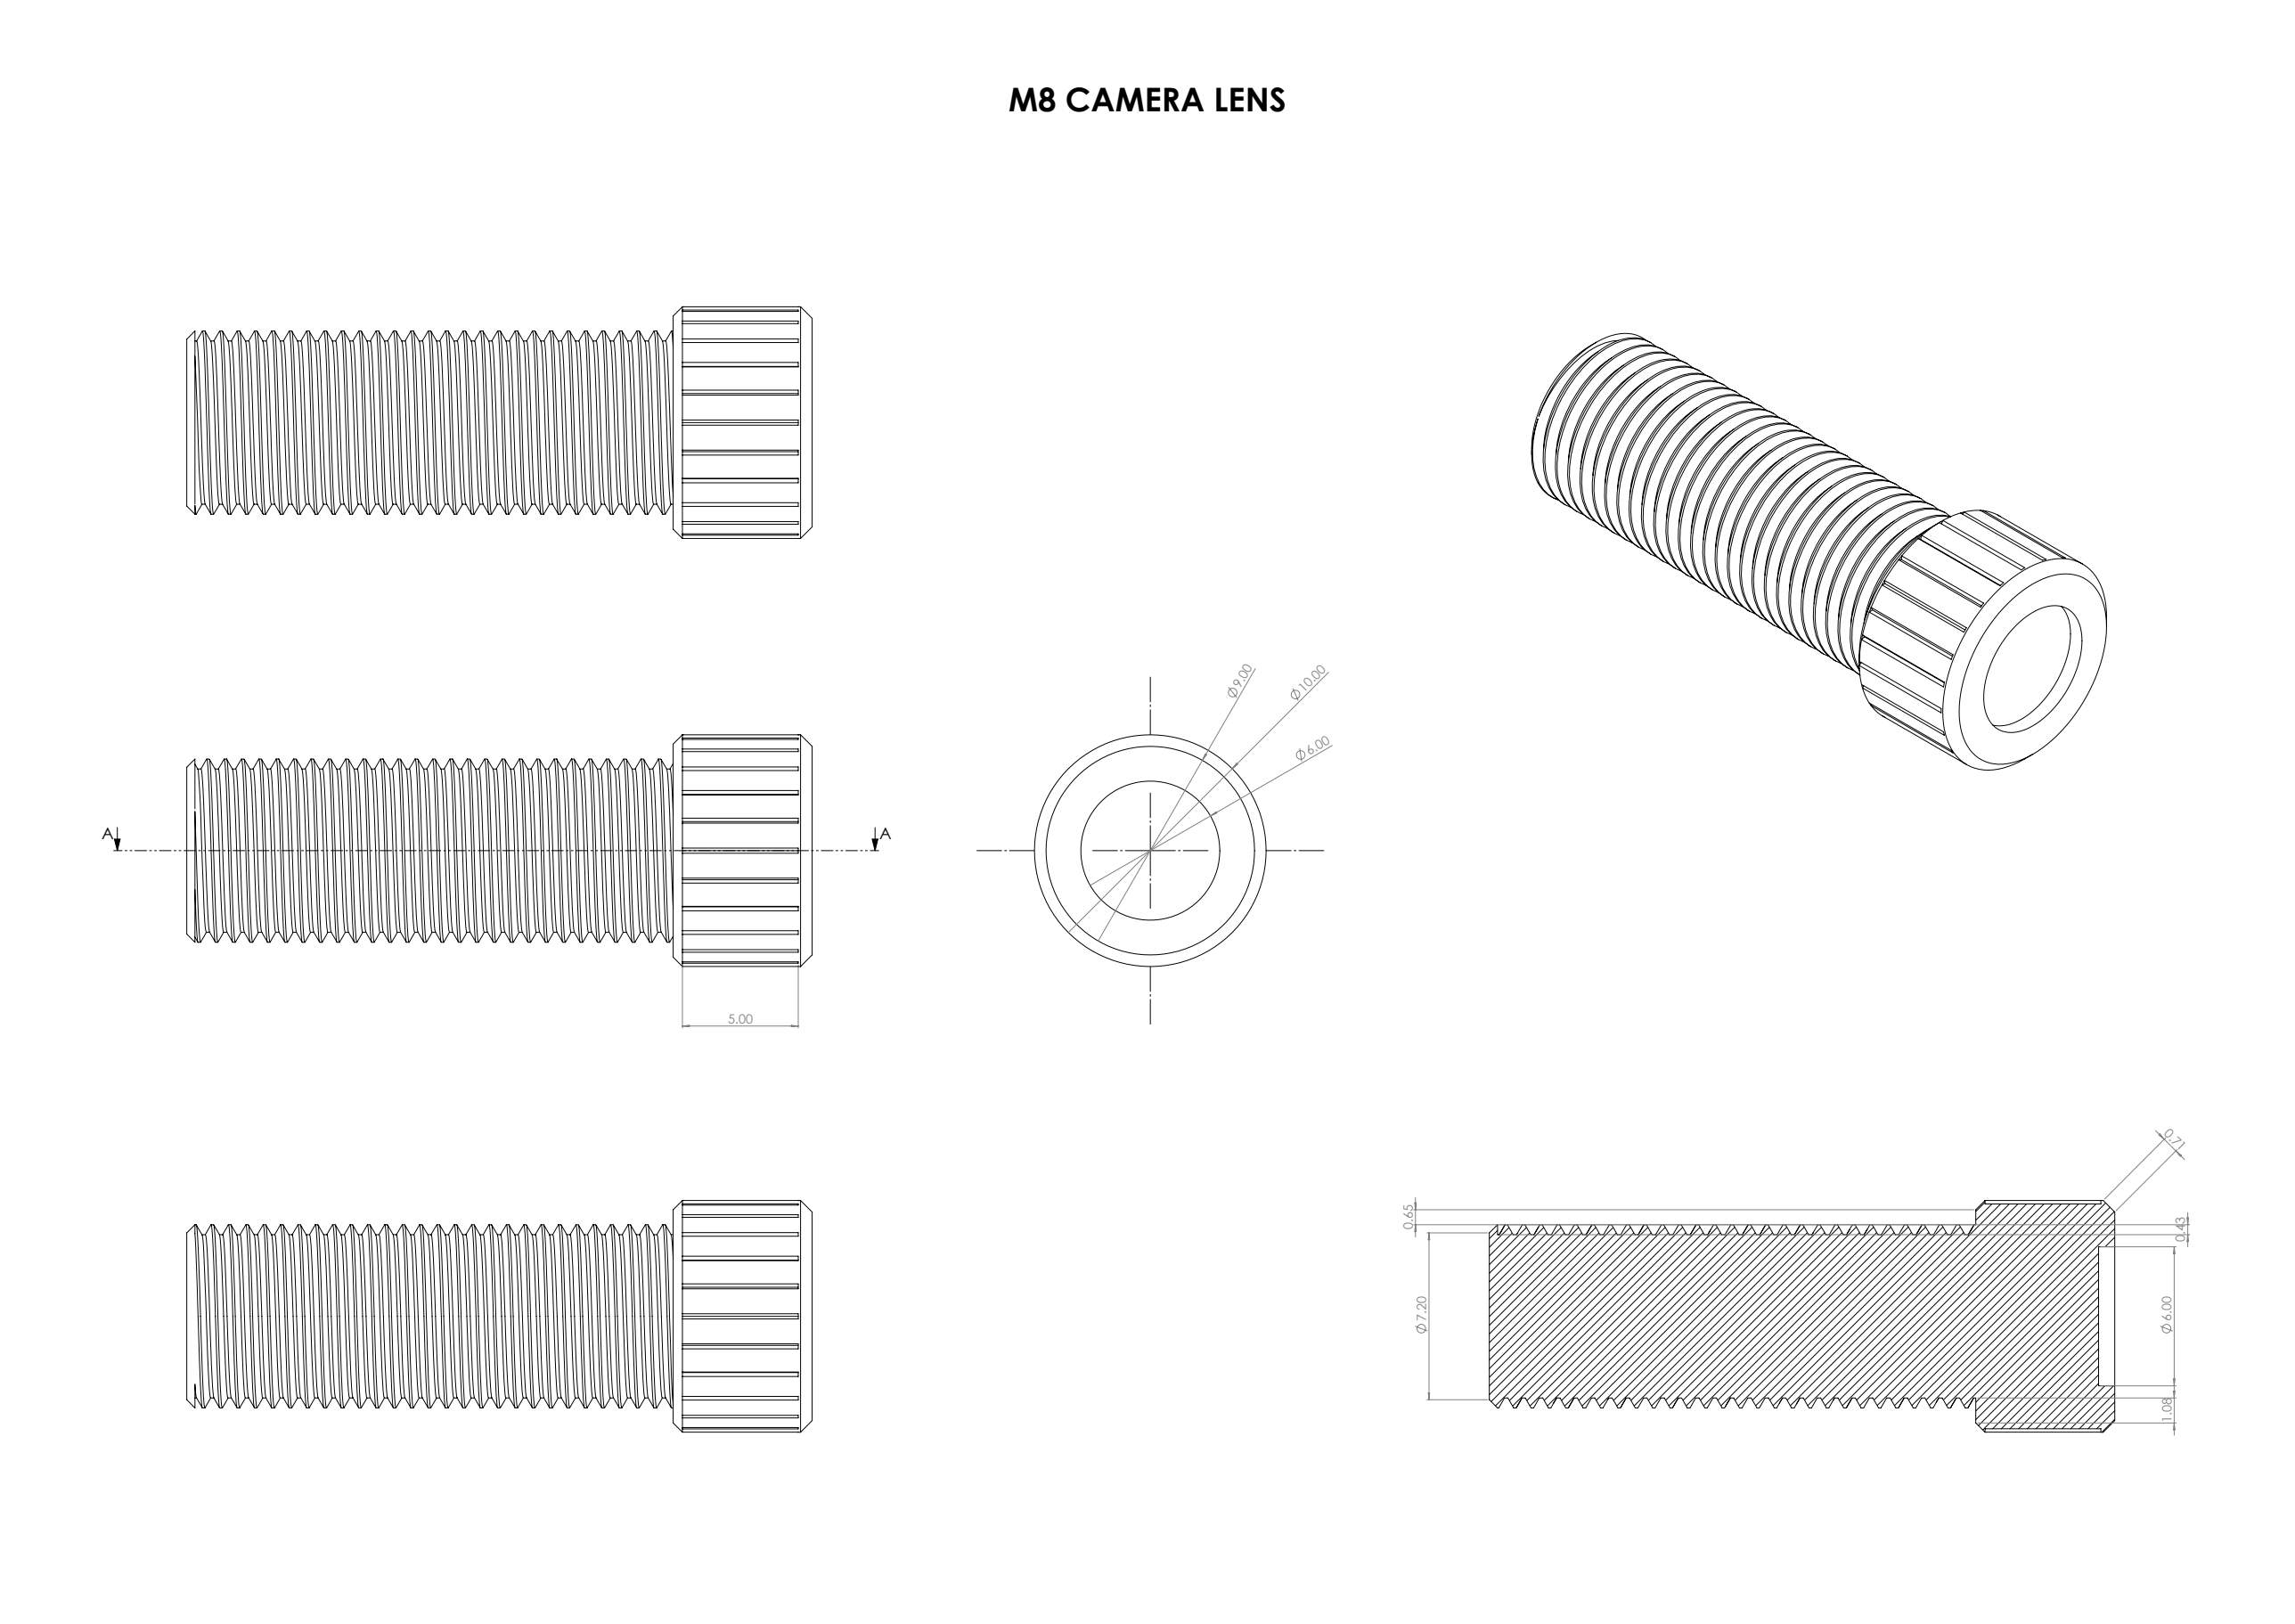
ISO-10303-21;
HEADER;
/* Generated by software containing ST-Developer
 * from STEP Tools, Inc. (www.steptools.com) 
 */

FILE_DESCRIPTION(
/* description */ (''),
/* implementation_level */ '2;1');

FILE_NAME(
/* name */ '07_M8_Camera_Lens.step',
/* time_stamp */ '2026-10-21T02:01:14-07:00',
/* author */ (''),
/* organization */ (''),
/* preprocessor_version */ 'ST-DEVELOPER v20.2',
/* originating_system */ 'Autodesk Translation Framework v15.15.0.0',
/* authorisation */ '');

FILE_SCHEMA (('AUTOMOTIVE_DESIGN { 1 0 10303 214 3 1 1 }'));
ENDSEC;

DATA;
#10=MECHANICAL_DESIGN_GEOMETRIC_PRESENTATION_REPRESENTATION('',(#620),#37181);
#111=B_SPLINE_SURFACE_WITH_KNOTS('',3,3,((#24257,#24258,#24259,#24260,#24261,
#24262,#24263,#24264,#24265,#24266,#24267,#24268,#24269,#24270,#24271,#24272,
#24273,#24274,#24275,#24276,#24277,#24278,#24279,#24280,#24281,#24282,#24283,
#24284,#24285,#24286,#24287,#24288,#24289,#24290,#24291,#24292,#24293,#24294,
#24295,#24296,#24297,#24298,#24299,#24300,#24301,#24302,#24303,#24304,#24305,
#24306,#24307,#24308,#24309,#24310,#24311,#24312,#24313,#24314,#24315,#24316,
#24317,#24318,#24319,#24320,#24321,#24322,#24323,#24324,#24325,#24326,#24327,
#24328,#24329,#24330,#24331,#24332,#24333,#24334,#24335,#24336,#24337,#24338,
#24339,#24340,#24341,#24342,#24343,#24344,#24345,#24346,#24347,#24348,#24349,
#24350,#24351,#24352,#24353,#24354,#24355,#24356,#24357,#24358,#24359,#24360,
#24361,#24362,#24363,#24364,#24365,#24366,#24367,#24368,#24369,#24370,#24371,
#24372,#24373,#24374,#24375,#24376,#24377,#24378,#24379,#24380,#24381,#24382,
#24383,#24384,#24385,#24386,#24387,#24388,#24389,#24390,#24391,#24392,#24393,
#24394,#24395,#24396,#24397,#24398,#24399,#24400,#24401,#24402,#24403,#24404,
#24405,#24406,#24407,#24408,#24409,#24410,#24411,#24412,#24413,#24414,#24415,
#24416,#24417,#24418,#24419,#24420,#24421,#24422,#24423,#24424,#24425,#24426,
#24427,#24428,#24429,#24430,#24431,#24432,#24433,#24434,#24435),(#24436,
#24437,#24438,#24439,#24440,#24441,#24442,#24443,#24444,#24445,#24446,#24447,
#24448,#24449,#24450,#24451,#24452,#24453,#24454,#24455,#24456,#24457,#24458,
#24459,#24460,#24461,#24462,#24463,#24464,#24465,#24466,#24467,#24468,#24469,
#24470,#24471,#24472,#24473,#24474,#24475,#24476,#24477,#24478,#24479,#24480,
#24481,#24482,#24483,#24484,#24485,#24486,#24487,#24488,#24489,#24490,#24491,
#24492,#24493,#24494,#24495,#24496,#24497,#24498,#24499,#24500,#24501,#24502,
#24503,#24504,#24505,#24506,#24507,#24508,#24509,#24510,#24511,#24512,#24513,
#24514,#24515,#24516,#24517,#24518,#24519,#24520,#24521,#24522,#24523,#24524,
#24525,#24526,#24527,#24528,#24529,#24530,#24531,#24532,#24533,#24534,#24535,
#24536,#24537,#24538,#24539,#24540,#24541,#24542,#24543,#24544,#24545,#24546,
#24547,#24548,#24549,#24550,#24551,#24552,#24553,#24554,#24555,#24556,#24557,
#24558,#24559,#24560,#24561,#24562,#24563,#24564,#24565,#24566,#24567,#24568,
#24569,#24570,#24571,#24572,#24573,#24574,#24575,#24576,#24577,#24578,#24579,
#24580,#24581,#24582,#24583,#24584,#24585,#24586,#24587,#24588,#24589,#24590,
#24591,#24592,#24593,#24594,#24595,#24596,#24597,#24598,#24599,#24600,#24601,
#24602,#24603,#24604,#24605,#24606,#24607,#24608,#24609,#24610,#24611,#24612,
#24613,#24614),(#24615,#24616,#24617,#24618,#24619,#24620,#24621,#24622,
#24623,#24624,#24625,#24626,#24627,#24628,#24629,#24630,#24631,#24632,#24633,
#24634,#24635,#24636,#24637,#24638,#24639,#24640,#24641,#24642,#24643,#24644,
#24645,#24646,#24647,#24648,#24649,#24650,#24651,#24652,#24653,#24654,#24655,
#24656,#24657,#24658,#24659,#24660,#24661,#24662,#24663,#24664,#24665,#24666,
#24667,#24668,#24669,#24670,#24671,#24672,#24673,#24674,#24675,#24676,#24677,
#24678,#24679,#24680,#24681,#24682,#24683,#24684,#24685,#24686,#24687,#24688,
#24689,#24690,#24691,#24692,#24693,#24694,#24695,#24696,#24697,#24698,#24699,
#24700,#24701,#24702,#24703,#24704,#24705,#24706,#24707,#24708,#24709,#24710,
#24711,#24712,#24713,#24714,#24715,#24716,#24717,#24718,#24719,#24720,#24721,
#24722,#24723,#24724,#24725,#24726,#24727,#24728,#24729,#24730,#24731,#24732,
#24733,#24734,#24735,#24736,#24737,#24738,#24739,#24740,#24741,#24742,#24743,
#24744,#24745,#24746,#24747,#24748,#24749,#24750,#24751,#24752,#24753,#24754,
#24755,#24756,#24757,#24758,#24759,#24760,#24761,#24762,#24763,#24764,#24765,
#24766,#24767,#24768,#24769,#24770,#24771,#24772,#24773,#24774,#24775,#24776,
#24777,#24778,#24779,#24780,#24781,#24782,#24783,#24784,#24785,#24786,#24787,
#24788,#24789,#24790,#24791,#24792,#24793),(#24794,#24795,#24796,#24797,
#24798,#24799,#24800,#24801,#24802,#24803,#24804,#24805,#24806,#24807,#24808,
#24809,#24810,#24811,#24812,#24813,#24814,#24815,#24816,#24817,#24818,#24819,
#24820,#24821,#24822,#24823,#24824,#24825,#24826,#24827,#24828,#24829,#24830,
#24831,#24832,#24833,#24834,#24835,#24836,#24837,#24838,#24839,#24840,#24841,
#24842,#24843,#24844,#24845,#24846,#24847,#24848,#24849,#24850,#24851,#24852,
#24853,#24854,#24855,#24856,#24857,#24858,#24859,#24860,#24861,#24862,#24863,
#24864,#24865,#24866,#24867,#24868,#24869,#24870,#24871,#24872,#24873,#24874,
#24875,#24876,#24877,#24878,#24879,#24880,#24881,#24882,#24883,#24884,#24885,
#24886,#24887,#24888,#24889,#24890,#24891,#24892,#24893,#24894,#24895,#24896,
#24897,#24898,#24899,#24900,#24901,#24902,#24903,#24904,#24905,#24906,#24907,
#24908,#24909,#24910,#24911,#24912,#24913,#24914,#24915,#24916,#24917,#24918,
#24919,#24920,#24921,#24922,#24923,#24924,#24925,#24926,#24927,#24928,#24929,
#24930,#24931,#24932,#24933,#24934,#24935,#24936,#24937,#24938,#24939,#24940,
#24941,#24942,#24943,#24944,#24945,#24946,#24947,#24948,#24949,#24950,#24951,
#24952,#24953,#24954,#24955,#24956,#24957,#24958,#24959,#24960,#24961,#24962,
#24963,#24964,#24965,#24966,#24967,#24968,#24969,#24970,#24971,#24972)),
 .UNSPECIFIED.,.F.,.F.,.F.,(4,4),(4,1,1,1,1,1,1,1,1,1,1,1,1,1,1,1,1,1,1,
1,1,1,1,1,1,1,1,1,1,1,1,1,1,1,1,1,1,1,1,1,1,1,1,1,1,1,1,1,1,1,1,1,1,1,1,
1,1,1,1,1,1,1,1,1,1,1,1,1,1,1,1,1,1,1,1,1,1,1,1,1,1,1,1,1,1,1,1,1,1,1,1,
1,1,1,1,1,1,1,1,1,1,1,1,1,1,1,1,1,1,1,1,1,1,1,1,1,1,1,1,1,1,1,1,1,1,1,1,
1,1,1,1,1,1,1,1,1,1,1,1,1,1,1,1,1,1,1,1,1,1,1,1,1,1,1,1,1,1,1,1,1,1,1,1,
1,1,1,1,1,1,1,1,1,1,1,1,1,4),(0.,0.0496809906637673),(8.29514371672438,
9.2897150667619,10.2842864167994,11.2788577668369,12.2734291168745,13.268000466912,
14.2625718169495,15.257143166987,16.2517145170246,17.2462858670621,18.2408572170996,
19.2354285671371,20.2299999171747,21.2245712672122,22.2191426172497,23.2137139672872,
24.2082853173248,25.2028566673623,26.1974280173998,27.1919993674374,28.1865707174749,
29.1811420675124,30.1757134175499,31.1702847675875,32.164856117625,33.1594274676625,
34.1539988177,35.1485701677375,36.1431415177751,37.1377128678126,38.1322842178501,
39.1268555678876,40.1214269179252,41.1159982679627,42.1105696180002,43.1051409680378,
44.0997123180753,45.0942836681128,46.0888550181503,47.0834263681879,48.0779977182254,
49.0725690682629,50.0671404183004,51.061711768338,52.0562831183755,53.050854468413,
54.0454258184505,55.039997168488,56.0345685185256,57.0291398685631,58.0237112186006,
59.0182825686381,60.0128539186757,61.0074252687132,62.0019966187507,62.9965679687882,
63.9911393188258,64.9857106688633,65.9802820189008,66.9748533689383,67.9694247189759,
68.9639960690134,69.9585674190509,70.9531387690884,71.947710119126,72.9422814691635,
73.936852819201,74.9314241692385,75.9259955192761,76.9205668693136,77.9151382193511,
78.9097095693886,79.9042809194262,80.8988522694637,81.8934236195012,82.8879949695387,
83.8825663195763,84.8771376696138,85.8717090196513,86.8662803696888,87.8608517197264,
88.8554230697639,89.8499944198014,90.8445657698389,91.8391371198765,92.833708469914,
93.8282798199515,94.822851169989,95.8174225200266,96.8119938700641,97.8065652201016,
98.8011365701391,99.7957079201767,100.790279270214,101.784850620252,102.779421970289,
103.773993320327,104.768564670364,105.763136020402,106.757707370439,107.752278720477,
108.746850070514,109.741421420552,110.735992770589,111.730564120627,112.725135470664,
113.719706820702,114.71427817074,115.708849520777,116.703420870815,117.697992220852,
118.69256357089,119.687134920927,120.681706270965,121.676277621002,122.67084897104,
123.665420321077,124.659991671115,125.654563021152,126.64913437119,127.643705721227,
128.638277071265,129.632848421302,130.62741977134,131.621991121377,132.616562471415,
133.611133821453,134.60570517149,135.600276521528,136.594847871565,137.589419221603,
138.58399057164,139.578561921678,140.573133271715,141.567704621753,142.56227597179,
143.556847321828,144.551418671865,145.545990021903,146.54056137194,147.535132721978,
148.529704072015,149.524275422053,150.51884677209,151.513418122128,152.507989472165,
153.502560822203,154.497132172241,155.491703522278,156.486274872316,157.480846222353,
158.475417572391,159.469988922428,160.464560272466,161.459131622503,162.453702972541,
163.448274322578,164.442845672616,165.437417022653,166.431988372691,167.426559722728,
168.421131072766,169.415702422803,170.410273772841,171.404845122878,172.399416472916,
173.393987822954,174.388559172991,175.383130523029,176.377701873066,177.372273223104,
178.366844573141,179.361415923179,180.355987273216,181.350558623254,182.345129973291,
183.339701323329),.UNSPECIFIED.);
#112=B_SPLINE_SURFACE_WITH_KNOTS('',3,3,((#25202,#25203,#25204,#25205,#25206,
#25207,#25208,#25209,#25210,#25211,#25212,#25213,#25214,#25215,#25216,#25217,
#25218,#25219,#25220,#25221,#25222,#25223,#25224,#25225,#25226,#25227,#25228,
#25229,#25230,#25231,#25232,#25233,#25234,#25235,#25236,#25237,#25238,#25239,
#25240,#25241,#25242,#25243,#25244,#25245,#25246,#25247,#25248,#25249,#25250,
#25251,#25252,#25253,#25254,#25255,#25256,#25257,#25258,#25259,#25260,#25261,
#25262,#25263,#25264,#25265,#25266,#25267,#25268,#25269,#25270,#25271,#25272,
#25273,#25274,#25275,#25276,#25277,#25278,#25279,#25280,#25281,#25282,#25283,
#25284,#25285,#25286,#25287,#25288,#25289,#25290,#25291,#25292,#25293,#25294,
#25295,#25296,#25297,#25298,#25299,#25300,#25301,#25302,#25303,#25304,#25305,
#25306,#25307,#25308,#25309,#25310,#25311,#25312,#25313,#25314,#25315,#25316,
#25317,#25318,#25319,#25320,#25321,#25322,#25323,#25324,#25325,#25326,#25327,
#25328,#25329,#25330,#25331,#25332,#25333,#25334,#25335,#25336,#25337,#25338,
#25339,#25340,#25341,#25342,#25343,#25344,#25345,#25346,#25347,#25348,#25349,
#25350,#25351,#25352,#25353,#25354,#25355,#25356,#25357,#25358,#25359,#25360,
#25361,#25362,#25363,#25364,#25365,#25366,#25367,#25368,#25369,#25370,#25371,
#25372,#25373,#25374,#25375,#25376,#25377,#25378,#25379,#25380),(#25381,
#25382,#25383,#25384,#25385,#25386,#25387,#25388,#25389,#25390,#25391,#25392,
#25393,#25394,#25395,#25396,#25397,#25398,#25399,#25400,#25401,#25402,#25403,
#25404,#25405,#25406,#25407,#25408,#25409,#25410,#25411,#25412,#25413,#25414,
#25415,#25416,#25417,#25418,#25419,#25420,#25421,#25422,#25423,#25424,#25425,
#25426,#25427,#25428,#25429,#25430,#25431,#25432,#25433,#25434,#25435,#25436,
#25437,#25438,#25439,#25440,#25441,#25442,#25443,#25444,#25445,#25446,#25447,
#25448,#25449,#25450,#25451,#25452,#25453,#25454,#25455,#25456,#25457,#25458,
#25459,#25460,#25461,#25462,#25463,#25464,#25465,#25466,#25467,#25468,#25469,
#25470,#25471,#25472,#25473,#25474,#25475,#25476,#25477,#25478,#25479,#25480,
#25481,#25482,#25483,#25484,#25485,#25486,#25487,#25488,#25489,#25490,#25491,
#25492,#25493,#25494,#25495,#25496,#25497,#25498,#25499,#25500,#25501,#25502,
#25503,#25504,#25505,#25506,#25507,#25508,#25509,#25510,#25511,#25512,#25513,
#25514,#25515,#25516,#25517,#25518,#25519,#25520,#25521,#25522,#25523,#25524,
#25525,#25526,#25527,#25528,#25529,#25530,#25531,#25532,#25533,#25534,#25535,
#25536,#25537,#25538,#25539,#25540,#25541,#25542,#25543,#25544,#25545,#25546,
#25547,#25548,#25549,#25550,#25551,#25552,#25553,#25554,#25555,#25556,#25557,
#25558,#25559),(#25560,#25561,#25562,#25563,#25564,#25565,#25566,#25567,
#25568,#25569,#25570,#25571,#25572,#25573,#25574,#25575,#25576,#25577,#25578,
#25579,#25580,#25581,#25582,#25583,#25584,#25585,#25586,#25587,#25588,#25589,
#25590,#25591,#25592,#25593,#25594,#25595,#25596,#25597,#25598,#25599,#25600,
#25601,#25602,#25603,#25604,#25605,#25606,#25607,#25608,#25609,#25610,#25611,
#25612,#25613,#25614,#25615,#25616,#25617,#25618,#25619,#25620,#25621,#25622,
#25623,#25624,#25625,#25626,#25627,#25628,#25629,#25630,#25631,#25632,#25633,
#25634,#25635,#25636,#25637,#25638,#25639,#25640,#25641,#25642,#25643,#25644,
#25645,#25646,#25647,#25648,#25649,#25650,#25651,#25652,#25653,#25654,#25655,
#25656,#25657,#25658,#25659,#25660,#25661,#25662,#25663,#25664,#25665,#25666,
#25667,#25668,#25669,#25670,#25671,#25672,#25673,#25674,#25675,#25676,#25677,
#25678,#25679,#25680,#25681,#25682,#25683,#25684,#25685,#25686,#25687,#25688,
#25689,#25690,#25691,#25692,#25693,#25694,#25695,#25696,#25697,#25698,#25699,
#25700,#25701,#25702,#25703,#25704,#25705,#25706,#25707,#25708,#25709,#25710,
#25711,#25712,#25713,#25714,#25715,#25716,#25717,#25718,#25719,#25720,#25721,
#25722,#25723,#25724,#25725,#25726,#25727,#25728,#25729,#25730,#25731,#25732,
#25733,#25734,#25735,#25736,#25737,#25738),(#25739,#25740,#25741,#25742,
#25743,#25744,#25745,#25746,#25747,#25748,#25749,#25750,#25751,#25752,#25753,
#25754,#25755,#25756,#25757,#25758,#25759,#25760,#25761,#25762,#25763,#25764,
#25765,#25766,#25767,#25768,#25769,#25770,#25771,#25772,#25773,#25774,#25775,
#25776,#25777,#25778,#25779,#25780,#25781,#25782,#25783,#25784,#25785,#25786,
#25787,#25788,#25789,#25790,#25791,#25792,#25793,#25794,#25795,#25796,#25797,
#25798,#25799,#25800,#25801,#25802,#25803,#25804,#25805,#25806,#25807,#25808,
#25809,#25810,#25811,#25812,#25813,#25814,#25815,#25816,#25817,#25818,#25819,
#25820,#25821,#25822,#25823,#25824,#25825,#25826,#25827,#25828,#25829,#25830,
#25831,#25832,#25833,#25834,#25835,#25836,#25837,#25838,#25839,#25840,#25841,
#25842,#25843,#25844,#25845,#25846,#25847,#25848,#25849,#25850,#25851,#25852,
#25853,#25854,#25855,#25856,#25857,#25858,#25859,#25860,#25861,#25862,#25863,
#25864,#25865,#25866,#25867,#25868,#25869,#25870,#25871,#25872,#25873,#25874,
#25875,#25876,#25877,#25878,#25879,#25880,#25881,#25882,#25883,#25884,#25885,
#25886,#25887,#25888,#25889,#25890,#25891,#25892,#25893,#25894,#25895,#25896,
#25897,#25898,#25899,#25900,#25901,#25902,#25903,#25904,#25905,#25906,#25907,
#25908,#25909,#25910,#25911,#25912,#25913,#25914,#25915,#25916,#25917)),
 .UNSPECIFIED.,.F.,.F.,.F.,(4,4),(4,1,1,1,1,1,1,1,1,1,1,1,1,1,1,1,1,1,1,
1,1,1,1,1,1,1,1,1,1,1,1,1,1,1,1,1,1,1,1,1,1,1,1,1,1,1,1,1,1,1,1,1,1,1,1,
1,1,1,1,1,1,1,1,1,1,1,1,1,1,1,1,1,1,1,1,1,1,1,1,1,1,1,1,1,1,1,1,1,1,1,1,
1,1,1,1,1,1,1,1,1,1,1,1,1,1,1,1,1,1,1,1,1,1,1,1,1,1,1,1,1,1,1,1,1,1,1,1,
1,1,1,1,1,1,1,1,1,1,1,1,1,1,1,1,1,1,1,1,1,1,1,1,1,1,1,1,1,1,1,1,1,1,1,1,
1,1,1,1,1,1,1,1,1,1,1,1,1,4),(0.,0.0496809906637673),(11.6149723878396,
12.6095437378771,13.6041150879146,14.5986864379522,15.5932577879897,16.5878291380272,
17.5824004880647,18.5769718381023,19.5715431881398,20.5661145381773,21.5606858882148,
22.5552572382524,23.5498285882899,24.5443999383274,25.5389712883649,26.5335426384025,
27.52811398844,28.5226853384775,29.517256688515,30.5118280385526,31.5063993885901,
32.5009707386276,33.4955420886651,34.4901134387027,35.4846847887402,36.4792561387777,
37.4738274888152,38.4683988388528,39.4629701888903,40.4575415389278,41.4521128889653,
42.4466842390029,43.4412555890404,44.4358269390779,45.4303982891154,46.424969639153,
47.4195409891905,48.414112339228,49.4086836892655,50.4032550393031,51.3978263893406,
52.3923977393781,53.3869690894156,54.3815404394532,55.3761117894907,56.3706831395282,
57.3652544895657,58.3598258396033,59.3543971896408,60.3489685396783,61.3435398897158,
62.3381112397534,63.3326825897909,64.3272539398284,65.3218252898659,66.3163966399035,
67.310967989941,68.3055393399785,69.300110690016,70.2946820400536,71.2892533900911,
72.2838247401286,73.2783960901661,74.2729674402037,75.2675387902412,76.2621101402787,
77.2566814903162,78.2512528403538,79.2458241903913,80.2403955404288,81.2349668904663,
82.2295382405039,83.2241095905414,84.2186809405789,85.2132522906164,86.207823640654,
87.2023949906915,88.196966340729,89.1915376907665,90.1861090408041,91.1806803908416,
92.1752517408791,93.1698230909166,94.1643944409542,95.1589657909917,96.1535371410292,
97.1481084910667,98.1426798411043,99.1372511911418,100.131822541179,101.126393891217,
102.120965241254,103.115536591292,104.110107941329,105.104679291367,106.099250641404,
107.093821991442,108.08839334148,109.082964691517,110.077536041555,111.072107391592,
112.06667874163,113.061250091667,114.055821441705,115.050392791742,116.04496414178,
117.039535491817,118.034106841855,119.028678191892,120.02324954193,121.017820891967,
122.012392242005,123.006963592042,124.00153494208,124.996106292117,125.990677642155,
126.985248992192,127.97982034223,128.974391692268,129.968963042305,130.963534392343,
131.95810574238,132.952677092418,133.947248442455,134.941819792493,135.93639114253,
136.930962492568,137.925533842605,138.920105192643,139.91467654268,140.909247892718,
141.903819242755,142.898390592793,143.89296194283,144.887533292868,145.882104642905,
146.876675992943,147.87124734298,148.865818693018,149.860390043056,150.854961393093,
151.849532743131,152.844104093168,153.838675443206,154.833246793243,155.827818143281,
156.822389493318,157.816960843356,158.811532193393,159.806103543431,160.800674893468,
161.795246243506,162.789817593543,163.784388943581,164.778960293618,165.773531643656,
166.768102993693,167.762674343731,168.757245693769,169.751817043806,170.746388393844,
171.740959743881,172.735531093919,173.730102443956,174.724673793994,175.719245144031,
176.713816494069,177.708387844106,178.702959194144,179.697530544181,180.692101894219,
181.686673244256,182.681244594294,183.675815944331,184.670387294369,185.664958644406,
186.659529994444),.UNSPECIFIED.);
#141=B_SPLINE_CURVE_WITH_KNOTS('',3,(#21804,#21805,#21806,#21807,#21808,
#21809,#21810,#21811,#21812,#21813),.UNSPECIFIED.,.F.,.F.,(4,3,3,4),(-4.09299088010945,
-3.9782854001501,-2.98371405011257,-2.08103247056473),.UNSPECIFIED.);
#142=B_SPLINE_CURVE_WITH_KNOTS('',3,(#21816,#21817,#21818,#21819,#21820,
#21821,#21822),.UNSPECIFIED.,.F.,.F.,(4,3,4),(0.,0.994571350037526,1.12963424404512),
 .UNSPECIFIED.);
#143=B_SPLINE_CURVE_WITH_KNOTS('',3,(#21827,#21828,#21829,#21830,#21831,
#21832,#21833,#21834,#21835,#21836,#21837,#21838,#21839,#21840,#21841,#21842,
#21843,#21844,#21845,#21846,#21847,#21848),.UNSPECIFIED.,.F.,.F.,(4,3,3,
3,3,3,3,4),(-10.376176187289,-9.94571350037525,-8.95114215033773,-7.9565708003002,
-6.96199945026268,-5.96742810022515,-4.97285675018763,-4.09299088010945),
 .UNSPECIFIED.);
#144=B_SPLINE_CURVE_WITH_KNOTS('',3,(#21849,#21850,#21851,#21852,#21853,
#21854,#21855,#21856,#21857,#21858,#21859,#21860,#21861,#21862,#21863,#21864,
#21865,#21866,#21867,#21868,#21869,#21870),.UNSPECIFIED.,.F.,.F.,(4,3,3,
3,3,3,3,4),(1.12963424404512,1.98914270007505,2.98371405011257,3.9782854001501,
4.97285675018762,5.96742810022515,6.96199945026267,7.4128195512247),
 .UNSPECIFIED.);
#145=B_SPLINE_CURVE_WITH_KNOTS('',3,(#21875,#21876,#21877,#21878,#21879,
#21880,#21881,#21882,#21883,#21884,#21885,#21886,#21887,#21888,#21889,#21890,
#21891,#21892,#21893,#21894,#21895,#21896),.UNSPECIFIED.,.F.,.F.,(4,3,3,
3,3,3,3,4),(-16.6593614944686,-15.9131416006004,-14.9185702505629,-13.9239989005253,
-12.9294275504878,-11.9348562004503,-10.9402848504128,-10.376176187289),
 .UNSPECIFIED.);
#146=B_SPLINE_CURVE_WITH_KNOTS('',3,(#21897,#21898,#21899,#21900,#21901,
#21902,#21903,#21904,#21905,#21906,#21907,#21908,#21909,#21910,#21911,#21912,
#21913,#21914,#21915,#21916,#21917,#21918),.UNSPECIFIED.,.F.,.F.,(4,3,3,
3,3,3,3,4),(7.4128195512247,7.9565708003002,8.95114215033773,9.94571350037526,
10.9402848504128,11.9348562004503,12.9294275504878,13.6960048584043),
 .UNSPECIFIED.);
#147=B_SPLINE_CURVE_WITH_KNOTS('',3,(#21923,#21924,#21925,#21926,#21927,
#21928,#21929,#21930,#21931,#21932,#21933,#21934,#21935,#21936,#21937,#21938,
#21939,#21940,#21941,#21942,#21943,#21944,#21945,#21946,#21947),
 .UNSPECIFIED.,.F.,.F.,(4,3,3,3,3,3,3,3,4),(-22.9425468016482,-22.8751410508631,
-21.8805697008255,-20.885998350788,-19.8914270007505,-18.896855650713,-17.9022843006754,
-16.9077129506379,-16.6593614944686),.UNSPECIFIED.);
#148=B_SPLINE_CURVE_WITH_KNOTS('',3,(#21948,#21949,#21950,#21951,#21952,
#21953,#21954,#21955,#21956,#21957,#21958,#21959,#21960,#21961,#21962,#21963,
#21964,#21965,#21966,#21967,#21968,#21969,#21970,#21971,#21972),
 .UNSPECIFIED.,.F.,.F.,(4,3,3,3,3,3,3,3,4),(13.6960048584043,13.9239989005254,
14.9185702505629,15.9131416006004,16.9077129506379,17.9022843006755,18.896855650713,
19.8914270007505,19.9791901655839),.UNSPECIFIED.);
#149=B_SPLINE_CURVE_WITH_KNOTS('',3,(#21977,#21978,#21979,#21980,#21981,
#21982,#21983,#21984,#21985,#21986,#21987,#21988,#21989,#21990,#21991,#21992,
#21993,#21994,#21995,#21996,#21997,#21998),.UNSPECIFIED.,.F.,.F.,(4,3,3,
3,3,3,3,4),(-29.2257321088278,-28.8425691510882,-27.8479978010507,-26.8534264510132,
-25.8588551009757,-24.8642837509381,-23.8697124009006,-22.9425468016482),
 .UNSPECIFIED.);
#150=B_SPLINE_CURVE_WITH_KNOTS('',3,(#21999,#22000,#22001,#22002,#22003,
#22004,#22005,#22006,#22007,#22008,#22009,#22010,#22011,#22012,#22013,#22014,
#22015,#22016,#22017,#22018,#22019,#22020),.UNSPECIFIED.,.F.,.F.,(4,3,3,
3,3,3,3,4),(19.9791901655839,20.885998350788,21.8805697008255,22.8751410508631,
23.8697124009006,24.8642837509381,25.8588551009756,26.2623754727635),
 .UNSPECIFIED.);
#151=B_SPLINE_CURVE_WITH_KNOTS('',3,(#22025,#22026,#22027,#22028,#22029,
#22030,#22031,#22032,#22033,#22034,#22035,#22036,#22037,#22038,#22039,#22040,
#22041,#22042,#22043,#22044,#22045,#22046),.UNSPECIFIED.,.F.,.F.,(4,3,3,
3,3,3,3,4),(-35.5089174160074,-34.8099972513134,-33.8154259012759,-32.8208545512383,
-31.8262832012008,-30.8317118511633,-29.8371405011258,-29.2257321088278),
 .UNSPECIFIED.);
#152=B_SPLINE_CURVE_WITH_KNOTS('',3,(#22047,#22048,#22049,#22050,#22051,
#22052,#22053,#22054,#22055,#22056,#22057,#22058,#22059,#22060,#22061,#22062,
#22063,#22064,#22065,#22066,#22067,#22068),.UNSPECIFIED.,.F.,.F.,(4,3,3,
3,3,3,3,4),(26.2623754727635,26.8534264510132,27.8479978010507,28.8425691510882,
29.8371405011258,30.8317118511633,31.8262832012008,32.545560779943),
 .UNSPECIFIED.);
#153=B_SPLINE_CURVE_WITH_KNOTS('',3,(#22073,#22074,#22075,#22076,#22077,
#22078,#22079,#22080,#22081,#22082,#22083,#22084,#22085,#22086,#22087,#22088,
#22089,#22090,#22091,#22092,#22093,#22094,#22095,#22096,#22097),
 .UNSPECIFIED.,.F.,.F.,(4,3,3,3,3,3,3,3,4),(-41.792102723187,-41.771996701576,
-40.7774253515385,-39.782854001501,-38.7882826514635,-37.7937113014259,
-36.7991399513884,-35.8045686013509,-35.5089174160074),.UNSPECIFIED.);
#154=B_SPLINE_CURVE_WITH_KNOTS('',3,(#22098,#22099,#22100,#22101,#22102,
#22103,#22104,#22105,#22106,#22107,#22108,#22109,#22110,#22111,#22112,#22113,
#22114,#22115,#22116,#22117,#22118,#22119,#22120,#22121,#22122),
 .UNSPECIFIED.,.F.,.F.,(4,3,3,3,3,3,3,3,4),(32.545560779943,32.8208545512383,
33.8154259012759,34.8099972513134,35.8045686013509,36.7991399513884,37.7937113014259,
38.7882826514634,38.8287460871226),.UNSPECIFIED.);
#155=B_SPLINE_CURVE_WITH_KNOTS('',3,(#22127,#22128,#22129,#22130,#22131,
#22132,#22133,#22134,#22135,#22136,#22137,#22138,#22139,#22140,#22141,#22142,
#22143,#22144,#22145,#22146,#22147,#22148),.UNSPECIFIED.,.F.,.F.,(4,3,3,
3,3,3,3,4),(-48.0752880303666,-47.7394248018012,-46.7448534517637,-45.7502821017261,
-44.7557107516886,-43.7611394016511,-42.7665680516136,-41.792102723187),
 .UNSPECIFIED.);
#156=B_SPLINE_CURVE_WITH_KNOTS('',3,(#22149,#22150,#22151,#22152,#22153,
#22154,#22155,#22156,#22157,#22158,#22159,#22160,#22161,#22162,#22163,#22164,
#22165,#22166,#22167,#22168,#22169,#22170),.UNSPECIFIED.,.F.,.F.,(4,3,3,
3,3,3,3,4),(38.8287460871226,39.782854001501,40.7774253515385,41.771996701576,
42.7665680516136,43.7611394016511,44.7557107516886,45.1119313943022),
 .UNSPECIFIED.);
#157=B_SPLINE_CURVE_WITH_KNOTS('',3,(#22175,#22176,#22177,#22178,#22179,
#22180,#22181,#22182,#22183,#22184,#22185,#22186,#22187,#22188,#22189,#22190,
#22191,#22192,#22193,#22194,#22195,#22196),.UNSPECIFIED.,.F.,.F.,(4,3,3,
3,3,3,3,4),(-54.3584733375462,-53.7068529020263,-52.7122815519888,-51.7177102019513,
-50.7231388519138,-49.7285675018762,-48.7339961518387,-48.0752880303666),
 .UNSPECIFIED.);
#158=B_SPLINE_CURVE_WITH_KNOTS('',3,(#22197,#22198,#22199,#22200,#22201,
#22202,#22203,#22204,#22205,#22206,#22207,#22208,#22209,#22210,#22211,#22212,
#22213,#22214,#22215,#22216,#22217,#22218),.UNSPECIFIED.,.F.,.F.,(4,3,3,
3,3,3,3,4),(45.1119313943022,45.7502821017262,46.7448534517637,47.7394248018012,
48.7339961518387,49.7285675018763,50.7231388519138,51.3951167014818),
 .UNSPECIFIED.);
#159=B_SPLINE_CURVE_WITH_KNOTS('',3,(#22223,#22224,#22225,#22226,#22227,
#22228,#22229,#22230,#22231,#22232,#22233,#22234,#22235,#22236,#22237,#22238,
#22239,#22240,#22241,#22242,#22243,#22244),.UNSPECIFIED.,.F.,.F.,(4,3,3,
3,3,3,3,4),(-60.6416586447258,-59.6742810022515,-58.679709652214,-57.6851383021764,
-56.6905669521389,-55.6959956021014,-54.7014242520639,-54.3584733375462),
 .UNSPECIFIED.);
#160=B_SPLINE_CURVE_WITH_KNOTS('',3,(#22245,#22246,#22247,#22248,#22249,
#22250,#22251,#22252,#22253,#22254,#22255,#22256,#22257,#22258,#22259,#22260,
#22261,#22262,#22263,#22264,#22265,#22266),.UNSPECIFIED.,.F.,.F.,(4,3,3,
3,3,3,3,4),(51.3951167014818,51.7177102019513,52.7122815519888,53.7068529020263,
54.7014242520639,55.6959956021014,56.6905669521389,57.6783020086614),
 .UNSPECIFIED.);
#161=B_SPLINE_CURVE_WITH_KNOTS('',3,(#22271,#22272,#22273,#22274,#22275,
#22276,#22277,#22278,#22279,#22280,#22281,#22282,#22283,#22284,#22285,#22286,
#22287,#22288,#22289,#22290,#22291,#22292,#22293,#22294,#22295),
 .UNSPECIFIED.,.F.,.F.,(4,3,3,3,3,3,3,3,4),(-66.9248439519054,-66.6362804525142,
-65.6417091024766,-64.6471377524391,-63.6525664024016,-62.6579950523641,
-61.6634237023265,-60.668852352289,-60.6416586447258),.UNSPECIFIED.);
#162=B_SPLINE_CURVE_WITH_KNOTS('',3,(#22296,#22297,#22298,#22299,#22300,
#22301,#22302,#22303,#22304,#22305,#22306,#22307,#22308,#22309,#22310,#22311,
#22312,#22313,#22314,#22315,#22316,#22317,#22318,#22319,#22320),
 .UNSPECIFIED.,.F.,.F.,(4,3,3,3,3,3,3,3,4),(57.6783020086614,57.6851383021765,
58.679709652214,59.6742810022515,60.668852352289,61.6634237023265,62.6579950523641,
63.6525664024016,63.961487315841),.UNSPECIFIED.);
#163=B_SPLINE_CURVE_WITH_KNOTS('',3,(#22325,#22326,#22327,#22328,#22329,
#22330,#22331,#22332,#22333,#22334,#22335,#22336,#22337,#22338,#22339,#22340,
#22341,#22342,#22343,#22344,#22345,#22346),.UNSPECIFIED.,.F.,.F.,(4,3,3,
3,3,3,3,4),(-73.2080292590849,-72.6037085527393,-71.6091372027018,-70.6145658526643,
-69.6199945026267,-68.6254231525892,-67.6308518025517,-66.9248439519054),
 .UNSPECIFIED.);
#164=B_SPLINE_CURVE_WITH_KNOTS('',3,(#22347,#22348,#22349,#22350,#22351,
#22352,#22353,#22354,#22355,#22356,#22357,#22358,#22359,#22360,#22361,#22362,
#22363,#22364,#22365,#22366,#22367,#22368),.UNSPECIFIED.,.F.,.F.,(4,3,3,
3,3,3,3,4),(63.961487315841,64.6471377524391,65.6417091024766,66.6362804525142,
67.6308518025517,68.6254231525892,69.6199945026268,70.2446726230206),
 .UNSPECIFIED.);
#165=B_SPLINE_CURVE_WITH_KNOTS('',3,(#22373,#22374,#22375,#22376,#22377,
#22378,#22379,#22380,#22381,#22382,#22383,#22384,#22385,#22386,#22387,#22388,
#22389,#22390,#22391,#22392,#22393,#22394),.UNSPECIFIED.,.F.,.F.,(4,3,3,
3,3,3,3,4),(-79.4912145662645,-78.5711366529645,-77.5765653029269,-76.5819939528894,
-75.5874226028519,-74.5928512528144,-73.5982799027768,-73.2080292590849),
 .UNSPECIFIED.);
#166=B_SPLINE_CURVE_WITH_KNOTS('',3,(#22395,#22396,#22397,#22398,#22399,
#22400,#22401,#22402,#22403,#22404,#22405,#22406,#22407,#22408,#22409,#22410,
#22411,#22412,#22413,#22414,#22415,#22416),.UNSPECIFIED.,.F.,.F.,(4,3,3,
3,3,3,3,4),(70.2446726230206,70.6145658526643,71.6091372027018,72.6037085527393,
73.5982799027769,74.5928512528144,75.5874226028519,76.5278579302002),
 .UNSPECIFIED.);
#167=B_SPLINE_CURVE_WITH_KNOTS('',3,(#22421,#22422,#22423,#22424,#22425,
#22426,#22427,#22428,#22429,#22430,#22431,#22432,#22433,#22434,#22435,#22436,
#22437,#22438,#22439,#22440,#22441,#22442,#22443,#22444,#22445),
 .UNSPECIFIED.,.F.,.F.,(4,3,3,3,3,3,3,3,4),(-85.7743998734441,-85.5331361032271,
-84.5385647531896,-83.5439934031521,-82.5494220531146,-81.554850703077,
-80.5602793530395,-79.565708003002,-79.4912145662645),.UNSPECIFIED.);
#168=B_SPLINE_CURVE_WITH_KNOTS('',3,(#22446,#22447,#22448,#22449,#22450,
#22451,#22452,#22453,#22454,#22455,#22456,#22457,#22458,#22459,#22460,#22461,
#22462,#22463,#22464,#22465,#22466,#22467,#22468,#22469,#22470),
 .UNSPECIFIED.,.F.,.F.,(4,3,3,3,3,3,3,3,4),(76.5278579302002,76.5819939528894,
77.576565302927,78.5711366529645,79.565708003002,80.5602793530395,81.5548507030771,
82.5494220531146,82.8110432373798),.UNSPECIFIED.);
#169=B_SPLINE_CURVE_WITH_KNOTS('',3,(#22475,#22476,#22477,#22478,#22479,
#22480,#22481,#22482,#22483,#22484,#22485,#22486,#22487,#22488,#22489,#22490,
#22491,#22492,#22493,#22494,#22495,#22496),.UNSPECIFIED.,.F.,.F.,(4,3,3,
3,3,3,3,4),(-92.0575851806237,-91.5005642034523,-90.5059928534148,-89.5114215033772,
-88.5168501533397,-87.5222788033022,-86.5277074532647,-85.7743998734441),
 .UNSPECIFIED.);
#170=B_SPLINE_CURVE_WITH_KNOTS('',3,(#22497,#22498,#22499,#22500,#22501,
#22502,#22503,#22504,#22505,#22506,#22507,#22508,#22509,#22510,#22511,#22512,
#22513,#22514,#22515,#22516,#22517,#22518),.UNSPECIFIED.,.F.,.F.,(4,3,3,
3,3,3,3,4),(82.8110432373798,83.5439934031521,84.5385647531896,85.5331361032272,
86.5277074532647,87.5222788033022,88.5168501533397,89.0942285445594),
 .UNSPECIFIED.);
#171=B_SPLINE_CURVE_WITH_KNOTS('',3,(#22523,#22524,#22525,#22526,#22527,
#22528,#22529,#22530,#22531,#22532,#22533,#22534,#22535,#22536,#22537,#22538,
#22539,#22540,#22541,#22542,#22543,#22544),.UNSPECIFIED.,.F.,.F.,(4,3,3,
3,3,3,3,4),(-98.3407704878033,-97.4679923036774,-96.4734209536399,-95.4788496036024,
-94.4842782535649,-93.4897069035273,-92.4951355534898,-92.0575851806237),
 .UNSPECIFIED.);
#172=B_SPLINE_CURVE_WITH_KNOTS('',3,(#22545,#22546,#22547,#22548,#22549,
#22550,#22551,#22552,#22553,#22554,#22555,#22556,#22557,#22558,#22559,#22560,
#22561,#22562,#22563,#22564,#22565,#22566),.UNSPECIFIED.,.F.,.F.,(4,3,3,
3,3,3,3,4),(89.0942285445594,89.5114215033772,90.5059928534148,91.5005642034523,
92.4951355534898,93.4897069035273,94.4842782535649,95.377413851739),
 .UNSPECIFIED.);
#173=B_SPLINE_CURVE_WITH_KNOTS('',3,(#22571,#22572,#22573,#22574,#22575,
#22576,#22577,#22578,#22579,#22580,#22581,#22582,#22583,#22584,#22585,#22586,
#22587,#22588,#22589,#22590,#22591,#22592,#22593,#22594,#22595),
 .UNSPECIFIED.,.F.,.F.,(4,3,3,3,3,3,3,3,4),(-104.623955794983,-104.42999175394,
-103.435420403903,-102.440849053865,-101.446277703828,-100.45170635379,
-99.4571350037525,-98.462563653715,-98.3407704878033),.UNSPECIFIED.);
#174=B_SPLINE_CURVE_WITH_KNOTS('',3,(#22596,#22597,#22598,#22599,#22600,
#22601,#22602,#22603,#22604,#22605,#22606,#22607,#22608,#22609,#22610,#22611,
#22612,#22613,#22614,#22615,#22616,#22617,#22618,#22619,#22620),
 .UNSPECIFIED.,.F.,.F.,(4,3,3,3,3,3,3,3,4),(95.377413851739,95.4788496036024,
96.4734209536399,97.4679923036774,98.462563653715,99.4571350037525,100.45170635379,
101.446277703828,101.660599158919),.UNSPECIFIED.);
#175=B_SPLINE_CURVE_WITH_KNOTS('',3,(#22625,#22626,#22627,#22628,#22629,
#22630,#22631,#22632,#22633,#22634,#22635,#22636,#22637,#22638,#22639,#22640,
#22641,#22642,#22643,#22644,#22645,#22646),.UNSPECIFIED.,.F.,.F.,(4,3,3,
3,3,3,3,4),(-110.907141102163,-110.397419854165,-109.402848504128,-108.40827715409,
-107.413705804053,-106.419134454015,-105.424563103978,-104.623955794983),
 .UNSPECIFIED.);
#176=B_SPLINE_CURVE_WITH_KNOTS('',3,(#22647,#22648,#22649,#22650,#22651,
#22652,#22653,#22654,#22655,#22656,#22657,#22658,#22659,#22660,#22661,#22662,
#22663,#22664,#22665,#22666,#22667,#22668),.UNSPECIFIED.,.F.,.F.,(4,3,3,
3,3,3,3,4),(101.660599158919,102.440849053865,103.435420403903,104.42999175394,
105.424563103978,106.419134454015,107.413705804053,107.943784466098),
 .UNSPECIFIED.);
#177=B_SPLINE_CURVE_WITH_KNOTS('',3,(#22673,#22674,#22675,#22676,#22677,
#22678,#22679,#22680,#22681,#22682,#22683,#22684,#22685,#22686,#22687,#22688,
#22689,#22690,#22691,#22692,#22693,#22694),.UNSPECIFIED.,.F.,.F.,(4,3,3,
3,3,3,3,4),(-117.190326409342,-116.36484795439,-115.370276604353,-114.375705254315,
-113.381133904278,-112.38656255424,-111.391991204203,-110.907141102163),
 .UNSPECIFIED.);
#178=B_SPLINE_CURVE_WITH_KNOTS('',3,(#22695,#22696,#22697,#22698,#22699,
#22700,#22701,#22702,#22703,#22704,#22705,#22706,#22707,#22708,#22709,#22710,
#22711,#22712,#22713,#22714,#22715,#22716),.UNSPECIFIED.,.F.,.F.,(4,3,3,
3,3,3,3,4),(107.943784466098,108.40827715409,109.402848504128,110.397419854165,
111.391991204203,112.38656255424,113.381133904278,114.226969773278),
 .UNSPECIFIED.);
#179=B_SPLINE_CURVE_WITH_KNOTS('',3,(#22721,#22722,#22723,#22724,#22725,
#22726,#22727,#22728,#22729,#22730,#22731,#22732,#22733,#22734,#22735,#22736,
#22737,#22738,#22739,#22740,#22741,#22742,#22743,#22744,#22745),
 .UNSPECIFIED.,.F.,.F.,(4,3,3,3,3,3,3,3,4),(-123.473511716522,-123.326847404653,
-122.332276054616,-121.337704704578,-120.343133354541,-119.348562004503,
-118.353990654465,-117.359419304428,-117.190326409342),.UNSPECIFIED.);
#180=B_SPLINE_CURVE_WITH_KNOTS('',3,(#22746,#22747,#22748,#22749,#22750,
#22751,#22752,#22753,#22754,#22755,#22756,#22757,#22758,#22759,#22760,#22761,
#22762,#22763,#22764,#22765,#22766,#22767,#22768,#22769,#22770),
 .UNSPECIFIED.,.F.,.F.,(4,3,3,3,3,3,3,3,4),(114.226969773278,114.375705254315,
115.370276604353,116.36484795439,117.359419304428,118.353990654465,119.348562004503,
120.343133354541,120.510155080457),.UNSPECIFIED.);
#181=B_SPLINE_CURVE_WITH_KNOTS('',3,(#22775,#22776,#22777,#22778,#22779,
#22780,#22781,#22782,#22783,#22784,#22785,#22786,#22787,#22788,#22789,#22790,
#22791,#22792,#22793,#22794,#22795,#22796),.UNSPECIFIED.,.F.,.F.,(4,3,3,
3,3,3,3,4),(-129.756697023701,-129.294275504878,-128.299704154841,-127.305132804803,
-126.310561454766,-125.315990104728,-124.321418754691,-123.473511716522),
 .UNSPECIFIED.);
#182=B_SPLINE_CURVE_WITH_KNOTS('',3,(#22797,#22798,#22799,#22800,#22801,
#22802,#22803,#22804,#22805,#22806,#22807,#22808,#22809,#22810,#22811,#22812,
#22813,#22814,#22815,#22816,#22817,#22818),.UNSPECIFIED.,.F.,.F.,(4,3,3,
3,3,3,3,4),(120.510155080457,121.337704704578,122.332276054616,123.326847404653,
124.321418754691,125.315990104728,126.310561454766,126.793340387637),
 .UNSPECIFIED.);
#183=B_SPLINE_CURVE_WITH_KNOTS('',3,(#22823,#22824,#22825,#22826,#22827,
#22828,#22829,#22830,#22831,#22832,#22833,#22834,#22835,#22836,#22837,#22838,
#22839,#22840,#22841,#22842,#22843,#22844),.UNSPECIFIED.,.F.,.F.,(4,3,3,
3,3,3,3,4),(-136.039882330881,-135.261703605103,-134.267132255066,-133.272560905028,
-132.277989554991,-131.283418204953,-130.288846854916,-129.756697023701),
 .UNSPECIFIED.);
#184=B_SPLINE_CURVE_WITH_KNOTS('',3,(#22845,#22846,#22847,#22848,#22849,
#22850,#22851,#22852,#22853,#22854,#22855,#22856,#22857,#22858,#22859,#22860,
#22861,#22862,#22863,#22864,#22865,#22866),.UNSPECIFIED.,.F.,.F.,(4,3,3,
3,3,3,3,4),(126.793340387637,127.305132804803,128.299704154841,129.294275504878,
130.288846854916,131.283418204953,132.277989554991,133.076525694817),
 .UNSPECIFIED.);
#185=B_SPLINE_CURVE_WITH_KNOTS('',3,(#22871,#22872,#22873,#22874,#22875,
#22876,#22877,#22878,#22879,#22880,#22881,#22882,#22883,#22884,#22885,#22886,
#22887,#22888,#22889,#22890,#22891,#22892,#22893,#22894,#22895),
 .UNSPECIFIED.,.F.,.F.,(4,3,3,3,3,3,3,3,4),(-142.32306763806,-142.223703055366,
-141.229131705329,-140.234560355291,-139.239989005253,-138.245417655216,
-137.250846305178,-136.256274955141,-136.039882330881),.UNSPECIFIED.);
#186=B_SPLINE_CURVE_WITH_KNOTS('',3,(#22896,#22897,#22898,#22899,#22900,
#22901,#22902,#22903,#22904,#22905,#22906,#22907,#22908,#22909,#22910,#22911,
#22912,#22913,#22914,#22915,#22916,#22917,#22918,#22919,#22920),
 .UNSPECIFIED.,.F.,.F.,(4,3,3,3,3,3,3,3,4),(133.076525694817,133.272560905028,
134.267132255066,135.261703605103,136.256274955141,137.250846305178,138.245417655216,
139.239989005254,139.359711001996),.UNSPECIFIED.);
#187=B_SPLINE_CURVE_WITH_KNOTS('',3,(#22925,#22926,#22927,#22928,#22929,
#22930,#22931,#22932,#22933,#22934,#22935,#22936,#22937,#22938,#22939,#22940,
#22941,#22942,#22943,#22944,#22945,#22946),.UNSPECIFIED.,.F.,.F.,(4,3,3,
3,3,3,3,4),(-148.60625294524,-148.191131155591,-147.196559805554,-146.201988455516,
-145.207417105479,-144.212845755441,-143.218274405404,-142.32306763806),
 .UNSPECIFIED.);
#188=B_SPLINE_CURVE_WITH_KNOTS('',3,(#22947,#22948,#22949,#22950,#22951,
#22952,#22953,#22954,#22955,#22956,#22957,#22958,#22959,#22960,#22961,#22962,
#22963,#22964,#22965,#22966,#22967,#22968),.UNSPECIFIED.,.F.,.F.,(4,3,3,
3,3,3,3,4),(139.359711001996,140.234560355291,141.229131705329,142.223703055366,
143.218274405404,144.212845755441,145.207417105479,145.642896309176),
 .UNSPECIFIED.);
#189=B_SPLINE_CURVE_WITH_KNOTS('',3,(#22973,#22974,#22975,#22976,#22977,
#22978,#22979,#22980,#22981,#22982,#22983,#22984,#22985,#22986,#22987,#22988,
#22989,#22990,#22991,#22992,#22993,#22994),.UNSPECIFIED.,.F.,.F.,(4,3,3,
3,3,3,3,4),(-154.88943825242,-154.158559255816,-153.163987905779,-152.169416555741,
-151.174845205704,-150.180273855666,-149.185702505629,-148.60625294524),
 .UNSPECIFIED.);
#190=B_SPLINE_CURVE_WITH_KNOTS('',3,(#22995,#22996,#22997,#22998,#22999,
#23000,#23001,#23002,#23003,#23004,#23005,#23006,#23007,#23008,#23009,#23010,
#23011,#23012,#23013,#23014,#23015,#23016),.UNSPECIFIED.,.F.,.F.,(4,3,3,
3,3,3,3,4),(145.642896309176,146.201988455516,147.196559805554,148.191131155591,
149.185702505629,150.180273855666,151.174845205704,151.926081616355),
 .UNSPECIFIED.);
#191=B_SPLINE_CURVE_WITH_KNOTS('',3,(#23021,#23022,#23023,#23024,#23025,
#23026,#23027,#23028,#23029,#23030,#23031,#23032,#23033,#23034,#23035,#23036,
#23037,#23038,#23039,#23040,#23041,#23042,#23043,#23044,#23045),
 .UNSPECIFIED.,.F.,.F.,(4,3,3,3,3,3,3,3,4),(-161.172623559599,-161.120558706079,
-160.125987356041,-159.131416006004,-158.136844655966,-157.142273305929,
-156.147701955891,-155.153130605854,-154.88943825242),.UNSPECIFIED.);
#192=B_SPLINE_CURVE_WITH_KNOTS('',3,(#23046,#23047,#23048,#23049,#23050,
#23051,#23052,#23053,#23054,#23055,#23056,#23057,#23058,#23059,#23060,#23061,
#23062,#23063,#23064,#23065,#23066,#23067,#23068,#23069,#23070),
 .UNSPECIFIED.,.F.,.F.,(4,3,3,3,3,3,3,3,4),(151.926081616355,152.169416555741,
153.163987905779,154.158559255816,155.153130605854,156.147701955891,157.142273305929,
158.136844655966,158.209266923535),.UNSPECIFIED.);
#193=B_SPLINE_CURVE_WITH_KNOTS('',3,(#23075,#23076,#23077,#23078,#23079,
#23080,#23081,#23082,#23083,#23084,#23085,#23086,#23087,#23088,#23089,#23090,
#23091,#23092,#23093,#23094,#23095,#23096),.UNSPECIFIED.,.F.,.F.,(4,3,3,
3,3,3,3,4),(-167.455808866779,-167.087986806304,-166.093415456267,-165.098844106229,
-164.104272756192,-163.109701406154,-162.115130056117,-161.172623559599),
 .UNSPECIFIED.);
#194=B_SPLINE_CURVE_WITH_KNOTS('',3,(#23097,#23098,#23099,#23100,#23101,
#23102,#23103,#23104,#23105,#23106,#23107,#23108,#23109,#23110,#23111,#23112,
#23113,#23114,#23115,#23116,#23117,#23118),.UNSPECIFIED.,.F.,.F.,(4,3,3,
3,3,3,3,4),(158.209266923535,159.131416006004,160.125987356042,161.120558706079,
162.115130056117,163.109701406154,164.104272756192,164.492452230714),
 .UNSPECIFIED.);
#195=B_SPLINE_CURVE_WITH_KNOTS('',3,(#23123,#23124,#23125,#23126,#23127,
#23128,#23129,#23130,#23131,#23132,#23133,#23134,#23135,#23136,#23137,#23138,
#23139,#23140,#23141,#23142,#23143,#23144),.UNSPECIFIED.,.F.,.F.,(4,3,3,
3,3,3,3,4),(-173.738994173958,-173.055414906529,-172.060843556492,-171.066272206454,
-170.071700856417,-169.077129506379,-168.082558156342,-167.455808866779),
 .UNSPECIFIED.);
#196=B_SPLINE_CURVE_WITH_KNOTS('',3,(#23145,#23146,#23147,#23148,#23149,
#23150,#23151,#23152,#23153,#23154,#23155,#23156,#23157,#23158,#23159,#23160,
#23161,#23162,#23163,#23164,#23165,#23166),.UNSPECIFIED.,.F.,.F.,(4,3,3,
3,3,3,3,4),(164.492452230714,165.098844106229,166.093415456267,167.087986806304,
168.082558156342,169.077129506379,170.071700856417,170.775637537894),
 .UNSPECIFIED.);
#197=B_SPLINE_CURVE_WITH_KNOTS('',3,(#23172,#23173,#23174,#23175,#23176,
#23177,#23178,#23179,#23180),.UNSPECIFIED.,.F.,.F.,(4,1,1,1,1,1,4),(179.070781254618,
179.697530544181,180.692101894219,181.686673244256,182.681244594294,183.675815944331,
184.578497523879),.UNSPECIFIED.);
#198=B_SPLINE_CURVE_WITH_KNOTS('',3,(#23183,#23184,#23185,#23186,#23187,
#23188,#23189,#23190),.UNSPECIFIED.,.F.,.F.,(4,1,1,1,1,4),(179.070781254618,
179.361415923179,180.355987273216,181.350558623254,182.345129973291,183.339701323329),
 .UNSPECIFIED.);
#199=B_SPLINE_CURVE_WITH_KNOTS('',3,(#23195,#23196,#23197,#23198,#23199,
#23200,#23201,#23202,#23203,#23204),.UNSPECIFIED.,.F.,.F.,(4,1,1,1,1,1,
1,4),(172.787595947439,173.730102443956,174.724673793994,175.719245144031,
176.713816494069,177.708387844106,178.702959194144,179.070781254618),
 .UNSPECIFIED.);
#200=B_SPLINE_CURVE_WITH_KNOTS('',3,(#23205,#23206,#23207,#23208,#23209,
#23210,#23211,#23212,#23213,#23214),.UNSPECIFIED.,.F.,.F.,(4,1,1,1,1,1,
1,4),(172.787595947439,173.393987822954,174.388559172991,175.383130523029,
176.377701873066,177.372273223104,178.366844573141,179.070781254618),
 .UNSPECIFIED.);
#201=B_SPLINE_CURVE_WITH_KNOTS('',3,(#23219,#23220,#23221,#23222,#23223,
#23224,#23225,#23226,#23227,#23228,#23229),.UNSPECIFIED.,.F.,.F.,(4,1,1,
1,1,1,1,1,4),(166.504410640259,166.768102993693,167.762674343731,168.757245693769,
169.751817043806,170.746388393844,171.740959743881,172.735531093919,172.787595947439),
 .UNSPECIFIED.);
#202=B_SPLINE_CURVE_WITH_KNOTS('',3,(#23230,#23231,#23232,#23233,#23234,
#23235,#23236,#23237,#23238,#23239),.UNSPECIFIED.,.F.,.F.,(4,1,1,1,1,1,
1,4),(166.504410640259,167.426559722728,168.421131072766,169.415702422803,
170.410273772841,171.404845122878,172.399416472916,172.787595947439),
 .UNSPECIFIED.);
#203=B_SPLINE_CURVE_WITH_KNOTS('',3,(#23244,#23245,#23246,#23247,#23248,
#23249,#23250,#23251,#23252,#23253),.UNSPECIFIED.,.F.,.F.,(4,1,1,1,1,1,
1,4),(160.22122533308,160.800674893468,161.795246243506,162.789817593543,
163.784388943581,164.778960293618,165.773531643656,166.504410640259),
 .UNSPECIFIED.);
#204=B_SPLINE_CURVE_WITH_KNOTS('',3,(#23254,#23255,#23256,#23257,#23258,
#23259,#23260,#23261,#23262,#23263,#23264),.UNSPECIFIED.,.F.,.F.,(4,1,1,
1,1,1,1,1,4),(160.22122533308,160.464560272466,161.459131622503,162.453702972541,
163.448274322578,164.442845672616,165.437417022653,166.431988372691,166.504410640259),
 .UNSPECIFIED.);
#205=B_SPLINE_CURVE_WITH_KNOTS('',3,(#23269,#23270,#23271,#23272,#23273,
#23274,#23275,#23276,#23277,#23278),.UNSPECIFIED.,.F.,.F.,(4,1,1,1,1,1,
1,4),(153.9380400259,154.833246793243,155.827818143281,156.822389493318,
157.816960843356,158.811532193393,159.806103543431,160.22122533308),
 .UNSPECIFIED.);
#206=B_SPLINE_CURVE_WITH_KNOTS('',3,(#23279,#23280,#23281,#23282,#23283,
#23284,#23285,#23286,#23287,#23288),.UNSPECIFIED.,.F.,.F.,(4,1,1,1,1,1,
1,4),(153.9380400259,154.497132172241,155.491703522278,156.486274872316,
157.480846222353,158.475417572391,159.469988922428,160.22122533308),
 .UNSPECIFIED.);
#207=B_SPLINE_CURVE_WITH_KNOTS('',3,(#23293,#23294,#23295,#23296,#23297,
#23298,#23299,#23300,#23301,#23302,#23303),.UNSPECIFIED.,.F.,.F.,(4,1,1,
1,1,1,1,1,4),(147.65485471872,147.87124734298,148.865818693018,149.860390043056,
150.854961393093,151.849532743131,152.844104093168,153.838675443206,153.9380400259),
 .UNSPECIFIED.);
#208=B_SPLINE_CURVE_WITH_KNOTS('',3,(#23304,#23305,#23306,#23307,#23308,
#23309,#23310,#23311,#23312,#23313),.UNSPECIFIED.,.F.,.F.,(4,1,1,1,1,1,
1,4),(147.65485471872,148.529704072015,149.524275422053,150.51884677209,
151.513418122128,152.507989472165,153.502560822203,153.9380400259),
 .UNSPECIFIED.);
#209=B_SPLINE_CURVE_WITH_KNOTS('',3,(#23318,#23319,#23320,#23321,#23322,
#23323,#23324,#23325,#23326,#23327),.UNSPECIFIED.,.F.,.F.,(4,1,1,1,1,1,
1,4),(141.371669411541,141.903819242755,142.898390592793,143.89296194283,
144.887533292868,145.882104642905,146.876675992943,147.65485471872),
 .UNSPECIFIED.);
#210=B_SPLINE_CURVE_WITH_KNOTS('',3,(#23328,#23329,#23330,#23331,#23332,
#23333,#23334,#23335,#23336,#23337,#23338),.UNSPECIFIED.,.F.,.F.,(4,1,1,
1,1,1,1,1,4),(141.371669411541,141.567704621753,142.56227597179,143.556847321828,
144.551418671865,145.545990021903,146.54056137194,147.535132721978,147.65485471872),
 .UNSPECIFIED.);
#211=B_SPLINE_CURVE_WITH_KNOTS('',3,(#23343,#23344,#23345,#23346,#23347,
#23348,#23349,#23350,#23351,#23352),.UNSPECIFIED.,.F.,.F.,(4,1,1,1,1,1,
1,4),(135.088484104361,135.93639114253,136.930962492568,137.925533842605,
138.920105192643,139.91467654268,140.909247892718,141.371669411541),
 .UNSPECIFIED.);
#212=B_SPLINE_CURVE_WITH_KNOTS('',3,(#23353,#23354,#23355,#23356,#23357,
#23358,#23359,#23360,#23361,#23362),.UNSPECIFIED.,.F.,.F.,(4,1,1,1,1,1,
1,4),(135.088484104361,135.600276521528,136.594847871565,137.589419221603,
138.58399057164,139.578561921678,140.573133271715,141.371669411541),
 .UNSPECIFIED.);
#213=B_SPLINE_CURVE_WITH_KNOTS('',3,(#23367,#23368,#23369,#23370,#23371,
#23372,#23373,#23374,#23375,#23376,#23377),.UNSPECIFIED.,.F.,.F.,(4,1,1,
1,1,1,1,1,4),(128.805298797182,128.974391692268,129.968963042305,130.963534392343,
131.95810574238,132.952677092418,133.947248442455,134.941819792493,135.088484104361),
 .UNSPECIFIED.);
#214=B_SPLINE_CURVE_WITH_KNOTS('',3,(#23378,#23379,#23380,#23381,#23382,
#23383,#23384,#23385,#23386,#23387),.UNSPECIFIED.,.F.,.F.,(4,1,1,1,1,1,
1,4),(128.805298797182,129.632848421302,130.62741977134,131.621991121377,
132.616562471415,133.611133821453,134.60570517149,135.088484104361),
 .UNSPECIFIED.);
#215=B_SPLINE_CURVE_WITH_KNOTS('',3,(#23392,#23393,#23394,#23395,#23396,
#23397,#23398,#23399,#23400,#23401),.UNSPECIFIED.,.F.,.F.,(4,1,1,1,1,1,
1,4),(122.522113490002,123.006963592042,124.00153494208,124.996106292117,
125.990677642155,126.985248992192,127.97982034223,128.805298797182),
 .UNSPECIFIED.);
#216=B_SPLINE_CURVE_WITH_KNOTS('',3,(#23402,#23403,#23404,#23405,#23406,
#23407,#23408,#23409,#23410,#23411,#23412),.UNSPECIFIED.,.F.,.F.,(4,1,1,
1,1,1,1,1,4),(122.522113490002,122.67084897104,123.665420321077,124.659991671115,
125.654563021152,126.64913437119,127.643705721227,128.638277071265,128.805298797182),
 .UNSPECIFIED.);
#217=B_SPLINE_CURVE_WITH_KNOTS('',3,(#23417,#23418,#23419,#23420,#23421,
#23422,#23423,#23424,#23425,#23426),.UNSPECIFIED.,.F.,.F.,(4,1,1,1,1,1,
1,4),(116.238928182823,117.039535491817,118.034106841855,119.028678191892,
120.02324954193,121.017820891967,122.012392242005,122.522113490002),
 .UNSPECIFIED.);
#218=B_SPLINE_CURVE_WITH_KNOTS('',3,(#23427,#23428,#23429,#23430,#23431,
#23432,#23433,#23434,#23435,#23436),.UNSPECIFIED.,.F.,.F.,(4,1,1,1,1,1,
1,4),(116.238928182823,116.703420870815,117.697992220852,118.69256357089,
119.687134920927,120.681706270965,121.676277621002,122.522113490002),
 .UNSPECIFIED.);
#219=B_SPLINE_CURVE_WITH_KNOTS('',3,(#23441,#23442,#23443,#23444,#23445,
#23446,#23447,#23448,#23449,#23450,#23451),.UNSPECIFIED.,.F.,.F.,(4,1,1,
1,1,1,1,1,4),(109.955742875643,110.077536041555,111.072107391592,112.06667874163,
113.061250091667,114.055821441705,115.050392791742,116.04496414178,116.238928182823),
 .UNSPECIFIED.);
#220=B_SPLINE_CURVE_WITH_KNOTS('',3,(#23452,#23453,#23454,#23455,#23456,
#23457,#23458,#23459,#23460,#23461),.UNSPECIFIED.,.F.,.F.,(4,1,1,1,1,1,
1,4),(109.955742875643,110.735992770589,111.730564120627,112.725135470664,
113.719706820702,114.71427817074,115.708849520777,116.238928182823),
 .UNSPECIFIED.);
#221=B_SPLINE_CURVE_WITH_KNOTS('',3,(#23466,#23467,#23468,#23469,#23470,
#23471,#23472,#23473,#23474,#23475),.UNSPECIFIED.,.F.,.F.,(4,1,1,1,1,1,
1,4),(103.672557568463,104.110107941329,105.104679291367,106.099250641404,
107.093821991442,108.08839334148,109.082964691517,109.955742875643),
 .UNSPECIFIED.);
#222=B_SPLINE_CURVE_WITH_KNOTS('',3,(#23476,#23477,#23478,#23479,#23480,
#23481,#23482,#23483,#23484,#23485,#23486),.UNSPECIFIED.,.F.,.F.,(4,1,1,
1,1,1,1,1,4),(103.672557568463,103.773993320327,104.768564670364,105.763136020402,
106.757707370439,107.752278720477,108.746850070514,109.741421420552,109.955742875643),
 .UNSPECIFIED.);
#223=B_SPLINE_CURVE_WITH_KNOTS('',3,(#23491,#23492,#23493,#23494,#23495,
#23496,#23497,#23498,#23499,#23500),.UNSPECIFIED.,.F.,.F.,(4,1,1,1,1,1,
1,4),(97.3893722612837,98.1426798411043,99.1372511911418,100.131822541179,
101.126393891217,102.120965241254,103.115536591292,103.672557568463),
 .UNSPECIFIED.);
#224=B_SPLINE_CURVE_WITH_KNOTS('',3,(#23501,#23502,#23503,#23504,#23505,
#23506,#23507,#23508,#23509,#23510),.UNSPECIFIED.,.F.,.F.,(4,1,1,1,1,1,
1,4),(97.3893722612837,97.8065652201016,98.8011365701391,99.7957079201767,
100.790279270214,101.784850620252,102.779421970289,103.672557568463),
 .UNSPECIFIED.);
#225=B_SPLINE_CURVE_WITH_KNOTS('',3,(#23515,#23516,#23517,#23518,#23519,
#23520,#23521,#23522,#23523,#23524,#23525),.UNSPECIFIED.,.F.,.F.,(4,1,1,
1,1,1,1,1,4),(91.1061869541041,91.1806803908416,92.1752517408791,93.1698230909166,
94.1643944409542,95.1589657909917,96.1535371410292,97.1481084910667,97.3893722612837),
 .UNSPECIFIED.);
#226=B_SPLINE_CURVE_WITH_KNOTS('',3,(#23526,#23527,#23528,#23529,#23530,
#23531,#23532,#23533,#23534,#23535),.UNSPECIFIED.,.F.,.F.,(4,1,1,1,1,1,
1,4),(91.1061869541041,91.8391371198765,92.833708469914,93.8282798199515,
94.822851169989,95.8174225200266,96.8119938700641,97.3893722612837),
 .UNSPECIFIED.);
#227=B_SPLINE_CURVE_WITH_KNOTS('',3,(#23540,#23541,#23542,#23543,#23544,
#23545,#23546,#23547,#23548,#23549),.UNSPECIFIED.,.F.,.F.,(4,1,1,1,1,1,
1,4),(84.8230016469245,85.2132522906164,86.207823640654,87.2023949906915,
88.196966340729,89.1915376907665,90.1861090408041,91.1061869541041),
 .UNSPECIFIED.);
#228=B_SPLINE_CURVE_WITH_KNOTS('',3,(#23550,#23551,#23552,#23553,#23554,
#23555,#23556,#23557,#23558,#23559,#23560),.UNSPECIFIED.,.F.,.F.,(4,1,1,
1,1,1,1,1,4),(84.8230016469246,84.8771376696138,85.8717090196513,86.8662803696888,
87.8608517197264,88.8554230697639,89.8499944198014,90.8445657698389,91.1061869541041),
 .UNSPECIFIED.);
#229=B_SPLINE_CURVE_WITH_KNOTS('',3,(#23565,#23566,#23567,#23568,#23569,
#23570,#23571,#23572,#23573,#23574),.UNSPECIFIED.,.F.,.F.,(4,1,1,1,1,1,
1,4),(78.539816339745,79.2458241903913,80.2403955404288,81.2349668904663,
82.2295382405039,83.2241095905414,84.2186809405789,84.8230016469245),
 .UNSPECIFIED.);
#230=B_SPLINE_CURVE_WITH_KNOTS('',3,(#23575,#23576,#23577,#23578,#23579,
#23580,#23581,#23582,#23583,#23584),.UNSPECIFIED.,.F.,.F.,(4,1,1,1,1,1,
1,4),(78.539816339745,78.9097095693886,79.9042809194262,80.8988522694637,
81.8934236195012,82.8879949695387,83.8825663195763,84.8230016469246),
 .UNSPECIFIED.);
#231=B_SPLINE_CURVE_WITH_KNOTS('',3,(#23589,#23590,#23591,#23592,#23593,
#23594,#23595,#23596,#23597,#23598,#23599),.UNSPECIFIED.,.F.,.F.,(4,1,1,
1,1,1,1,1,4),(72.2566310325654,72.2838247401286,73.2783960901661,74.2729674402037,
75.2675387902412,76.2621101402787,77.2566814903162,78.2512528403538,78.539816339745),
 .UNSPECIFIED.);
#232=B_SPLINE_CURVE_WITH_KNOTS('',3,(#23600,#23601,#23602,#23603,#23604,
#23605,#23606,#23607,#23608,#23609),.UNSPECIFIED.,.F.,.F.,(4,1,1,1,1,1,
1,4),(72.2566310325654,72.9422814691635,73.936852819201,74.9314241692385,
75.9259955192761,76.9205668693136,77.9151382193511,78.539816339745),
 .UNSPECIFIED.);
#233=B_SPLINE_CURVE_WITH_KNOTS('',3,(#23614,#23615,#23616,#23617,#23618,
#23619,#23620,#23621,#23622,#23623),.UNSPECIFIED.,.F.,.F.,(4,1,1,1,1,1,
1,4),(65.9734457253857,66.3163966399035,67.310967989941,68.3055393399785,
69.300110690016,70.2946820400536,71.2892533900911,72.2566310325654),
 .UNSPECIFIED.);
#234=B_SPLINE_CURVE_WITH_KNOTS('',3,(#23624,#23625,#23626,#23627,#23628,
#23629,#23630,#23631,#23632,#23633,#23634),.UNSPECIFIED.,.F.,.F.,(4,1,1,
1,1,1,1,1,4),(65.9734457253857,65.9802820189008,66.9748533689383,67.9694247189759,
68.9639960690134,69.9585674190509,70.9531387690884,71.947710119126,72.2566310325654),
 .UNSPECIFIED.);
#235=B_SPLINE_CURVE_WITH_KNOTS('',3,(#23639,#23640,#23641,#23642,#23643,
#23644,#23645,#23646,#23647,#23648),.UNSPECIFIED.,.F.,.F.,(4,1,1,1,1,1,
1,4),(59.6902604182062,60.3489685396783,61.3435398897158,62.3381112397534,
63.3326825897909,64.3272539398284,65.3218252898659,65.9734457253857),
 .UNSPECIFIED.);
#236=B_SPLINE_CURVE_WITH_KNOTS('',3,(#23649,#23650,#23651,#23652,#23653,
#23654,#23655,#23656,#23657,#23658),.UNSPECIFIED.,.F.,.F.,(4,1,1,1,1,1,
1,4),(59.6902604182062,60.0128539186757,61.0074252687132,62.0019966187507,
62.9965679687882,63.9911393188258,64.9857106688633,65.9734457253857),
 .UNSPECIFIED.);
#237=B_SPLINE_CURVE_WITH_KNOTS('',3,(#23663,#23664,#23665,#23666,#23667,
#23668,#23669,#23670,#23671,#23672),.UNSPECIFIED.,.F.,.F.,(4,1,1,1,1,1,
1,4),(53.4070751110266,54.3815404394532,55.3761117894907,56.3706831395282,
57.3652544895657,58.3598258396033,59.3543971896408,59.6902604182062),
 .UNSPECIFIED.);
#238=B_SPLINE_CURVE_WITH_KNOTS('',3,(#23673,#23674,#23675,#23676,#23677,
#23678,#23679,#23680,#23681,#23682),.UNSPECIFIED.,.F.,.F.,(4,1,1,1,1,1,
1,4),(53.4070751110266,54.0454258184505,55.039997168488,56.0345685185256,
57.0291398685631,58.0237112186006,59.0182825686381,59.6902604182062),
 .UNSPECIFIED.);
#239=B_SPLINE_CURVE_WITH_KNOTS('',3,(#23687,#23688,#23689,#23690,#23691,
#23692,#23693,#23694,#23695,#23696,#23697),.UNSPECIFIED.,.F.,.F.,(4,1,1,
1,1,1,1,1,4),(47.123889803847,47.4195409891905,48.414112339228,49.4086836892655,
50.4032550393031,51.3978263893406,52.3923977393781,53.3869690894156,53.4070751110266),
 .UNSPECIFIED.);
#240=B_SPLINE_CURVE_WITH_KNOTS('',3,(#23698,#23699,#23700,#23701,#23702,
#23703,#23704,#23705,#23706,#23707),.UNSPECIFIED.,.F.,.F.,(4,1,1,1,1,1,
1,4),(47.123889803847,48.0779977182254,49.0725690682629,50.0671404183004,
51.061711768338,52.0562831183755,53.050854468413,53.4070751110266),
 .UNSPECIFIED.);
#241=B_SPLINE_CURVE_WITH_KNOTS('',3,(#23712,#23713,#23714,#23715,#23716,
#23717,#23718,#23719,#23720,#23721),.UNSPECIFIED.,.F.,.F.,(4,1,1,1,1,1,
1,4),(40.8407044966674,41.4521128889653,42.4466842390029,43.4412555890404,
44.4358269390779,45.4303982891154,46.424969639153,47.123889803847),
 .UNSPECIFIED.);
#242=B_SPLINE_CURVE_WITH_KNOTS('',3,(#23722,#23723,#23724,#23725,#23726,
#23727,#23728,#23729,#23730,#23731,#23732),.UNSPECIFIED.,.F.,.F.,(4,1,1,
1,1,1,1,1,4),(40.8407044966674,41.1159982679627,42.1105696180002,43.1051409680378,
44.0997123180753,45.0942836681128,46.0888550181503,47.0834263681879,47.123889803847),
 .UNSPECIFIED.);
#243=B_SPLINE_CURVE_WITH_KNOTS('',3,(#23737,#23738,#23739,#23740,#23741,
#23742,#23743,#23744,#23745,#23746),.UNSPECIFIED.,.F.,.F.,(4,1,1,1,1,1,
1,4),(34.5575191894878,35.4846847887402,36.4792561387777,37.4738274888152,
38.4683988388528,39.4629701888903,40.4575415389278,40.8407044966674),
 .UNSPECIFIED.);
#244=B_SPLINE_CURVE_WITH_KNOTS('',3,(#23747,#23748,#23749,#23750,#23751,
#23752,#23753,#23754,#23755,#23756),.UNSPECIFIED.,.F.,.F.,(4,1,1,1,1,1,
1,4),(34.5575191894878,35.1485701677375,36.1431415177751,37.1377128678126,
38.1322842178501,39.1268555678876,40.1214269179252,40.8407044966674),
 .UNSPECIFIED.);
#245=B_SPLINE_CURVE_WITH_KNOTS('',3,(#23761,#23762,#23763,#23764,#23765,
#23766,#23767,#23768,#23769,#23770,#23771),.UNSPECIFIED.,.F.,.F.,(4,1,1,
1,1,1,1,1,4),(28.2743338823082,28.5226853384775,29.517256688515,30.5118280385526,
31.5063993885901,32.5009707386276,33.4955420886651,34.4901134387027,34.5575191894878),
 .UNSPECIFIED.);
#246=B_SPLINE_CURVE_WITH_KNOTS('',3,(#23772,#23773,#23774,#23775,#23776,
#23777,#23778,#23779,#23780,#23781),.UNSPECIFIED.,.F.,.F.,(4,1,1,1,1,1,
1,4),(28.2743338823082,29.1811420675124,30.1757134175499,31.1702847675875,
32.164856117625,33.1594274676625,34.1539988177,34.5575191894878),
 .UNSPECIFIED.);
#247=B_SPLINE_CURVE_WITH_KNOTS('',3,(#23786,#23787,#23788,#23789,#23790,
#23791,#23792,#23793,#23794,#23795),.UNSPECIFIED.,.F.,.F.,(4,1,1,1,1,1,
1,4),(21.9911485751286,22.5552572382524,23.5498285882899,24.5443999383274,
25.5389712883649,26.5335426384025,27.52811398844,28.2743338823082),
 .UNSPECIFIED.);
#248=B_SPLINE_CURVE_WITH_KNOTS('',3,(#23796,#23797,#23798,#23799,#23800,
#23801,#23802,#23803,#23804,#23805,#23806),.UNSPECIFIED.,.F.,.F.,(4,1,1,
1,1,1,1,1,4),(21.9911485751286,22.2191426172497,23.2137139672872,24.2082853173248,
25.2028566673623,26.1974280173998,27.1919993674374,28.1865707174749,28.2743338823082),
 .UNSPECIFIED.);
#249=B_SPLINE_CURVE_WITH_KNOTS('',3,(#23811,#23812,#23813,#23814,#23815,
#23816,#23817,#23818,#23819,#23820),.UNSPECIFIED.,.F.,.F.,(4,1,1,1,1,1,
1,4),(15.707963267949,16.5878291380272,17.5824004880647,18.5769718381023,
19.5715431881398,20.5661145381773,21.5606858882148,21.9911485751286),
 .UNSPECIFIED.);
#250=B_SPLINE_CURVE_WITH_KNOTS('',3,(#23821,#23822,#23823,#23824,#23825,
#23826,#23827,#23828,#23829,#23830),.UNSPECIFIED.,.F.,.F.,(4,1,1,1,1,1,
1,4),(15.707963267949,16.2517145170246,17.2462858670621,18.2408572170996,
19.2354285671371,20.2299999171747,21.2245712672122,21.9911485751286),
 .UNSPECIFIED.);
#251=B_SPLINE_CURVE_WITH_KNOTS('',3,(#24063,#24064,#24065,#24066,#24067,
#24068,#24069,#24070,#24071,#24072,#24073,#24074,#24075,#24076,#24077,#24078,
#24079,#24080,#24081,#24082,#24083,#24084,#24085,#24086,#24087,#24088,#24089,
#24090,#24091,#24092,#24093,#24094,#24095,#24096,#24097,#24098,#24099,#24100,
#24101,#24102,#24103,#24104,#24105,#24106,#24107,#24108,#24109,#24110,#24111,
#24112,#24113,#24114,#24115,#24116,#24117,#24118,#24119,#24120,#24121,#24122,
#24123,#24124,#24125,#24126,#24127,#24128,#24129,#24130,#24131,#24132,#24133,
#24134,#24135,#24136,#24137,#24138,#24139,#24140,#24141,#24142,#24143,#24144,
#24145,#24146,#24147,#24148,#24149,#24150,#24151,#24152,#24153,#24154,#24155,
#24156,#24157,#24158,#24159),.UNSPECIFIED.,.F.,.F.,(4,3,3,3,3,3,3,3,3,3,
3,3,3,3,3,3,3,3,3,3,3,3,3,3,3,3,3,3,3,3,3,3,4),(-0.780432929098692,-0.744171076506414,
-0.707269362542449,-0.685703619005375,-0.677641063801082,-0.671987810898122,
-0.635377863422115,-0.601232813738007,-0.58629435450121,-0.577918583648485,
-0.570482007246046,-0.534001224941446,-0.497606122019792,-0.462171004484833,
-0.437182619850938,-0.428169806816731,-0.422783055253062,-0.387505838307544,
-0.362217465949252,-0.326639251159082,-0.290748131513672,-0.281156185824485,
-0.276193604589621,-0.241028956991022,-0.205655214290034,-0.170550703428344,
-0.149231865499801,-0.141809112984284,-0.135579482248505,-0.100965757631287,
-0.0667517818268251,-0.0333758909134126,0.),.UNSPECIFIED.);
#252=B_SPLINE_CURVE_WITH_KNOTS('',3,(#24160,#24161,#24162,#24163,#24164,
#24165,#24166,#24167,#24168,#24169,#24170,#24171,#24172,#24173,#24174,#24175,
#24176,#24177,#24178,#24179,#24180,#24181,#24182,#24183,#24184,#24185,#24186,
#24187,#24188,#24189,#24190,#24191,#24192,#24193,#24194,#24195,#24196,#24197,
#24198,#24199,#24200,#24201,#24202,#24203,#24204,#24205,#24206,#24207,#24208,
#24209,#24210,#24211,#24212,#24213,#24214,#24215,#24216,#24217,#24218,#24219,
#24220,#24221,#24222,#24223,#24224,#24225,#24226,#24227,#24228,#24229,#24230,
#24231,#24232,#24233,#24234,#24235,#24236,#24237,#24238,#24239,#24240,#24241,
#24242,#24243,#24244,#24245,#24246,#24247,#24248,#24249,#24250,#24251,#24252,
#24253,#24254,#24255,#24256),.UNSPECIFIED.,.F.,.F.,(4,3,3,3,3,3,3,3,3,3,
3,3,3,3,3,3,3,3,3,3,3,3,3,3,3,3,3,3,3,3,3,3,4),(-0.782320427274638,-0.749691875557366,
-0.716079002773824,-0.69538894405227,-0.688774800459675,-0.682477718221598,
-0.648343944567492,-0.615430709400175,-0.601031169014474,-0.592885555855582,
-0.587118698134123,-0.551838327246284,-0.516166914508928,-0.48087202150747,
-0.456913531937842,-0.450542037325468,-0.445610077462954,-0.409473029571469,
-0.385038063228958,-0.349835104468143,-0.31400993863385,-0.305067953562657,
-0.298844713484155,-0.261489124298636,-0.224910226260933,-0.188134349953557,
-0.164617556209363,-0.155035509146063,-0.149135266247745,-0.111810553481794,
-0.0745528270350788,-0.0372764135175394,0.),.UNSPECIFIED.);
#253=B_SPLINE_CURVE_WITH_KNOTS('',3,(#24973,#24974,#24975,#24976,#24977,
#24978,#24979,#24980,#24981,#24982),.UNSPECIFIED.,.F.,.F.,(4,3,3,4),(170.775637537894,
171.066272206454,172.060843556492,172.96352513604),.UNSPECIFIED.);
#254=B_SPLINE_CURVE_WITH_KNOTS('',3,(#24984,#24985,#24986,#24987,#24988,
#24989,#24990,#24991,#24992,#24993,#24994,#24995,#24996,#24997,#24998,#24999,
#25000,#25001,#25002,#25003,#25004,#25005,#25006,#25007,#25008,#25009,#25010,
#25011,#25012,#25013,#25014,#25015,#25016,#25017,#25018,#25019,#25020,#25021,
#25022,#25023,#25024,#25025,#25026,#25027,#25028,#25029,#25030,#25031,#25032,
#25033,#25034,#25035,#25036,#25037,#25038,#25039,#25040,#25041,#25042,#25043,
#25044,#25045,#25046,#25047,#25048,#25049,#25050,#25051,#25052,#25053,#25054,
#25055,#25056,#25057,#25058,#25059,#25060,#25061,#25062,#25063,#25064,#25065,
#25066,#25067,#25068,#25069,#25070,#25071,#25072,#25073,#25074,#25075,#25076,
#25077,#25078,#25079,#25080),.UNSPECIFIED.,.F.,.F.,(4,3,3,3,3,3,3,3,3,3,
3,3,3,3,3,3,3,3,3,3,3,3,3,3,3,3,3,3,3,3,3,3,4),(-0.782320427274655,-0.749691875557393,
-0.716078998607798,-0.695388940146623,-0.688774779534789,-0.68247771551652,
-0.648343938050999,-0.615430703698248,-0.601031163668919,-0.592885529328257,
-0.587118690997954,-0.551838318465963,-0.516166905662748,-0.48087201177489,
-0.456913524638415,-0.450542066424711,-0.445610092428472,-0.409473044351031,
-0.385038063228989,-0.349835101082961,-0.314009932195594,-0.305067936627418,
-0.298844709169275,-0.261489120523116,-0.224910219813707,-0.188134343389742,
-0.164617550466024,-0.155035492002945,-0.149135262336089,-0.111810548816022,
-0.074552824760043,-0.0372764123800215,0.),.UNSPECIFIED.);
#255=B_SPLINE_CURVE_WITH_KNOTS('',3,(#25081,#25082,#25083,#25084,#25085,
#25086,#25087,#25088,#25089),.UNSPECIFIED.,.F.,.F.,(4,1,1,1,1,1,4),(10.3761761872891,
11.2788577668369,12.2734291168745,13.268000466912,14.2625718169495,15.257143166987,
15.707963267949),.UNSPECIFIED.);
#256=B_SPLINE_CURVE_WITH_KNOTS('',3,(#25095,#25096,#25097,#25098,#25099,
#25100,#25101,#25102,#25103,#25104,#25105,#25106,#25107,#25108,#25109,#25110,
#25111,#25112,#25113,#25114,#25115,#25116,#25117,#25118,#25119,#25120,#25121,
#25122,#25123,#25124,#25125,#25126,#25127,#25128,#25129,#25130,#25131,#25132,
#25133,#25134,#25135,#25136,#25137,#25138,#25139,#25140,#25141,#25142,#25143,
#25144,#25145,#25146,#25147,#25148,#25149,#25150,#25151,#25152,#25153,#25154,
#25155,#25156,#25157,#25158,#25159,#25160,#25161,#25162,#25163,#25164,#25165,
#25166,#25167,#25168,#25169,#25170,#25171,#25172,#25173,#25174,#25175,#25176,
#25177,#25178,#25179,#25180,#25181,#25182,#25183,#25184,#25185,#25186,#25187,
#25188,#25189,#25190,#25191),.UNSPECIFIED.,.F.,.F.,(4,3,3,3,3,3,3,3,3,3,
3,3,3,3,3,3,3,3,3,3,3,3,3,3,3,3,3,3,3,3,3,3,4),(-0.780432929098614,-0.744171076506339,
-0.70726936348061,-0.685703619884899,-0.677641067625544,-0.671987820717708,
-0.635377874072834,-0.601232823057384,-0.586294363238125,-0.577918591325873,
-0.570482007745035,-0.534001225423256,-0.497606123558654,-0.462171010723763,
-0.437182624530132,-0.428169820114518,-0.422783054578572,-0.387505840929447,
-0.362217465949239,-0.326639254971974,-0.290748136090389,-0.281156242639861,
-0.27619361681087,-0.241028972315843,-0.205655229311345,-0.170550714021067,
-0.149231874768433,-0.141809159915445,-0.135579488063576,-0.100965760056957,
-0.0667517778475045,-0.0333758889237523,0.),.UNSPECIFIED.);
#257=B_SPLINE_CURVE_WITH_KNOTS('',3,(#25194,#25195,#25196,#25197,#25198,
#25199,#25200,#25201),.UNSPECIFIED.,.F.,.F.,(4,1,1,1,1,4),(11.6149723878396,
12.6095437378771,13.6041150879146,14.5986864379522,15.5932577879897,15.707963267949),
 .UNSPECIFIED.);
#258=B_SPLINE_CURVE_WITH_KNOTS('',3,(#25918,#25919,#25920,#25921,#25922,
#25923,#25924),.UNSPECIFIED.,.F.,.F.,(4,3,4),(-175.044557606604,-174.049986256567,
-173.738994173958),.UNSPECIFIED.);
#594=SHAPE_REPRESENTATION_RELATIONSHIP('SRR','None',#37244,#607);
#607=ADVANCED_BREP_SHAPE_REPRESENTATION('',(#633),#37174);
#620=STYLED_ITEM('',(#37387),#633);
#633=MANIFOLD_SOLID_BREP('Body1',#14782);
#676=FACE_BOUND('',#2678,.T.);
#677=FACE_BOUND('',#2784,.T.);
#727=CYLINDRICAL_SURFACE('',#15456,3.954);
#728=CYLINDRICAL_SURFACE('',#15458,3.954);
#729=CYLINDRICAL_SURFACE('',#15459,3.954);
#730=CYLINDRICAL_SURFACE('',#15460,3.954);
#731=CYLINDRICAL_SURFACE('',#15461,3.954);
#732=CYLINDRICAL_SURFACE('',#15462,3.954);
#733=CYLINDRICAL_SURFACE('',#15463,3.954);
#734=CYLINDRICAL_SURFACE('',#15464,3.954);
#735=CYLINDRICAL_SURFACE('',#15465,3.954);
#736=CYLINDRICAL_SURFACE('',#15466,3.954);
#737=CYLINDRICAL_SURFACE('',#15467,3.954);
#738=CYLINDRICAL_SURFACE('',#15468,3.954);
#739=CYLINDRICAL_SURFACE('',#15469,3.954);
#740=CYLINDRICAL_SURFACE('',#15470,3.954);
#741=CYLINDRICAL_SURFACE('',#15471,3.954);
#742=CYLINDRICAL_SURFACE('',#15472,3.954);
#743=CYLINDRICAL_SURFACE('',#15473,3.954);
#744=CYLINDRICAL_SURFACE('',#15474,3.954);
#745=CYLINDRICAL_SURFACE('',#15475,3.954);
#746=CYLINDRICAL_SURFACE('',#15476,3.954);
#747=CYLINDRICAL_SURFACE('',#15477,3.954);
#748=CYLINDRICAL_SURFACE('',#15478,3.954);
#749=CYLINDRICAL_SURFACE('',#15479,3.954);
#750=CYLINDRICAL_SURFACE('',#15480,3.954);
#751=CYLINDRICAL_SURFACE('',#15481,3.954);
#752=CYLINDRICAL_SURFACE('',#15482,3.954);
#753=CYLINDRICAL_SURFACE('',#15483,3.954);
#754=CYLINDRICAL_SURFACE('',#15484,3.954);
#755=CYLINDRICAL_SURFACE('',#15485,3.52375);
#756=CYLINDRICAL_SURFACE('',#15487,3.52375);
#757=CYLINDRICAL_SURFACE('',#15488,3.52375);
#758=CYLINDRICAL_SURFACE('',#15489,3.52375);
#759=CYLINDRICAL_SURFACE('',#15490,3.52375);
#760=CYLINDRICAL_SURFACE('',#15491,3.52375);
#761=CYLINDRICAL_SURFACE('',#15492,3.52375);
#762=CYLINDRICAL_SURFACE('',#15493,3.52375);
#763=CYLINDRICAL_SURFACE('',#15494,3.52375);
#764=CYLINDRICAL_SURFACE('',#15495,3.52375);
#765=CYLINDRICAL_SURFACE('',#15496,3.52375);
#766=CYLINDRICAL_SURFACE('',#15497,3.52375);
#767=CYLINDRICAL_SURFACE('',#15498,3.52375);
#768=CYLINDRICAL_SURFACE('',#15499,3.52375);
#769=CYLINDRICAL_SURFACE('',#15500,3.52375);
#770=CYLINDRICAL_SURFACE('',#15501,3.52375);
#771=CYLINDRICAL_SURFACE('',#15502,3.52375);
#772=CYLINDRICAL_SURFACE('',#15503,3.52375);
#773=CYLINDRICAL_SURFACE('',#15504,3.52375);
#774=CYLINDRICAL_SURFACE('',#15505,3.52375);
#775=CYLINDRICAL_SURFACE('',#15506,3.52375);
#776=CYLINDRICAL_SURFACE('',#15507,3.52375);
#777=CYLINDRICAL_SURFACE('',#15508,3.52375);
#778=CYLINDRICAL_SURFACE('',#15509,3.52375);
#779=CYLINDRICAL_SURFACE('',#15510,3.52375);
#780=CYLINDRICAL_SURFACE('',#15511,3.52375);
#781=CYLINDRICAL_SURFACE('',#15512,3.52375);
#782=CYLINDRICAL_SURFACE('',#15564,5.);
#783=CYLINDRICAL_SURFACE('',#15597,3.52375);
#784=CYLINDRICAL_SURFACE('',#15697,3.954);
#785=CYLINDRICAL_SURFACE('',#15702,3.);
#1096=CIRCLE('',#15457,3.954);
#1097=CIRCLE('',#15486,3.52375);
#1098=CIRCLE('',#15514,5.);
#1099=CIRCLE('',#15515,4.6);
#1100=CIRCLE('',#15516,5.);
#1101=CIRCLE('',#15517,5.);
#1102=CIRCLE('',#15518,5.);
#1103=CIRCLE('',#15519,5.);
#1104=CIRCLE('',#15520,5.);
#1105=CIRCLE('',#15521,5.);
#1106=CIRCLE('',#15522,5.);
#1107=CIRCLE('',#15523,5.);
#1108=CIRCLE('',#15524,5.);
#1109=CIRCLE('',#15525,5.);
#1110=CIRCLE('',#15526,5.);
#1111=CIRCLE('',#15527,5.);
#1112=CIRCLE('',#15528,5.);
#1113=CIRCLE('',#15529,5.);
#1114=CIRCLE('',#15530,5.);
#1115=CIRCLE('',#15531,5.);
#1116=CIRCLE('',#15532,5.);
#1117=CIRCLE('',#15533,5.);
#1118=CIRCLE('',#15534,5.);
#1119=CIRCLE('',#15535,5.);
#1120=CIRCLE('',#15536,5.);
#1121=CIRCLE('',#15537,5.);
#1122=CIRCLE('',#15538,5.);
#1123=CIRCLE('',#15539,5.);
#1124=CIRCLE('',#15540,5.);
#1125=CIRCLE('',#15541,5.);
#1126=CIRCLE('',#15542,5.);
#1127=CIRCLE('',#15543,5.);
#1128=CIRCLE('',#15544,5.);
#1129=CIRCLE('',#15545,5.);
#1130=CIRCLE('',#15546,5.);
#1131=CIRCLE('',#15547,5.);
#1132=CIRCLE('',#15548,5.);
#1133=CIRCLE('',#15549,5.);
#1134=CIRCLE('',#15550,5.);
#1135=CIRCLE('',#15551,5.);
#1136=CIRCLE('',#15552,5.);
#1137=CIRCLE('',#15553,5.);
#1138=CIRCLE('',#15554,5.);
#1139=CIRCLE('',#15555,5.);
#1140=CIRCLE('',#15556,5.);
#1141=CIRCLE('',#15557,5.);
#1142=CIRCLE('',#15558,5.);
#1143=CIRCLE('',#15559,5.);
#1144=CIRCLE('',#15560,5.);
#1145=CIRCLE('',#15561,5.);
#1146=CIRCLE('',#15562,5.);
#1147=CIRCLE('',#15563,5.);
#1148=CIRCLE('',#15565,5.);
#1149=CIRCLE('',#15566,5.);
#1150=CIRCLE('',#15567,5.);
#1151=CIRCLE('',#15568,5.);
#1152=CIRCLE('',#15569,5.);
#1153=CIRCLE('',#15570,5.);
#1154=CIRCLE('',#15571,5.);
#1155=CIRCLE('',#15572,5.);
#1156=CIRCLE('',#15573,5.);
#1157=CIRCLE('',#15574,5.);
#1158=CIRCLE('',#15575,5.);
#1159=CIRCLE('',#15576,5.);
#1160=CIRCLE('',#15577,5.);
#1161=CIRCLE('',#15578,5.);
#1162=CIRCLE('',#15579,5.);
#1163=CIRCLE('',#15580,5.);
#1164=CIRCLE('',#15581,5.);
#1165=CIRCLE('',#15582,5.);
#1166=CIRCLE('',#15583,5.);
#1167=CIRCLE('',#15584,5.);
#1168=CIRCLE('',#15585,5.);
#1169=CIRCLE('',#15586,5.);
#1170=CIRCLE('',#15587,5.);
#1171=CIRCLE('',#15588,5.);
#1172=CIRCLE('',#15589,5.);
#1173=CIRCLE('',#15590,5.);
#1174=CIRCLE('',#15592,3.954);
#1175=CIRCLE('',#15594,3.954);
#1176=CIRCLE('',#15595,3.954);
#1177=CIRCLE('',#15596,3.52375);
#1178=CIRCLE('',#15695,3.6);
#1179=CIRCLE('',#15699,4.5);
#1180=CIRCLE('',#15701,3.);
#1181=CIRCLE('',#15703,3.);
#1349=CONICAL_SURFACE('',#15513,4.8,0.785398163397448);
#1350=CONICAL_SURFACE('',#15696,3.8,0.785398163397448);
#1351=CONICAL_SURFACE('',#15698,4.75,0.785398163397446);
#1744=FACE_OUTER_BOUND('',#2620,.T.);
#1745=FACE_OUTER_BOUND('',#2621,.T.);
#1746=FACE_OUTER_BOUND('',#2622,.T.);
#1747=FACE_OUTER_BOUND('',#2623,.T.);
#1748=FACE_OUTER_BOUND('',#2624,.T.);
#1749=FACE_OUTER_BOUND('',#2625,.T.);
#1750=FACE_OUTER_BOUND('',#2626,.T.);
#1751=FACE_OUTER_BOUND('',#2627,.T.);
#1752=FACE_OUTER_BOUND('',#2628,.T.);
#1753=FACE_OUTER_BOUND('',#2629,.T.);
#1754=FACE_OUTER_BOUND('',#2630,.T.);
#1755=FACE_OUTER_BOUND('',#2631,.T.);
#1756=FACE_OUTER_BOUND('',#2632,.T.);
#1757=FACE_OUTER_BOUND('',#2633,.T.);
#1758=FACE_OUTER_BOUND('',#2634,.T.);
#1759=FACE_OUTER_BOUND('',#2635,.T.);
#1760=FACE_OUTER_BOUND('',#2636,.T.);
#1761=FACE_OUTER_BOUND('',#2637,.T.);
#1762=FACE_OUTER_BOUND('',#2638,.T.);
#1763=FACE_OUTER_BOUND('',#2639,.T.);
#1764=FACE_OUTER_BOUND('',#2640,.T.);
#1765=FACE_OUTER_BOUND('',#2641,.T.);
#1766=FACE_OUTER_BOUND('',#2642,.T.);
#1767=FACE_OUTER_BOUND('',#2643,.T.);
#1768=FACE_OUTER_BOUND('',#2644,.T.);
#1769=FACE_OUTER_BOUND('',#2645,.T.);
#1770=FACE_OUTER_BOUND('',#2646,.T.);
#1771=FACE_OUTER_BOUND('',#2647,.T.);
#1772=FACE_OUTER_BOUND('',#2648,.T.);
#1773=FACE_OUTER_BOUND('',#2649,.T.);
#1774=FACE_OUTER_BOUND('',#2650,.T.);
#1775=FACE_OUTER_BOUND('',#2651,.T.);
#1776=FACE_OUTER_BOUND('',#2652,.T.);
#1777=FACE_OUTER_BOUND('',#2653,.T.);
#1778=FACE_OUTER_BOUND('',#2654,.T.);
#1779=FACE_OUTER_BOUND('',#2655,.T.);
#1780=FACE_OUTER_BOUND('',#2656,.T.);
#1781=FACE_OUTER_BOUND('',#2657,.T.);
#1782=FACE_OUTER_BOUND('',#2658,.T.);
#1783=FACE_OUTER_BOUND('',#2659,.T.);
#1784=FACE_OUTER_BOUND('',#2660,.T.);
#1785=FACE_OUTER_BOUND('',#2661,.T.);
#1786=FACE_OUTER_BOUND('',#2662,.T.);
#1787=FACE_OUTER_BOUND('',#2663,.T.);
#1788=FACE_OUTER_BOUND('',#2664,.T.);
#1789=FACE_OUTER_BOUND('',#2665,.T.);
#1790=FACE_OUTER_BOUND('',#2666,.T.);
#1791=FACE_OUTER_BOUND('',#2667,.T.);
#1792=FACE_OUTER_BOUND('',#2668,.T.);
#1793=FACE_OUTER_BOUND('',#2669,.T.);
#1794=FACE_OUTER_BOUND('',#2670,.T.);
#1795=FACE_OUTER_BOUND('',#2671,.T.);
#1796=FACE_OUTER_BOUND('',#2672,.T.);
#1797=FACE_OUTER_BOUND('',#2673,.T.);
#1798=FACE_OUTER_BOUND('',#2674,.T.);
#1799=FACE_OUTER_BOUND('',#2675,.T.);
#1800=FACE_OUTER_BOUND('',#2676,.T.);
#1801=FACE_OUTER_BOUND('',#2677,.T.);
#1802=FACE_OUTER_BOUND('',#2679,.T.);
#1803=FACE_OUTER_BOUND('',#2680,.T.);
#1804=FACE_OUTER_BOUND('',#2681,.T.);
#1805=FACE_OUTER_BOUND('',#2682,.T.);
#1806=FACE_OUTER_BOUND('',#2683,.T.);
#1807=FACE_OUTER_BOUND('',#2684,.T.);
#1808=FACE_OUTER_BOUND('',#2685,.T.);
#1809=FACE_OUTER_BOUND('',#2686,.T.);
#1810=FACE_OUTER_BOUND('',#2687,.T.);
#1811=FACE_OUTER_BOUND('',#2688,.T.);
#1812=FACE_OUTER_BOUND('',#2689,.T.);
#1813=FACE_OUTER_BOUND('',#2690,.T.);
#1814=FACE_OUTER_BOUND('',#2691,.T.);
#1815=FACE_OUTER_BOUND('',#2692,.T.);
#1816=FACE_OUTER_BOUND('',#2693,.T.);
#1817=FACE_OUTER_BOUND('',#2694,.T.);
#1818=FACE_OUTER_BOUND('',#2695,.T.);
#1819=FACE_OUTER_BOUND('',#2696,.T.);
#1820=FACE_OUTER_BOUND('',#2697,.T.);
#1821=FACE_OUTER_BOUND('',#2698,.T.);
#1822=FACE_OUTER_BOUND('',#2699,.T.);
#1823=FACE_OUTER_BOUND('',#2700,.T.);
#1824=FACE_OUTER_BOUND('',#2701,.T.);
#1825=FACE_OUTER_BOUND('',#2702,.T.);
#1826=FACE_OUTER_BOUND('',#2703,.T.);
#1827=FACE_OUTER_BOUND('',#2704,.T.);
#1828=FACE_OUTER_BOUND('',#2705,.T.);
#1829=FACE_OUTER_BOUND('',#2706,.T.);
#1830=FACE_OUTER_BOUND('',#2707,.T.);
#1831=FACE_OUTER_BOUND('',#2708,.T.);
#1832=FACE_OUTER_BOUND('',#2709,.T.);
#1833=FACE_OUTER_BOUND('',#2710,.T.);
#1834=FACE_OUTER_BOUND('',#2711,.T.);
#1835=FACE_OUTER_BOUND('',#2712,.T.);
#1836=FACE_OUTER_BOUND('',#2713,.T.);
#1837=FACE_OUTER_BOUND('',#2714,.T.);
#1838=FACE_OUTER_BOUND('',#2715,.T.);
#1839=FACE_OUTER_BOUND('',#2716,.T.);
#1840=FACE_OUTER_BOUND('',#2717,.T.);
#1841=FACE_OUTER_BOUND('',#2718,.T.);
#1842=FACE_OUTER_BOUND('',#2719,.T.);
#1843=FACE_OUTER_BOUND('',#2720,.T.);
#1844=FACE_OUTER_BOUND('',#2721,.T.);
#1845=FACE_OUTER_BOUND('',#2722,.T.);
#1846=FACE_OUTER_BOUND('',#2723,.T.);
#1847=FACE_OUTER_BOUND('',#2724,.T.);
#1848=FACE_OUTER_BOUND('',#2725,.T.);
#1849=FACE_OUTER_BOUND('',#2726,.T.);
#1850=FACE_OUTER_BOUND('',#2727,.T.);
#1851=FACE_OUTER_BOUND('',#2728,.T.);
#1852=FACE_OUTER_BOUND('',#2729,.T.);
#1853=FACE_OUTER_BOUND('',#2730,.T.);
#1854=FACE_OUTER_BOUND('',#2731,.T.);
#1855=FACE_OUTER_BOUND('',#2732,.T.);
#1856=FACE_OUTER_BOUND('',#2733,.T.);
#1857=FACE_OUTER_BOUND('',#2734,.T.);
#1858=FACE_OUTER_BOUND('',#2735,.T.);
#1859=FACE_OUTER_BOUND('',#2736,.T.);
#1860=FACE_OUTER_BOUND('',#2737,.T.);
#1861=FACE_OUTER_BOUND('',#2738,.T.);
#1862=FACE_OUTER_BOUND('',#2739,.T.);
#1863=FACE_OUTER_BOUND('',#2740,.T.);
#1864=FACE_OUTER_BOUND('',#2741,.T.);
#1865=FACE_OUTER_BOUND('',#2742,.T.);
#1866=FACE_OUTER_BOUND('',#2743,.T.);
#1867=FACE_OUTER_BOUND('',#2744,.T.);
#1868=FACE_OUTER_BOUND('',#2745,.T.);
#1869=FACE_OUTER_BOUND('',#2746,.T.);
#1870=FACE_OUTER_BOUND('',#2747,.T.);
#1871=FACE_OUTER_BOUND('',#2748,.T.);
#1872=FACE_OUTER_BOUND('',#2749,.T.);
#1873=FACE_OUTER_BOUND('',#2750,.T.);
#1874=FACE_OUTER_BOUND('',#2751,.T.);
#1875=FACE_OUTER_BOUND('',#2752,.T.);
#1876=FACE_OUTER_BOUND('',#2753,.T.);
#1877=FACE_OUTER_BOUND('',#2754,.T.);
#1878=FACE_OUTER_BOUND('',#2755,.T.);
#1879=FACE_OUTER_BOUND('',#2756,.T.);
#1880=FACE_OUTER_BOUND('',#2757,.T.);
#1881=FACE_OUTER_BOUND('',#2758,.T.);
#1882=FACE_OUTER_BOUND('',#2759,.T.);
#1883=FACE_OUTER_BOUND('',#2760,.T.);
#1884=FACE_OUTER_BOUND('',#2761,.T.);
#1885=FACE_OUTER_BOUND('',#2762,.T.);
#1886=FACE_OUTER_BOUND('',#2763,.T.);
#1887=FACE_OUTER_BOUND('',#2764,.T.);
#1888=FACE_OUTER_BOUND('',#2765,.T.);
#1889=FACE_OUTER_BOUND('',#2766,.T.);
#1890=FACE_OUTER_BOUND('',#2767,.T.);
#1891=FACE_OUTER_BOUND('',#2768,.T.);
#1892=FACE_OUTER_BOUND('',#2769,.T.);
#1893=FACE_OUTER_BOUND('',#2770,.T.);
#1894=FACE_OUTER_BOUND('',#2771,.T.);
#1895=FACE_OUTER_BOUND('',#2772,.T.);
#1896=FACE_OUTER_BOUND('',#2773,.T.);
#1897=FACE_OUTER_BOUND('',#2774,.T.);
#1898=FACE_OUTER_BOUND('',#2775,.T.);
#1899=FACE_OUTER_BOUND('',#2776,.T.);
#1900=FACE_OUTER_BOUND('',#2777,.T.);
#1901=FACE_OUTER_BOUND('',#2778,.T.);
#1902=FACE_OUTER_BOUND('',#2779,.T.);
#1903=FACE_OUTER_BOUND('',#2780,.T.);
#1904=FACE_OUTER_BOUND('',#2781,.T.);
#1905=FACE_OUTER_BOUND('',#2782,.T.);
#1906=FACE_OUTER_BOUND('',#2783,.T.);
#1907=FACE_OUTER_BOUND('',#2785,.T.);
#1908=FACE_OUTER_BOUND('',#2786,.T.);
#2620=EDGE_LOOP('',(#10939,#10940,#10941,#10942));
#2621=EDGE_LOOP('',(#10943,#10944,#10945,#10946));
#2622=EDGE_LOOP('',(#10947,#10948,#10949,#10950));
#2623=EDGE_LOOP('',(#10951,#10952,#10953,#10954));
#2624=EDGE_LOOP('',(#10955,#10956,#10957,#10958));
#2625=EDGE_LOOP('',(#10959,#10960,#10961,#10962));
#2626=EDGE_LOOP('',(#10963,#10964,#10965,#10966));
#2627=EDGE_LOOP('',(#10967,#10968,#10969,#10970));
#2628=EDGE_LOOP('',(#10971,#10972,#10973,#10974));
#2629=EDGE_LOOP('',(#10975,#10976,#10977,#10978));
#2630=EDGE_LOOP('',(#10979,#10980,#10981,#10982));
#2631=EDGE_LOOP('',(#10983,#10984,#10985,#10986));
#2632=EDGE_LOOP('',(#10987,#10988,#10989,#10990));
#2633=EDGE_LOOP('',(#10991,#10992,#10993,#10994));
#2634=EDGE_LOOP('',(#10995,#10996,#10997,#10998));
#2635=EDGE_LOOP('',(#10999,#11000,#11001,#11002));
#2636=EDGE_LOOP('',(#11003,#11004,#11005,#11006));
#2637=EDGE_LOOP('',(#11007,#11008,#11009,#11010));
#2638=EDGE_LOOP('',(#11011,#11012,#11013,#11014));
#2639=EDGE_LOOP('',(#11015,#11016,#11017,#11018));
#2640=EDGE_LOOP('',(#11019,#11020,#11021,#11022));
#2641=EDGE_LOOP('',(#11023,#11024,#11025,#11026));
#2642=EDGE_LOOP('',(#11027,#11028,#11029,#11030));
#2643=EDGE_LOOP('',(#11031,#11032,#11033,#11034));
#2644=EDGE_LOOP('',(#11035,#11036,#11037,#11038));
#2645=EDGE_LOOP('',(#11039,#11040,#11041,#11042));
#2646=EDGE_LOOP('',(#11043,#11044,#11045,#11046));
#2647=EDGE_LOOP('',(#11047,#11048,#11049,#11050));
#2648=EDGE_LOOP('',(#11051,#11052,#11053,#11054));
#2649=EDGE_LOOP('',(#11055,#11056,#11057,#11058));
#2650=EDGE_LOOP('',(#11059,#11060,#11061,#11062));
#2651=EDGE_LOOP('',(#11063,#11064,#11065,#11066));
#2652=EDGE_LOOP('',(#11067,#11068,#11069,#11070));
#2653=EDGE_LOOP('',(#11071,#11072,#11073,#11074));
#2654=EDGE_LOOP('',(#11075,#11076,#11077,#11078));
#2655=EDGE_LOOP('',(#11079,#11080,#11081,#11082));
#2656=EDGE_LOOP('',(#11083,#11084,#11085,#11086));
#2657=EDGE_LOOP('',(#11087,#11088,#11089,#11090));
#2658=EDGE_LOOP('',(#11091,#11092,#11093,#11094));
#2659=EDGE_LOOP('',(#11095,#11096,#11097,#11098));
#2660=EDGE_LOOP('',(#11099,#11100,#11101,#11102));
#2661=EDGE_LOOP('',(#11103,#11104,#11105,#11106));
#2662=EDGE_LOOP('',(#11107,#11108,#11109,#11110));
#2663=EDGE_LOOP('',(#11111,#11112,#11113,#11114));
#2664=EDGE_LOOP('',(#11115,#11116,#11117,#11118));
#2665=EDGE_LOOP('',(#11119,#11120,#11121,#11122));
#2666=EDGE_LOOP('',(#11123,#11124,#11125,#11126));
#2667=EDGE_LOOP('',(#11127,#11128,#11129,#11130));
#2668=EDGE_LOOP('',(#11131,#11132,#11133,#11134));
#2669=EDGE_LOOP('',(#11135,#11136,#11137,#11138));
#2670=EDGE_LOOP('',(#11139,#11140,#11141,#11142));
#2671=EDGE_LOOP('',(#11143,#11144,#11145,#11146));
#2672=EDGE_LOOP('',(#11147,#11148,#11149,#11150));
#2673=EDGE_LOOP('',(#11151,#11152,#11153,#11154));
#2674=EDGE_LOOP('',(#11155,#11156,#11157,#11158));
#2675=EDGE_LOOP('',(#11159,#11160,#11161,#11162,#11163,#11164,#11165,#11166,
#11167,#11168,#11169,#11170,#11171,#11172,#11173,#11174,#11175,#11176,#11177,
#11178,#11179,#11180,#11181,#11182,#11183,#11184,#11185,#11186,#11187,#11188,
#11189,#11190,#11191,#11192,#11193,#11194,#11195,#11196,#11197,#11198,#11199,
#11200,#11201,#11202,#11203,#11204,#11205,#11206,#11207,#11208,#11209,#11210));
#2676=EDGE_LOOP('',(#11211,#11212,#11213,#11214,#11215,#11216,#11217,#11218,
#11219,#11220,#11221,#11222,#11223,#11224,#11225,#11226,#11227,#11228,#11229,
#11230,#11231,#11232,#11233,#11234,#11235,#11236,#11237,#11238,#11239,#11240,
#11241,#11242,#11243,#11244,#11245,#11246,#11247,#11248,#11249,#11250,#11251,
#11252,#11253,#11254,#11255,#11256,#11257,#11258,#11259,#11260,#11261,#11262,
#11263,#11264,#11265,#11266,#11267,#11268,#11269,#11270,#11271,#11272,#11273,
#11274,#11275,#11276,#11277,#11278,#11279,#11280,#11281,#11282,#11283,#11284,
#11285,#11286,#11287,#11288,#11289,#11290,#11291,#11292,#11293,#11294,#11295,
#11296,#11297,#11298,#11299,#11300,#11301,#11302,#11303,#11304,#11305,#11306,
#11307,#11308,#11309,#11310));
#2677=EDGE_LOOP('',(#11311));
#2678=EDGE_LOOP('',(#11312,#11313,#11314,#11315));
#2679=EDGE_LOOP('',(#11316,#11317,#11318,#11319,#11320,#11321,#11322,#11323,
#11324,#11325,#11326,#11327,#11328,#11329,#11330,#11331,#11332,#11333,#11334,
#11335,#11336,#11337,#11338,#11339,#11340,#11341,#11342,#11343,#11344,#11345,
#11346,#11347,#11348,#11349,#11350,#11351,#11352,#11353,#11354,#11355,#11356,
#11357,#11358,#11359,#11360,#11361,#11362,#11363,#11364,#11365,#11366,#11367,
#11368,#11369,#11370,#11371,#11372,#11373,#11374));
#2680=EDGE_LOOP('',(#11375,#11376,#11377,#11378,#11379));
#2681=EDGE_LOOP('',(#11380,#11381,#11382,#11383));
#2682=EDGE_LOOP('',(#11384,#11385,#11386,#11387,#11388,#11389,#11390,#11391,
#11392,#11393,#11394,#11395,#11396,#11397,#11398,#11399,#11400,#11401,#11402,
#11403,#11404,#11405,#11406,#11407,#11408,#11409,#11410,#11411,#11412,#11413,
#11414,#11415,#11416,#11417,#11418,#11419,#11420,#11421,#11422,#11423,#11424,
#11425,#11426,#11427,#11428,#11429,#11430,#11431,#11432,#11433,#11434,#11435,
#11436,#11437,#11438,#11439,#11440,#11441,#11442));
#2683=EDGE_LOOP('',(#11443,#11444,#11445,#11446));
#2684=EDGE_LOOP('',(#11447,#11448,#11449));
#2685=EDGE_LOOP('',(#11450,#11451,#11452,#11453));
#2686=EDGE_LOOP('',(#11454,#11455,#11456));
#2687=EDGE_LOOP('',(#11457,#11458,#11459,#11460));
#2688=EDGE_LOOP('',(#11461,#11462,#11463));
#2689=EDGE_LOOP('',(#11464,#11465,#11466,#11467));
#2690=EDGE_LOOP('',(#11468,#11469,#11470));
#2691=EDGE_LOOP('',(#11471,#11472,#11473,#11474));
#2692=EDGE_LOOP('',(#11475,#11476,#11477));
#2693=EDGE_LOOP('',(#11478,#11479,#11480,#11481));
#2694=EDGE_LOOP('',(#11482,#11483,#11484));
#2695=EDGE_LOOP('',(#11485,#11486,#11487,#11488));
#2696=EDGE_LOOP('',(#11489,#11490,#11491));
#2697=EDGE_LOOP('',(#11492,#11493,#11494,#11495));
#2698=EDGE_LOOP('',(#11496,#11497,#11498));
#2699=EDGE_LOOP('',(#11499,#11500,#11501,#11502));
#2700=EDGE_LOOP('',(#11503,#11504,#11505));
#2701=EDGE_LOOP('',(#11506,#11507,#11508,#11509));
#2702=EDGE_LOOP('',(#11510,#11511,#11512));
#2703=EDGE_LOOP('',(#11513,#11514,#11515,#11516));
#2704=EDGE_LOOP('',(#11517,#11518,#11519));
#2705=EDGE_LOOP('',(#11520,#11521,#11522,#11523));
#2706=EDGE_LOOP('',(#11524,#11525,#11526));
#2707=EDGE_LOOP('',(#11527,#11528,#11529,#11530));
#2708=EDGE_LOOP('',(#11531,#11532,#11533));
#2709=EDGE_LOOP('',(#11534,#11535,#11536,#11537));
#2710=EDGE_LOOP('',(#11538,#11539,#11540));
#2711=EDGE_LOOP('',(#11541,#11542,#11543,#11544));
#2712=EDGE_LOOP('',(#11545,#11546,#11547));
#2713=EDGE_LOOP('',(#11548,#11549,#11550,#11551));
#2714=EDGE_LOOP('',(#11552,#11553,#11554));
#2715=EDGE_LOOP('',(#11555,#11556,#11557,#11558));
#2716=EDGE_LOOP('',(#11559,#11560,#11561));
#2717=EDGE_LOOP('',(#11562,#11563,#11564,#11565));
#2718=EDGE_LOOP('',(#11566,#11567,#11568));
#2719=EDGE_LOOP('',(#11569,#11570,#11571,#11572));
#2720=EDGE_LOOP('',(#11573,#11574,#11575));
#2721=EDGE_LOOP('',(#11576,#11577,#11578,#11579));
#2722=EDGE_LOOP('',(#11580,#11581,#11582));
#2723=EDGE_LOOP('',(#11583,#11584,#11585,#11586));
#2724=EDGE_LOOP('',(#11587,#11588,#11589));
#2725=EDGE_LOOP('',(#11590,#11591,#11592,#11593));
#2726=EDGE_LOOP('',(#11594,#11595,#11596));
#2727=EDGE_LOOP('',(#11597,#11598,#11599,#11600));
#2728=EDGE_LOOP('',(#11601,#11602,#11603));
#2729=EDGE_LOOP('',(#11604,#11605,#11606,#11607));
#2730=EDGE_LOOP('',(#11608,#11609,#11610,#11611));
#2731=EDGE_LOOP('',(#11612,#11613,#11614,#11615));
#2732=EDGE_LOOP('',(#11616,#11617,#11618));
#2733=EDGE_LOOP('',(#11619,#11620,#11621,#11622));
#2734=EDGE_LOOP('',(#11623,#11624,#11625));
#2735=EDGE_LOOP('',(#11626,#11627,#11628,#11629));
#2736=EDGE_LOOP('',(#11630,#11631,#11632));
#2737=EDGE_LOOP('',(#11633,#11634,#11635,#11636));
#2738=EDGE_LOOP('',(#11637,#11638,#11639));
#2739=EDGE_LOOP('',(#11640,#11641,#11642,#11643));
#2740=EDGE_LOOP('',(#11644,#11645,#11646));
#2741=EDGE_LOOP('',(#11647,#11648,#11649,#11650));
#2742=EDGE_LOOP('',(#11651,#11652,#11653));
#2743=EDGE_LOOP('',(#11654,#11655,#11656,#11657));
#2744=EDGE_LOOP('',(#11658,#11659,#11660));
#2745=EDGE_LOOP('',(#11661,#11662,#11663,#11664));
#2746=EDGE_LOOP('',(#11665,#11666,#11667));
#2747=EDGE_LOOP('',(#11668,#11669,#11670,#11671));
#2748=EDGE_LOOP('',(#11672,#11673,#11674));
#2749=EDGE_LOOP('',(#11675,#11676,#11677,#11678));
#2750=EDGE_LOOP('',(#11679,#11680,#11681));
#2751=EDGE_LOOP('',(#11682,#11683,#11684,#11685));
#2752=EDGE_LOOP('',(#11686,#11687,#11688));
#2753=EDGE_LOOP('',(#11689,#11690,#11691,#11692));
#2754=EDGE_LOOP('',(#11693,#11694,#11695));
#2755=EDGE_LOOP('',(#11696,#11697,#11698,#11699));
#2756=EDGE_LOOP('',(#11700,#11701,#11702));
#2757=EDGE_LOOP('',(#11703,#11704,#11705,#11706));
#2758=EDGE_LOOP('',(#11707,#11708,#11709));
#2759=EDGE_LOOP('',(#11710,#11711,#11712,#11713));
#2760=EDGE_LOOP('',(#11714,#11715,#11716));
#2761=EDGE_LOOP('',(#11717,#11718,#11719,#11720));
#2762=EDGE_LOOP('',(#11721,#11722,#11723));
#2763=EDGE_LOOP('',(#11724,#11725,#11726,#11727));
#2764=EDGE_LOOP('',(#11728,#11729,#11730));
#2765=EDGE_LOOP('',(#11731,#11732,#11733,#11734));
#2766=EDGE_LOOP('',(#11735,#11736,#11737));
#2767=EDGE_LOOP('',(#11738,#11739,#11740,#11741));
#2768=EDGE_LOOP('',(#11742,#11743,#11744));
#2769=EDGE_LOOP('',(#11745,#11746,#11747,#11748));
#2770=EDGE_LOOP('',(#11749,#11750,#11751));
#2771=EDGE_LOOP('',(#11752,#11753,#11754,#11755));
#2772=EDGE_LOOP('',(#11756,#11757,#11758));
#2773=EDGE_LOOP('',(#11759,#11760,#11761,#11762));
#2774=EDGE_LOOP('',(#11763,#11764,#11765));
#2775=EDGE_LOOP('',(#11766,#11767,#11768,#11769));
#2776=EDGE_LOOP('',(#11770,#11771,#11772,#11773));
#2777=EDGE_LOOP('',(#11774,#11775,#11776,#11777));
#2778=EDGE_LOOP('',(#11778,#11779,#11780));
#2779=EDGE_LOOP('',(#11781));
#2780=EDGE_LOOP('',(#11782,#11783,#11784,#11785,#11786,#11787));
#2781=EDGE_LOOP('',(#11788,#11789,#11790,#11791));
#2782=EDGE_LOOP('',(#11792,#11793,#11794,#11795));
#2783=EDGE_LOOP('',(#11796));
#2784=EDGE_LOOP('',(#11797));
#2785=EDGE_LOOP('',(#11798,#11799,#11800,#11801));
#2786=EDGE_LOOP('',(#11802));
#3881=LINE('',#21802,#5120);
#3882=LINE('',#21826,#5121);
#3883=LINE('',#21874,#5122);
#3884=LINE('',#21922,#5123);
#3885=LINE('',#21976,#5124);
#3886=LINE('',#22024,#5125);
#3887=LINE('',#22072,#5126);
#3888=LINE('',#22126,#5127);
#3889=LINE('',#22174,#5128);
#3890=LINE('',#22222,#5129);
#3891=LINE('',#22270,#5130);
#3892=LINE('',#22324,#5131);
#3893=LINE('',#22372,#5132);
#3894=LINE('',#22420,#5133);
#3895=LINE('',#22474,#5134);
#3896=LINE('',#22522,#5135);
#3897=LINE('',#22570,#5136);
#3898=LINE('',#22624,#5137);
#3899=LINE('',#22672,#5138);
#3900=LINE('',#22720,#5139);
#3901=LINE('',#22774,#5140);
#3902=LINE('',#22822,#5141);
#3903=LINE('',#22870,#5142);
#3904=LINE('',#22924,#5143);
#3905=LINE('',#22972,#5144);
#3906=LINE('',#23020,#5145);
#3907=LINE('',#23074,#5146);
#3908=LINE('',#23122,#5147);
#3909=LINE('',#23170,#5148);
#3910=LINE('',#23194,#5149);
#3911=LINE('',#23218,#5150);
#3912=LINE('',#23243,#5151);
#3913=LINE('',#23268,#5152);
#3914=LINE('',#23292,#5153);
#3915=LINE('',#23317,#5154);
#3916=LINE('',#23342,#5155);
#3917=LINE('',#23366,#5156);
#3918=LINE('',#23391,#5157);
#3919=LINE('',#23416,#5158);
#3920=LINE('',#23440,#5159);
#3921=LINE('',#23465,#5160);
#3922=LINE('',#23490,#5161);
#3923=LINE('',#23514,#5162);
#3924=LINE('',#23539,#5163);
#3925=LINE('',#23564,#5164);
#3926=LINE('',#23588,#5165);
#3927=LINE('',#23613,#5166);
#3928=LINE('',#23638,#5167);
#3929=LINE('',#23662,#5168);
#3930=LINE('',#23686,#5169);
#3931=LINE('',#23711,#5170);
#3932=LINE('',#23736,#5171);
#3933=LINE('',#23760,#5172);
#3934=LINE('',#23785,#5173);
#3935=LINE('',#23810,#5174);
#3936=LINE('',#23836,#5175);
#3937=LINE('',#23937,#5176);
#3938=LINE('',#23940,#5177);
#3939=LINE('',#23942,#5178);
#3940=LINE('',#23945,#5179);
#3941=LINE('',#23947,#5180);
#3942=LINE('',#23950,#5181);
#3943=LINE('',#23952,#5182);
#3944=LINE('',#23955,#5183);
#3945=LINE('',#23957,#5184);
#3946=LINE('',#23960,#5185);
#3947=LINE('',#23962,#5186);
#3948=LINE('',#23965,#5187);
#3949=LINE('',#23967,#5188);
#3950=LINE('',#23970,#5189);
#3951=LINE('',#23972,#5190);
#3952=LINE('',#23975,#5191);
#3953=LINE('',#23977,#5192);
#3954=LINE('',#23980,#5193);
#3955=LINE('',#23982,#5194);
#3956=LINE('',#23985,#5195);
#3957=LINE('',#23987,#5196);
#3958=LINE('',#23990,#5197);
#3959=LINE('',#23992,#5198);
#3960=LINE('',#23995,#5199);
#3961=LINE('',#23997,#5200);
#3962=LINE('',#24000,#5201);
#3963=LINE('',#24002,#5202);
#3964=LINE('',#24005,#5203);
#3965=LINE('',#24007,#5204);
#3966=LINE('',#24010,#5205);
#3967=LINE('',#24012,#5206);
#3968=LINE('',#24015,#5207);
#3969=LINE('',#24017,#5208);
#3970=LINE('',#24020,#5209);
#3971=LINE('',#24022,#5210);
#3972=LINE('',#24025,#5211);
#3973=LINE('',#24027,#5212);
#3974=LINE('',#24030,#5213);
#3975=LINE('',#24032,#5214);
#3976=LINE('',#24035,#5215);
#3977=LINE('',#24037,#5216);
#3978=LINE('',#24040,#5217);
#3979=LINE('',#24042,#5218);
#3980=LINE('',#24045,#5219);
#3981=LINE('',#24047,#5220);
#3982=LINE('',#24050,#5221);
#3983=LINE('',#24052,#5222);
#3984=LINE('',#24055,#5223);
#3985=LINE('',#24057,#5224);
#3986=LINE('',#25927,#5225);
#3987=LINE('',#25929,#5226);
#3988=LINE('',#25930,#5227);
#3989=LINE('',#25932,#5228);
#3990=LINE('',#25934,#5229);
#3991=LINE('',#25938,#5230);
#3992=LINE('',#25940,#5231);
#3993=LINE('',#25941,#5232);
#3994=LINE('',#25943,#5233);
#3995=LINE('',#25945,#5234);
#3996=LINE('',#25949,#5235);
#3997=LINE('',#25951,#5236);
#3998=LINE('',#25952,#5237);
#3999=LINE('',#25954,#5238);
#4000=LINE('',#25956,#5239);
#4001=LINE('',#25960,#5240);
#4002=LINE('',#25962,#5241);
#4003=LINE('',#25963,#5242);
#4004=LINE('',#25965,#5243);
#4005=LINE('',#25967,#5244);
#4006=LINE('',#25971,#5245);
#4007=LINE('',#25973,#5246);
#4008=LINE('',#25974,#5247);
#4009=LINE('',#25976,#5248);
#4010=LINE('',#25978,#5249);
#4011=LINE('',#25982,#5250);
#4012=LINE('',#25984,#5251);
#4013=LINE('',#25985,#5252);
#4014=LINE('',#25987,#5253);
#4015=LINE('',#25989,#5254);
#4016=LINE('',#25993,#5255);
#4017=LINE('',#25995,#5256);
#4018=LINE('',#25996,#5257);
#4019=LINE('',#25998,#5258);
#4020=LINE('',#26000,#5259);
#4021=LINE('',#26004,#5260);
#4022=LINE('',#26006,#5261);
#4023=LINE('',#26007,#5262);
#4024=LINE('',#26009,#5263);
#4025=LINE('',#26011,#5264);
#4026=LINE('',#26015,#5265);
#4027=LINE('',#26017,#5266);
#4028=LINE('',#26018,#5267);
#4029=LINE('',#26020,#5268);
#4030=LINE('',#26022,#5269);
#4031=LINE('',#26026,#5270);
#4032=LINE('',#26028,#5271);
#4033=LINE('',#26029,#5272);
#4034=LINE('',#26031,#5273);
#4035=LINE('',#26033,#5274);
#4036=LINE('',#26037,#5275);
#4037=LINE('',#26039,#5276);
#4038=LINE('',#26040,#5277);
#4039=LINE('',#26042,#5278);
#4040=LINE('',#26044,#5279);
#4041=LINE('',#26048,#5280);
#4042=LINE('',#26050,#5281);
#4043=LINE('',#26051,#5282);
#4044=LINE('',#26053,#5283);
#4045=LINE('',#26055,#5284);
#4046=LINE('',#26059,#5285);
#4047=LINE('',#26061,#5286);
#4048=LINE('',#26062,#5287);
#4049=LINE('',#26064,#5288);
#4050=LINE('',#26066,#5289);
#4051=LINE('',#26070,#5290);
#4052=LINE('',#26072,#5291);
#4053=LINE('',#26073,#5292);
#4054=LINE('',#26075,#5293);
#4055=LINE('',#26077,#5294);
#4056=LINE('',#26081,#5295);
#4057=LINE('',#26083,#5296);
#4058=LINE('',#26084,#5297);
#4059=LINE('',#26086,#5298);
#4060=LINE('',#26088,#5299);
#4061=LINE('',#26092,#5300);
#4062=LINE('',#26094,#5301);
#4063=LINE('',#26095,#5302);
#4064=LINE('',#26097,#5303);
#4065=LINE('',#26099,#5304);
#4066=LINE('',#26103,#5305);
#4067=LINE('',#26105,#5306);
#4068=LINE('',#26106,#5307);
#4069=LINE('',#26108,#5308);
#4070=LINE('',#26110,#5309);
#4071=LINE('',#26114,#5310);
#4072=LINE('',#26116,#5311);
#4073=LINE('',#26117,#5312);
#4074=LINE('',#26119,#5313);
#4075=LINE('',#26121,#5314);
#4076=LINE('',#26125,#5315);
#4077=LINE('',#26127,#5316);
#4078=LINE('',#26128,#5317);
#4079=LINE('',#26130,#5318);
#4080=LINE('',#26132,#5319);
#4081=LINE('',#26136,#5320);
#4082=LINE('',#26138,#5321);
#4083=LINE('',#26139,#5322);
#4084=LINE('',#26141,#5323);
#4085=LINE('',#26143,#5324);
#4086=LINE('',#26147,#5325);
#4087=LINE('',#26149,#5326);
#4088=LINE('',#26150,#5327);
#4089=LINE('',#26152,#5328);
#4090=LINE('',#26154,#5329);
#4091=LINE('',#26158,#5330);
#4092=LINE('',#26160,#5331);
#4093=LINE('',#26161,#5332);
#4094=LINE('',#26163,#5333);
#4095=LINE('',#26165,#5334);
#4096=LINE('',#26169,#5335);
#4097=LINE('',#26171,#5336);
#4098=LINE('',#26172,#5337);
#4099=LINE('',#26174,#5338);
#4100=LINE('',#26176,#5339);
#4101=LINE('',#26180,#5340);
#4102=LINE('',#26182,#5341);
#4103=LINE('',#26183,#5342);
#4104=LINE('',#26185,#5343);
#4105=LINE('',#26187,#5344);
#4106=LINE('',#26193,#5345);
#4107=LINE('',#26198,#5346);
#4108=LINE('',#26204,#5347);
#5120=VECTOR('',#17851,4.);
#5121=VECTOR('',#17856,4.);
#5122=VECTOR('',#17859,4.);
#5123=VECTOR('',#17862,4.);
#5124=VECTOR('',#17865,4.);
#5125=VECTOR('',#17868,4.);
#5126=VECTOR('',#17871,4.);
#5127=VECTOR('',#17874,4.);
#5128=VECTOR('',#17877,4.);
#5129=VECTOR('',#17880,4.);
#5130=VECTOR('',#17883,4.);
#5131=VECTOR('',#17886,4.);
#5132=VECTOR('',#17889,4.);
#5133=VECTOR('',#17892,4.);
#5134=VECTOR('',#17895,4.);
#5135=VECTOR('',#17898,4.);
#5136=VECTOR('',#17901,4.);
#5137=VECTOR('',#17904,4.);
#5138=VECTOR('',#17907,4.);
#5139=VECTOR('',#17910,4.);
#5140=VECTOR('',#17913,4.);
#5141=VECTOR('',#17916,4.);
#5142=VECTOR('',#17919,4.);
#5143=VECTOR('',#17922,4.);
#5144=VECTOR('',#17925,4.);
#5145=VECTOR('',#17928,4.);
#5146=VECTOR('',#17931,4.);
#5147=VECTOR('',#17934,4.);
#5148=VECTOR('',#17937,3.52375);
#5149=VECTOR('',#17942,3.52375);
#5150=VECTOR('',#17945,3.52375);
#5151=VECTOR('',#17948,3.52375);
#5152=VECTOR('',#17951,3.52375);
#5153=VECTOR('',#17954,3.52375);
#5154=VECTOR('',#17957,3.52375);
#5155=VECTOR('',#17960,3.52375);
#5156=VECTOR('',#17963,3.52375);
#5157=VECTOR('',#17966,3.52375);
#5158=VECTOR('',#17969,3.52375);
#5159=VECTOR('',#17972,3.52375);
#5160=VECTOR('',#17975,3.52375);
#5161=VECTOR('',#17978,3.52375);
#5162=VECTOR('',#17981,3.52375);
#5163=VECTOR('',#17984,3.52375);
#5164=VECTOR('',#17987,3.52375);
#5165=VECTOR('',#17990,3.52375);
#5166=VECTOR('',#17993,3.52375);
#5167=VECTOR('',#17996,3.52375);
#5168=VECTOR('',#17999,3.52375);
#5169=VECTOR('',#18002,3.52375);
#5170=VECTOR('',#18005,3.52375);
#5171=VECTOR('',#18008,3.52375);
#5172=VECTOR('',#18011,3.52375);
#5173=VECTOR('',#18014,3.52375);
#5174=VECTOR('',#18017,3.52375);
#5175=VECTOR('',#18022,4.8);
#5176=VECTOR('',#18125,5.);
#5177=VECTOR('',#18128,10.);
#5178=VECTOR('',#18129,10.);
#5179=VECTOR('',#18132,10.);
#5180=VECTOR('',#18133,10.);
#5181=VECTOR('',#18136,10.);
#5182=VECTOR('',#18137,10.);
#5183=VECTOR('',#18140,10.);
#5184=VECTOR('',#18141,10.);
#5185=VECTOR('',#18144,10.);
#5186=VECTOR('',#18145,10.);
#5187=VECTOR('',#18148,10.);
#5188=VECTOR('',#18149,10.);
#5189=VECTOR('',#18152,10.);
#5190=VECTOR('',#18153,10.);
#5191=VECTOR('',#18156,10.);
#5192=VECTOR('',#18157,10.);
#5193=VECTOR('',#18160,10.);
#5194=VECTOR('',#18161,10.);
#5195=VECTOR('',#18164,10.);
#5196=VECTOR('',#18165,10.);
#5197=VECTOR('',#18168,10.);
#5198=VECTOR('',#18169,10.);
#5199=VECTOR('',#18172,10.);
#5200=VECTOR('',#18173,10.);
#5201=VECTOR('',#18176,10.);
#5202=VECTOR('',#18177,10.);
#5203=VECTOR('',#18180,10.);
#5204=VECTOR('',#18181,10.);
#5205=VECTOR('',#18184,10.);
#5206=VECTOR('',#18185,10.);
#5207=VECTOR('',#18188,10.);
#5208=VECTOR('',#18189,10.);
#5209=VECTOR('',#18192,10.);
#5210=VECTOR('',#18193,10.);
#5211=VECTOR('',#18196,10.);
#5212=VECTOR('',#18197,10.);
#5213=VECTOR('',#18200,10.);
#5214=VECTOR('',#18201,10.);
#5215=VECTOR('',#18204,10.);
#5216=VECTOR('',#18205,10.);
#5217=VECTOR('',#18208,10.);
#5218=VECTOR('',#18209,10.);
#5219=VECTOR('',#18212,10.);
#5220=VECTOR('',#18213,10.);
#5221=VECTOR('',#18216,10.);
#5222=VECTOR('',#18217,10.);
#5223=VECTOR('',#18220,10.);
#5224=VECTOR('',#18221,10.);
#5225=VECTOR('',#18240,10.);
#5226=VECTOR('',#18241,10.);
#5227=VECTOR('',#18242,10.);
#5228=VECTOR('',#18245,10.);
#5229=VECTOR('',#18248,10.);
#5230=VECTOR('',#18253,10.);
#5231=VECTOR('',#18254,10.);
#5232=VECTOR('',#18255,10.);
#5233=VECTOR('',#18258,10.);
#5234=VECTOR('',#18261,10.);
#5235=VECTOR('',#18266,10.);
#5236=VECTOR('',#18267,10.);
#5237=VECTOR('',#18268,10.);
#5238=VECTOR('',#18271,10.);
#5239=VECTOR('',#18274,10.);
#5240=VECTOR('',#18279,10.);
#5241=VECTOR('',#18280,10.);
#5242=VECTOR('',#18281,10.);
#5243=VECTOR('',#18284,10.);
#5244=VECTOR('',#18287,10.);
#5245=VECTOR('',#18292,10.);
#5246=VECTOR('',#18293,10.);
#5247=VECTOR('',#18294,10.);
#5248=VECTOR('',#18297,10.);
#5249=VECTOR('',#18300,10.);
#5250=VECTOR('',#18305,10.);
#5251=VECTOR('',#18306,10.);
#5252=VECTOR('',#18307,10.);
#5253=VECTOR('',#18310,10.);
#5254=VECTOR('',#18313,10.);
#5255=VECTOR('',#18318,10.);
#5256=VECTOR('',#18319,10.);
#5257=VECTOR('',#18320,10.);
#5258=VECTOR('',#18323,10.);
#5259=VECTOR('',#18326,10.);
#5260=VECTOR('',#18331,10.);
#5261=VECTOR('',#18332,10.);
#5262=VECTOR('',#18333,10.);
#5263=VECTOR('',#18336,10.);
#5264=VECTOR('',#18339,10.);
#5265=VECTOR('',#18344,10.);
#5266=VECTOR('',#18345,10.);
#5267=VECTOR('',#18346,10.);
#5268=VECTOR('',#18349,10.);
#5269=VECTOR('',#18352,10.);
#5270=VECTOR('',#18357,10.);
#5271=VECTOR('',#18358,10.);
#5272=VECTOR('',#18359,10.);
#5273=VECTOR('',#18362,10.);
#5274=VECTOR('',#18365,10.);
#5275=VECTOR('',#18370,10.);
#5276=VECTOR('',#18371,10.);
#5277=VECTOR('',#18372,10.);
#5278=VECTOR('',#18375,10.);
#5279=VECTOR('',#18378,10.);
#5280=VECTOR('',#18383,10.);
#5281=VECTOR('',#18384,10.);
#5282=VECTOR('',#18385,10.);
#5283=VECTOR('',#18388,10.);
#5284=VECTOR('',#18391,10.);
#5285=VECTOR('',#18396,10.);
#5286=VECTOR('',#18397,10.);
#5287=VECTOR('',#18398,10.);
#5288=VECTOR('',#18401,10.);
#5289=VECTOR('',#18404,10.);
#5290=VECTOR('',#18409,10.);
#5291=VECTOR('',#18410,10.);
#5292=VECTOR('',#18411,10.);
#5293=VECTOR('',#18414,10.);
#5294=VECTOR('',#18417,10.);
#5295=VECTOR('',#18422,10.);
#5296=VECTOR('',#18423,10.);
#5297=VECTOR('',#18424,10.);
#5298=VECTOR('',#18427,10.);
#5299=VECTOR('',#18430,10.);
#5300=VECTOR('',#18435,10.);
#5301=VECTOR('',#18436,10.);
#5302=VECTOR('',#18437,10.);
#5303=VECTOR('',#18440,10.);
#5304=VECTOR('',#18443,10.);
#5305=VECTOR('',#18448,10.);
#5306=VECTOR('',#18449,10.);
#5307=VECTOR('',#18450,10.);
#5308=VECTOR('',#18453,10.);
#5309=VECTOR('',#18456,10.);
#5310=VECTOR('',#18461,10.);
#5311=VECTOR('',#18462,10.);
#5312=VECTOR('',#18463,10.);
#5313=VECTOR('',#18466,10.);
#5314=VECTOR('',#18469,10.);
#5315=VECTOR('',#18474,10.);
#5316=VECTOR('',#18475,10.);
#5317=VECTOR('',#18476,10.);
#5318=VECTOR('',#18479,10.);
#5319=VECTOR('',#18482,10.);
#5320=VECTOR('',#18487,10.);
#5321=VECTOR('',#18488,10.);
#5322=VECTOR('',#18489,10.);
#5323=VECTOR('',#18492,10.);
#5324=VECTOR('',#18495,10.);
#5325=VECTOR('',#18500,10.);
#5326=VECTOR('',#18501,10.);
#5327=VECTOR('',#18502,10.);
#5328=VECTOR('',#18505,10.);
#5329=VECTOR('',#18508,10.);
#5330=VECTOR('',#18513,10.);
#5331=VECTOR('',#18514,10.);
#5332=VECTOR('',#18515,10.);
#5333=VECTOR('',#18518,10.);
#5334=VECTOR('',#18521,10.);
#5335=VECTOR('',#18526,10.);
#5336=VECTOR('',#18527,10.);
#5337=VECTOR('',#18528,10.);
#5338=VECTOR('',#18531,10.);
#5339=VECTOR('',#18534,10.);
#5340=VECTOR('',#18539,10.);
#5341=VECTOR('',#18540,10.);
#5342=VECTOR('',#18541,10.);
#5343=VECTOR('',#18544,10.);
#5344=VECTOR('',#18547,10.);
#5345=VECTOR('',#18556,3.8);
#5346=VECTOR('',#18563,4.75);
#5347=VECTOR('',#18570,3.);
#6209=VERTEX_POINT('',#21800);
#6210=VERTEX_POINT('',#21801);
#6211=VERTEX_POINT('',#21803);
#6212=VERTEX_POINT('',#21814);
#6213=VERTEX_POINT('',#21824);
#6214=VERTEX_POINT('',#21825);
#6215=VERTEX_POINT('',#21872);
#6216=VERTEX_POINT('',#21873);
#6217=VERTEX_POINT('',#21920);
#6218=VERTEX_POINT('',#21921);
#6219=VERTEX_POINT('',#21974);
#6220=VERTEX_POINT('',#21975);
#6221=VERTEX_POINT('',#22022);
#6222=VERTEX_POINT('',#22023);
#6223=VERTEX_POINT('',#22070);
#6224=VERTEX_POINT('',#22071);
#6225=VERTEX_POINT('',#22124);
#6226=VERTEX_POINT('',#22125);
#6227=VERTEX_POINT('',#22172);
#6228=VERTEX_POINT('',#22173);
#6229=VERTEX_POINT('',#22220);
#6230=VERTEX_POINT('',#22221);
#6231=VERTEX_POINT('',#22268);
#6232=VERTEX_POINT('',#22269);
#6233=VERTEX_POINT('',#22322);
#6234=VERTEX_POINT('',#22323);
#6235=VERTEX_POINT('',#22370);
#6236=VERTEX_POINT('',#22371);
#6237=VERTEX_POINT('',#22418);
#6238=VERTEX_POINT('',#22419);
#6239=VERTEX_POINT('',#22472);
#6240=VERTEX_POINT('',#22473);
#6241=VERTEX_POINT('',#22520);
#6242=VERTEX_POINT('',#22521);
#6243=VERTEX_POINT('',#22568);
#6244=VERTEX_POINT('',#22569);
#6245=VERTEX_POINT('',#22622);
#6246=VERTEX_POINT('',#22623);
#6247=VERTEX_POINT('',#22670);
#6248=VERTEX_POINT('',#22671);
#6249=VERTEX_POINT('',#22718);
#6250=VERTEX_POINT('',#22719);
#6251=VERTEX_POINT('',#22772);
#6252=VERTEX_POINT('',#22773);
#6253=VERTEX_POINT('',#22820);
#6254=VERTEX_POINT('',#22821);
#6255=VERTEX_POINT('',#22868);
#6256=VERTEX_POINT('',#22869);
#6257=VERTEX_POINT('',#22922);
#6258=VERTEX_POINT('',#22923);
#6259=VERTEX_POINT('',#22970);
#6260=VERTEX_POINT('',#22971);
#6261=VERTEX_POINT('',#23018);
#6262=VERTEX_POINT('',#23019);
#6263=VERTEX_POINT('',#23072);
#6264=VERTEX_POINT('',#23073);
#6265=VERTEX_POINT('',#23120);
#6266=VERTEX_POINT('',#23121);
#6267=VERTEX_POINT('',#23168);
#6268=VERTEX_POINT('',#23169);
#6269=VERTEX_POINT('',#23171);
#6270=VERTEX_POINT('',#23181);
#6271=VERTEX_POINT('',#23192);
#6272=VERTEX_POINT('',#23193);
#6273=VERTEX_POINT('',#23216);
#6274=VERTEX_POINT('',#23217);
#6275=VERTEX_POINT('',#23241);
#6276=VERTEX_POINT('',#23242);
#6277=VERTEX_POINT('',#23266);
#6278=VERTEX_POINT('',#23267);
#6279=VERTEX_POINT('',#23290);
#6280=VERTEX_POINT('',#23291);
#6281=VERTEX_POINT('',#23315);
#6282=VERTEX_POINT('',#23316);
#6283=VERTEX_POINT('',#23340);
#6284=VERTEX_POINT('',#23341);
#6285=VERTEX_POINT('',#23364);
#6286=VERTEX_POINT('',#23365);
#6287=VERTEX_POINT('',#23389);
#6288=VERTEX_POINT('',#23390);
#6289=VERTEX_POINT('',#23414);
#6290=VERTEX_POINT('',#23415);
#6291=VERTEX_POINT('',#23438);
#6292=VERTEX_POINT('',#23439);
#6293=VERTEX_POINT('',#23463);
#6294=VERTEX_POINT('',#23464);
#6295=VERTEX_POINT('',#23488);
#6296=VERTEX_POINT('',#23489);
#6297=VERTEX_POINT('',#23512);
#6298=VERTEX_POINT('',#23513);
#6299=VERTEX_POINT('',#23537);
#6300=VERTEX_POINT('',#23538);
#6301=VERTEX_POINT('',#23562);
#6302=VERTEX_POINT('',#23563);
#6303=VERTEX_POINT('',#23586);
#6304=VERTEX_POINT('',#23587);
#6305=VERTEX_POINT('',#23611);
#6306=VERTEX_POINT('',#23612);
#6307=VERTEX_POINT('',#23636);
#6308=VERTEX_POINT('',#23637);
#6309=VERTEX_POINT('',#23660);
#6310=VERTEX_POINT('',#23661);
#6311=VERTEX_POINT('',#23684);
#6312=VERTEX_POINT('',#23685);
#6313=VERTEX_POINT('',#23709);
#6314=VERTEX_POINT('',#23710);
#6315=VERTEX_POINT('',#23734);
#6316=VERTEX_POINT('',#23735);
#6317=VERTEX_POINT('',#23758);
#6318=VERTEX_POINT('',#23759);
#6319=VERTEX_POINT('',#23783);
#6320=VERTEX_POINT('',#23784);
#6321=VERTEX_POINT('',#23808);
#6322=VERTEX_POINT('',#23809);
#6323=VERTEX_POINT('',#23832);
#6324=VERTEX_POINT('',#23833);
#6325=VERTEX_POINT('',#23835);
#6326=VERTEX_POINT('',#23838);
#6327=VERTEX_POINT('',#23840);
#6328=VERTEX_POINT('',#23842);
#6329=VERTEX_POINT('',#23844);
#6330=VERTEX_POINT('',#23846);
#6331=VERTEX_POINT('',#23848);
#6332=VERTEX_POINT('',#23850);
#6333=VERTEX_POINT('',#23852);
#6334=VERTEX_POINT('',#23854);
#6335=VERTEX_POINT('',#23856);
#6336=VERTEX_POINT('',#23858);
#6337=VERTEX_POINT('',#23860);
#6338=VERTEX_POINT('',#23862);
#6339=VERTEX_POINT('',#23864);
#6340=VERTEX_POINT('',#23866);
#6341=VERTEX_POINT('',#23868);
#6342=VERTEX_POINT('',#23870);
#6343=VERTEX_POINT('',#23872);
#6344=VERTEX_POINT('',#23874);
#6345=VERTEX_POINT('',#23876);
#6346=VERTEX_POINT('',#23878);
#6347=VERTEX_POINT('',#23880);
#6348=VERTEX_POINT('',#23882);
#6349=VERTEX_POINT('',#23884);
#6350=VERTEX_POINT('',#23886);
#6351=VERTEX_POINT('',#23888);
#6352=VERTEX_POINT('',#23890);
#6353=VERTEX_POINT('',#23892);
#6354=VERTEX_POINT('',#23894);
#6355=VERTEX_POINT('',#23896);
#6356=VERTEX_POINT('',#23898);
#6357=VERTEX_POINT('',#23900);
#6358=VERTEX_POINT('',#23902);
#6359=VERTEX_POINT('',#23904);
#6360=VERTEX_POINT('',#23906);
#6361=VERTEX_POINT('',#23908);
#6362=VERTEX_POINT('',#23910);
#6363=VERTEX_POINT('',#23912);
#6364=VERTEX_POINT('',#23914);
#6365=VERTEX_POINT('',#23916);
#6366=VERTEX_POINT('',#23918);
#6367=VERTEX_POINT('',#23920);
#6368=VERTEX_POINT('',#23922);
#6369=VERTEX_POINT('',#23924);
#6370=VERTEX_POINT('',#23926);
#6371=VERTEX_POINT('',#23928);
#6372=VERTEX_POINT('',#23930);
#6373=VERTEX_POINT('',#23934);
#6374=VERTEX_POINT('',#23936);
#6375=VERTEX_POINT('',#23938);
#6376=VERTEX_POINT('',#23941);
#6377=VERTEX_POINT('',#23943);
#6378=VERTEX_POINT('',#23946);
#6379=VERTEX_POINT('',#23948);
#6380=VERTEX_POINT('',#23951);
#6381=VERTEX_POINT('',#23953);
#6382=VERTEX_POINT('',#23956);
#6383=VERTEX_POINT('',#23958);
#6384=VERTEX_POINT('',#23961);
#6385=VERTEX_POINT('',#23963);
#6386=VERTEX_POINT('',#23966);
#6387=VERTEX_POINT('',#23968);
#6388=VERTEX_POINT('',#23971);
#6389=VERTEX_POINT('',#23973);
#6390=VERTEX_POINT('',#23976);
#6391=VERTEX_POINT('',#23978);
#6392=VERTEX_POINT('',#23981);
#6393=VERTEX_POINT('',#23983);
#6394=VERTEX_POINT('',#23986);
#6395=VERTEX_POINT('',#23988);
#6396=VERTEX_POINT('',#23991);
#6397=VERTEX_POINT('',#23993);
#6398=VERTEX_POINT('',#23996);
#6399=VERTEX_POINT('',#23998);
#6400=VERTEX_POINT('',#24001);
#6401=VERTEX_POINT('',#24003);
#6402=VERTEX_POINT('',#24006);
#6403=VERTEX_POINT('',#24008);
#6404=VERTEX_POINT('',#24011);
#6405=VERTEX_POINT('',#24013);
#6406=VERTEX_POINT('',#24016);
#6407=VERTEX_POINT('',#24018);
#6408=VERTEX_POINT('',#24021);
#6409=VERTEX_POINT('',#24023);
#6410=VERTEX_POINT('',#24026);
#6411=VERTEX_POINT('',#24028);
#6412=VERTEX_POINT('',#24031);
#6413=VERTEX_POINT('',#24033);
#6414=VERTEX_POINT('',#24036);
#6415=VERTEX_POINT('',#24038);
#6416=VERTEX_POINT('',#24041);
#6417=VERTEX_POINT('',#24043);
#6418=VERTEX_POINT('',#24046);
#6419=VERTEX_POINT('',#24048);
#6420=VERTEX_POINT('',#24051);
#6421=VERTEX_POINT('',#24053);
#6422=VERTEX_POINT('',#24056);
#6423=VERTEX_POINT('',#24060);
#6424=VERTEX_POINT('',#24061);
#6425=VERTEX_POINT('',#24983);
#6426=VERTEX_POINT('',#25091);
#6427=VERTEX_POINT('',#25094);
#6428=VERTEX_POINT('',#25926);
#6429=VERTEX_POINT('',#25928);
#6430=VERTEX_POINT('',#25937);
#6431=VERTEX_POINT('',#25939);
#6432=VERTEX_POINT('',#25948);
#6433=VERTEX_POINT('',#25950);
#6434=VERTEX_POINT('',#25959);
#6435=VERTEX_POINT('',#25961);
#6436=VERTEX_POINT('',#25970);
#6437=VERTEX_POINT('',#25972);
#6438=VERTEX_POINT('',#25981);
#6439=VERTEX_POINT('',#25983);
#6440=VERTEX_POINT('',#25992);
#6441=VERTEX_POINT('',#25994);
#6442=VERTEX_POINT('',#26003);
#6443=VERTEX_POINT('',#26005);
#6444=VERTEX_POINT('',#26014);
#6445=VERTEX_POINT('',#26016);
#6446=VERTEX_POINT('',#26025);
#6447=VERTEX_POINT('',#26027);
#6448=VERTEX_POINT('',#26036);
#6449=VERTEX_POINT('',#26038);
#6450=VERTEX_POINT('',#26047);
#6451=VERTEX_POINT('',#26049);
#6452=VERTEX_POINT('',#26058);
#6453=VERTEX_POINT('',#26060);
#6454=VERTEX_POINT('',#26069);
#6455=VERTEX_POINT('',#26071);
#6456=VERTEX_POINT('',#26080);
#6457=VERTEX_POINT('',#26082);
#6458=VERTEX_POINT('',#26091);
#6459=VERTEX_POINT('',#26093);
#6460=VERTEX_POINT('',#26102);
#6461=VERTEX_POINT('',#26104);
#6462=VERTEX_POINT('',#26113);
#6463=VERTEX_POINT('',#26115);
#6464=VERTEX_POINT('',#26124);
#6465=VERTEX_POINT('',#26126);
#6466=VERTEX_POINT('',#26135);
#6467=VERTEX_POINT('',#26137);
#6468=VERTEX_POINT('',#26146);
#6469=VERTEX_POINT('',#26148);
#6470=VERTEX_POINT('',#26157);
#6471=VERTEX_POINT('',#26159);
#6472=VERTEX_POINT('',#26168);
#6473=VERTEX_POINT('',#26170);
#6474=VERTEX_POINT('',#26179);
#6475=VERTEX_POINT('',#26181);
#6476=VERTEX_POINT('',#26190);
#6477=VERTEX_POINT('',#26196);
#6478=VERTEX_POINT('',#26200);
#6479=VERTEX_POINT('',#26203);
#7911=EDGE_CURVE('',#6209,#6210,#3881,.T.);
#7912=EDGE_CURVE('',#6209,#6211,#141,.T.);
#7913=EDGE_CURVE('',#6211,#6212,#1096,.T.);
#7914=EDGE_CURVE('',#6212,#6210,#142,.T.);
#7915=EDGE_CURVE('',#6213,#6214,#3882,.T.);
#7916=EDGE_CURVE('',#6213,#6209,#143,.T.);
#7917=EDGE_CURVE('',#6210,#6214,#144,.T.);
#7918=EDGE_CURVE('',#6215,#6216,#3883,.T.);
#7919=EDGE_CURVE('',#6215,#6213,#145,.T.);
#7920=EDGE_CURVE('',#6214,#6216,#146,.T.);
#7921=EDGE_CURVE('',#6217,#6218,#3884,.T.);
#7922=EDGE_CURVE('',#6217,#6215,#147,.T.);
#7923=EDGE_CURVE('',#6216,#6218,#148,.T.);
#7924=EDGE_CURVE('',#6219,#6220,#3885,.T.);
#7925=EDGE_CURVE('',#6219,#6217,#149,.T.);
#7926=EDGE_CURVE('',#6218,#6220,#150,.T.);
#7927=EDGE_CURVE('',#6221,#6222,#3886,.T.);
#7928=EDGE_CURVE('',#6221,#6219,#151,.T.);
#7929=EDGE_CURVE('',#6220,#6222,#152,.T.);
#7930=EDGE_CURVE('',#6223,#6224,#3887,.T.);
#7931=EDGE_CURVE('',#6223,#6221,#153,.T.);
#7932=EDGE_CURVE('',#6222,#6224,#154,.T.);
#7933=EDGE_CURVE('',#6225,#6226,#3888,.T.);
#7934=EDGE_CURVE('',#6225,#6223,#155,.T.);
#7935=EDGE_CURVE('',#6224,#6226,#156,.T.);
#7936=EDGE_CURVE('',#6227,#6228,#3889,.T.);
#7937=EDGE_CURVE('',#6227,#6225,#157,.T.);
#7938=EDGE_CURVE('',#6226,#6228,#158,.T.);
#7939=EDGE_CURVE('',#6229,#6230,#3890,.T.);
#7940=EDGE_CURVE('',#6229,#6227,#159,.T.);
#7941=EDGE_CURVE('',#6228,#6230,#160,.T.);
#7942=EDGE_CURVE('',#6231,#6232,#3891,.T.);
#7943=EDGE_CURVE('',#6231,#6229,#161,.T.);
#7944=EDGE_CURVE('',#6230,#6232,#162,.T.);
#7945=EDGE_CURVE('',#6233,#6234,#3892,.T.);
#7946=EDGE_CURVE('',#6233,#6231,#163,.T.);
#7947=EDGE_CURVE('',#6232,#6234,#164,.T.);
#7948=EDGE_CURVE('',#6235,#6236,#3893,.T.);
#7949=EDGE_CURVE('',#6235,#6233,#165,.T.);
#7950=EDGE_CURVE('',#6234,#6236,#166,.T.);
#7951=EDGE_CURVE('',#6237,#6238,#3894,.T.);
#7952=EDGE_CURVE('',#6237,#6235,#167,.T.);
#7953=EDGE_CURVE('',#6236,#6238,#168,.T.);
#7954=EDGE_CURVE('',#6239,#6240,#3895,.T.);
#7955=EDGE_CURVE('',#6239,#6237,#169,.T.);
#7956=EDGE_CURVE('',#6238,#6240,#170,.T.);
#7957=EDGE_CURVE('',#6241,#6242,#3896,.T.);
#7958=EDGE_CURVE('',#6241,#6239,#171,.T.);
#7959=EDGE_CURVE('',#6240,#6242,#172,.T.);
#7960=EDGE_CURVE('',#6243,#6244,#3897,.T.);
#7961=EDGE_CURVE('',#6243,#6241,#173,.T.);
#7962=EDGE_CURVE('',#6242,#6244,#174,.T.);
#7963=EDGE_CURVE('',#6245,#6246,#3898,.T.);
#7964=EDGE_CURVE('',#6245,#6243,#175,.T.);
#7965=EDGE_CURVE('',#6244,#6246,#176,.T.);
#7966=EDGE_CURVE('',#6247,#6248,#3899,.T.);
#7967=EDGE_CURVE('',#6247,#6245,#177,.T.);
#7968=EDGE_CURVE('',#6246,#6248,#178,.T.);
#7969=EDGE_CURVE('',#6249,#6250,#3900,.T.);
#7970=EDGE_CURVE('',#6249,#6247,#179,.T.);
#7971=EDGE_CURVE('',#6248,#6250,#180,.T.);
#7972=EDGE_CURVE('',#6251,#6252,#3901,.T.);
#7973=EDGE_CURVE('',#6251,#6249,#181,.T.);
#7974=EDGE_CURVE('',#6250,#6252,#182,.T.);
#7975=EDGE_CURVE('',#6253,#6254,#3902,.T.);
#7976=EDGE_CURVE('',#6253,#6251,#183,.T.);
#7977=EDGE_CURVE('',#6252,#6254,#184,.T.);
#7978=EDGE_CURVE('',#6255,#6256,#3903,.T.);
#7979=EDGE_CURVE('',#6255,#6253,#185,.T.);
#7980=EDGE_CURVE('',#6254,#6256,#186,.T.);
#7981=EDGE_CURVE('',#6257,#6258,#3904,.T.);
#7982=EDGE_CURVE('',#6257,#6255,#187,.T.);
#7983=EDGE_CURVE('',#6256,#6258,#188,.T.);
#7984=EDGE_CURVE('',#6259,#6260,#3905,.T.);
#7985=EDGE_CURVE('',#6259,#6257,#189,.T.);
#7986=EDGE_CURVE('',#6258,#6260,#190,.T.);
#7987=EDGE_CURVE('',#6261,#6262,#3906,.T.);
#7988=EDGE_CURVE('',#6261,#6259,#191,.T.);
#7989=EDGE_CURVE('',#6260,#6262,#192,.T.);
#7990=EDGE_CURVE('',#6263,#6264,#3907,.T.);
#7991=EDGE_CURVE('',#6263,#6261,#193,.T.);
#7992=EDGE_CURVE('',#6262,#6264,#194,.T.);
#7993=EDGE_CURVE('',#6265,#6266,#3908,.T.);
#7994=EDGE_CURVE('',#6265,#6263,#195,.T.);
#7995=EDGE_CURVE('',#6264,#6266,#196,.T.);
#7996=EDGE_CURVE('',#6267,#6268,#3909,.T.);
#7997=EDGE_CURVE('',#6267,#6269,#197,.T.);
#7998=EDGE_CURVE('',#6270,#6269,#1097,.T.);
#7999=EDGE_CURVE('',#6268,#6270,#198,.T.);
#8000=EDGE_CURVE('',#6271,#6272,#3910,.T.);
#8001=EDGE_CURVE('',#6271,#6267,#199,.T.);
#8002=EDGE_CURVE('',#6272,#6268,#200,.T.);
#8003=EDGE_CURVE('',#6273,#6274,#3911,.T.);
#8004=EDGE_CURVE('',#6273,#6271,#201,.T.);
#8005=EDGE_CURVE('',#6274,#6272,#202,.T.);
#8006=EDGE_CURVE('',#6275,#6276,#3912,.T.);
#8007=EDGE_CURVE('',#6275,#6273,#203,.T.);
#8008=EDGE_CURVE('',#6276,#6274,#204,.T.);
#8009=EDGE_CURVE('',#6277,#6278,#3913,.T.);
#8010=EDGE_CURVE('',#6277,#6275,#205,.T.);
#8011=EDGE_CURVE('',#6278,#6276,#206,.T.);
#8012=EDGE_CURVE('',#6279,#6280,#3914,.T.);
#8013=EDGE_CURVE('',#6279,#6277,#207,.T.);
#8014=EDGE_CURVE('',#6280,#6278,#208,.T.);
#8015=EDGE_CURVE('',#6281,#6282,#3915,.T.);
#8016=EDGE_CURVE('',#6281,#6279,#209,.T.);
#8017=EDGE_CURVE('',#6282,#6280,#210,.T.);
#8018=EDGE_CURVE('',#6283,#6284,#3916,.T.);
#8019=EDGE_CURVE('',#6283,#6281,#211,.T.);
#8020=EDGE_CURVE('',#6284,#6282,#212,.T.);
#8021=EDGE_CURVE('',#6285,#6286,#3917,.T.);
#8022=EDGE_CURVE('',#6285,#6283,#213,.T.);
#8023=EDGE_CURVE('',#6286,#6284,#214,.T.);
#8024=EDGE_CURVE('',#6287,#6288,#3918,.T.);
#8025=EDGE_CURVE('',#6287,#6285,#215,.T.);
#8026=EDGE_CURVE('',#6288,#6286,#216,.T.);
#8027=EDGE_CURVE('',#6289,#6290,#3919,.T.);
#8028=EDGE_CURVE('',#6289,#6287,#217,.T.);
#8029=EDGE_CURVE('',#6290,#6288,#218,.T.);
#8030=EDGE_CURVE('',#6291,#6292,#3920,.T.);
#8031=EDGE_CURVE('',#6291,#6289,#219,.T.);
#8032=EDGE_CURVE('',#6292,#6290,#220,.T.);
#8033=EDGE_CURVE('',#6293,#6294,#3921,.T.);
#8034=EDGE_CURVE('',#6293,#6291,#221,.T.);
#8035=EDGE_CURVE('',#6294,#6292,#222,.T.);
#8036=EDGE_CURVE('',#6295,#6296,#3922,.T.);
#8037=EDGE_CURVE('',#6295,#6293,#223,.T.);
#8038=EDGE_CURVE('',#6296,#6294,#224,.T.);
#8039=EDGE_CURVE('',#6297,#6298,#3923,.T.);
#8040=EDGE_CURVE('',#6297,#6295,#225,.T.);
#8041=EDGE_CURVE('',#6298,#6296,#226,.T.);
#8042=EDGE_CURVE('',#6299,#6300,#3924,.T.);
#8043=EDGE_CURVE('',#6299,#6297,#227,.T.);
#8044=EDGE_CURVE('',#6300,#6298,#228,.T.);
#8045=EDGE_CURVE('',#6301,#6302,#3925,.T.);
#8046=EDGE_CURVE('',#6301,#6299,#229,.T.);
#8047=EDGE_CURVE('',#6302,#6300,#230,.T.);
#8048=EDGE_CURVE('',#6303,#6304,#3926,.T.);
#8049=EDGE_CURVE('',#6303,#6301,#231,.T.);
#8050=EDGE_CURVE('',#6304,#6302,#232,.T.);
#8051=EDGE_CURVE('',#6305,#6306,#3927,.T.);
#8052=EDGE_CURVE('',#6305,#6303,#233,.T.);
#8053=EDGE_CURVE('',#6306,#6304,#234,.T.);
#8054=EDGE_CURVE('',#6307,#6308,#3928,.T.);
#8055=EDGE_CURVE('',#6307,#6305,#235,.T.);
#8056=EDGE_CURVE('',#6308,#6306,#236,.T.);
#8057=EDGE_CURVE('',#6309,#6310,#3929,.T.);
#8058=EDGE_CURVE('',#6309,#6307,#237,.T.);
#8059=EDGE_CURVE('',#6310,#6308,#238,.T.);
#8060=EDGE_CURVE('',#6311,#6312,#3930,.T.);
#8061=EDGE_CURVE('',#6311,#6309,#239,.T.);
#8062=EDGE_CURVE('',#6312,#6310,#240,.T.);
#8063=EDGE_CURVE('',#6313,#6314,#3931,.T.);
#8064=EDGE_CURVE('',#6313,#6311,#241,.T.);
#8065=EDGE_CURVE('',#6314,#6312,#242,.T.);
#8066=EDGE_CURVE('',#6315,#6316,#3932,.T.);
#8067=EDGE_CURVE('',#6315,#6313,#243,.T.);
#8068=EDGE_CURVE('',#6316,#6314,#244,.T.);
#8069=EDGE_CURVE('',#6317,#6318,#3933,.T.);
#8070=EDGE_CURVE('',#6317,#6315,#245,.T.);
#8071=EDGE_CURVE('',#6318,#6316,#246,.T.);
#8072=EDGE_CURVE('',#6319,#6320,#3934,.T.);
#8073=EDGE_CURVE('',#6319,#6317,#247,.T.);
#8074=EDGE_CURVE('',#6320,#6318,#248,.T.);
#8075=EDGE_CURVE('',#6321,#6322,#3935,.T.);
#8076=EDGE_CURVE('',#6321,#6319,#249,.T.);
#8077=EDGE_CURVE('',#6322,#6320,#250,.T.);
#8078=EDGE_CURVE('',#6323,#6324,#1098,.T.);
#8079=EDGE_CURVE('',#6324,#6325,#3936,.T.);
#8080=EDGE_CURVE('',#6325,#6325,#1099,.T.);
#8081=EDGE_CURVE('',#6324,#6326,#1100,.T.);
#8082=EDGE_CURVE('',#6326,#6327,#1101,.T.);
#8083=EDGE_CURVE('',#6327,#6328,#1102,.T.);
#8084=EDGE_CURVE('',#6328,#6329,#1103,.T.);
#8085=EDGE_CURVE('',#6329,#6330,#1104,.T.);
#8086=EDGE_CURVE('',#6330,#6331,#1105,.T.);
#8087=EDGE_CURVE('',#6331,#6332,#1106,.T.);
#8088=EDGE_CURVE('',#6332,#6333,#1107,.T.);
#8089=EDGE_CURVE('',#6333,#6334,#1108,.T.);
#8090=EDGE_CURVE('',#6334,#6335,#1109,.T.);
#8091=EDGE_CURVE('',#6335,#6336,#1110,.T.);
#8092=EDGE_CURVE('',#6336,#6337,#1111,.T.);
#8093=EDGE_CURVE('',#6337,#6338,#1112,.T.);
#8094=EDGE_CURVE('',#6338,#6339,#1113,.T.);
#8095=EDGE_CURVE('',#6339,#6340,#1114,.T.);
#8096=EDGE_CURVE('',#6340,#6341,#1115,.T.);
#8097=EDGE_CURVE('',#6341,#6342,#1116,.T.);
#8098=EDGE_CURVE('',#6342,#6343,#1117,.T.);
#8099=EDGE_CURVE('',#6343,#6344,#1118,.T.);
#8100=EDGE_CURVE('',#6344,#6345,#1119,.T.);
#8101=EDGE_CURVE('',#6345,#6346,#1120,.T.);
#8102=EDGE_CURVE('',#6346,#6347,#1121,.T.);
#8103=EDGE_CURVE('',#6347,#6348,#1122,.T.);
#8104=EDGE_CURVE('',#6348,#6349,#1123,.T.);
#8105=EDGE_CURVE('',#6349,#6350,#1124,.T.);
#8106=EDGE_CURVE('',#6350,#6351,#1125,.T.);
#8107=EDGE_CURVE('',#6351,#6352,#1126,.T.);
#8108=EDGE_CURVE('',#6352,#6353,#1127,.T.);
#8109=EDGE_CURVE('',#6353,#6354,#1128,.T.);
#8110=EDGE_CURVE('',#6354,#6355,#1129,.T.);
#8111=EDGE_CURVE('',#6355,#6356,#1130,.T.);
#8112=EDGE_CURVE('',#6356,#6357,#1131,.T.);
#8113=EDGE_CURVE('',#6357,#6358,#1132,.T.);
#8114=EDGE_CURVE('',#6358,#6359,#1133,.T.);
#8115=EDGE_CURVE('',#6359,#6360,#1134,.T.);
#8116=EDGE_CURVE('',#6360,#6361,#1135,.T.);
#8117=EDGE_CURVE('',#6361,#6362,#1136,.T.);
#8118=EDGE_CURVE('',#6362,#6363,#1137,.T.);
#8119=EDGE_CURVE('',#6363,#6364,#1138,.T.);
#8120=EDGE_CURVE('',#6364,#6365,#1139,.T.);
#8121=EDGE_CURVE('',#6365,#6366,#1140,.T.);
#8122=EDGE_CURVE('',#6366,#6367,#1141,.T.);
#8123=EDGE_CURVE('',#6367,#6368,#1142,.T.);
#8124=EDGE_CURVE('',#6368,#6369,#1143,.T.);
#8125=EDGE_CURVE('',#6369,#6370,#1144,.T.);
#8126=EDGE_CURVE('',#6370,#6371,#1145,.T.);
#8127=EDGE_CURVE('',#6371,#6372,#1146,.T.);
#8128=EDGE_CURVE('',#6372,#6323,#1147,.T.);
#8129=EDGE_CURVE('',#6373,#6373,#1148,.T.);
#8130=EDGE_CURVE('',#6373,#6374,#3937,.T.);
#8131=EDGE_CURVE('',#6374,#6375,#1149,.T.);
#8132=EDGE_CURVE('',#6375,#6349,#3938,.T.);
#8133=EDGE_CURVE('',#6348,#6376,#3939,.T.);
#8134=EDGE_CURVE('',#6376,#6377,#1150,.T.);
#8135=EDGE_CURVE('',#6377,#6347,#3940,.T.);
#8136=EDGE_CURVE('',#6346,#6378,#3941,.T.);
#8137=EDGE_CURVE('',#6378,#6379,#1151,.T.);
#8138=EDGE_CURVE('',#6379,#6345,#3942,.T.);
#8139=EDGE_CURVE('',#6344,#6380,#3943,.T.);
#8140=EDGE_CURVE('',#6380,#6381,#1152,.T.);
#8141=EDGE_CURVE('',#6381,#6343,#3944,.T.);
#8142=EDGE_CURVE('',#6342,#6382,#3945,.T.);
#8143=EDGE_CURVE('',#6382,#6383,#1153,.T.);
#8144=EDGE_CURVE('',#6383,#6341,#3946,.T.);
#8145=EDGE_CURVE('',#6340,#6384,#3947,.T.);
#8146=EDGE_CURVE('',#6384,#6385,#1154,.T.);
#8147=EDGE_CURVE('',#6385,#6339,#3948,.T.);
#8148=EDGE_CURVE('',#6338,#6386,#3949,.T.);
#8149=EDGE_CURVE('',#6386,#6387,#1155,.T.);
#8150=EDGE_CURVE('',#6387,#6337,#3950,.T.);
#8151=EDGE_CURVE('',#6336,#6388,#3951,.T.);
#8152=EDGE_CURVE('',#6388,#6389,#1156,.T.);
#8153=EDGE_CURVE('',#6389,#6335,#3952,.T.);
#8154=EDGE_CURVE('',#6334,#6390,#3953,.T.);
#8155=EDGE_CURVE('',#6390,#6391,#1157,.T.);
#8156=EDGE_CURVE('',#6391,#6333,#3954,.T.);
#8157=EDGE_CURVE('',#6332,#6392,#3955,.T.);
#8158=EDGE_CURVE('',#6392,#6393,#1158,.T.);
#8159=EDGE_CURVE('',#6393,#6331,#3956,.T.);
#8160=EDGE_CURVE('',#6330,#6394,#3957,.T.);
#8161=EDGE_CURVE('',#6394,#6395,#1159,.T.);
#8162=EDGE_CURVE('',#6395,#6329,#3958,.T.);
#8163=EDGE_CURVE('',#6328,#6396,#3959,.T.);
#8164=EDGE_CURVE('',#6396,#6397,#1160,.T.);
#8165=EDGE_CURVE('',#6397,#6327,#3960,.T.);
#8166=EDGE_CURVE('',#6326,#6398,#3961,.T.);
#8167=EDGE_CURVE('',#6398,#6399,#1161,.T.);
#8168=EDGE_CURVE('',#6399,#6323,#3962,.T.);
#8169=EDGE_CURVE('',#6372,#6400,#3963,.T.);
#8170=EDGE_CURVE('',#6400,#6401,#1162,.T.);
#8171=EDGE_CURVE('',#6401,#6371,#3964,.T.);
#8172=EDGE_CURVE('',#6370,#6402,#3965,.T.);
#8173=EDGE_CURVE('',#6402,#6403,#1163,.T.);
#8174=EDGE_CURVE('',#6403,#6369,#3966,.T.);
#8175=EDGE_CURVE('',#6368,#6404,#3967,.T.);
#8176=EDGE_CURVE('',#6404,#6405,#1164,.T.);
#8177=EDGE_CURVE('',#6405,#6367,#3968,.T.);
#8178=EDGE_CURVE('',#6366,#6406,#3969,.T.);
#8179=EDGE_CURVE('',#6406,#6407,#1165,.T.);
#8180=EDGE_CURVE('',#6407,#6365,#3970,.T.);
#8181=EDGE_CURVE('',#6364,#6408,#3971,.T.);
#8182=EDGE_CURVE('',#6408,#6409,#1166,.T.);
#8183=EDGE_CURVE('',#6409,#6363,#3972,.T.);
#8184=EDGE_CURVE('',#6362,#6410,#3973,.T.);
#8185=EDGE_CURVE('',#6410,#6411,#1167,.T.);
#8186=EDGE_CURVE('',#6411,#6361,#3974,.T.);
#8187=EDGE_CURVE('',#6360,#6412,#3975,.T.);
#8188=EDGE_CURVE('',#6412,#6413,#1168,.T.);
#8189=EDGE_CURVE('',#6413,#6359,#3976,.T.);
#8190=EDGE_CURVE('',#6358,#6414,#3977,.T.);
#8191=EDGE_CURVE('',#6414,#6415,#1169,.T.);
#8192=EDGE_CURVE('',#6415,#6357,#3978,.T.);
#8193=EDGE_CURVE('',#6356,#6416,#3979,.T.);
#8194=EDGE_CURVE('',#6416,#6417,#1170,.T.);
#8195=EDGE_CURVE('',#6417,#6355,#3980,.T.);
#8196=EDGE_CURVE('',#6354,#6418,#3981,.T.);
#8197=EDGE_CURVE('',#6418,#6419,#1171,.T.);
#8198=EDGE_CURVE('',#6419,#6353,#3982,.T.);
#8199=EDGE_CURVE('',#6352,#6420,#3983,.T.);
#8200=EDGE_CURVE('',#6420,#6421,#1172,.T.);
#8201=EDGE_CURVE('',#6421,#6351,#3984,.T.);
#8202=EDGE_CURVE('',#6350,#6422,#3985,.T.);
#8203=EDGE_CURVE('',#6422,#6374,#1173,.T.);
#8204=EDGE_CURVE('',#6423,#6424,#1174,.T.);
#8205=EDGE_CURVE('',#6424,#6270,#251,.T.);
#8206=EDGE_CURVE('',#6269,#6423,#252,.T.);
#8207=EDGE_CURVE('',#6266,#6424,#253,.T.);
#8208=EDGE_CURVE('',#6425,#6212,#254,.T.);
#8209=EDGE_CURVE('',#6425,#6322,#255,.T.);
#8210=EDGE_CURVE('',#6212,#6426,#1175,.T.);
#8211=EDGE_CURVE('',#6426,#6211,#1176,.T.);
#8212=EDGE_CURVE('',#6211,#6427,#256,.T.);
#8213=EDGE_CURVE('',#6427,#6425,#1177,.T.);
#8214=EDGE_CURVE('',#6427,#6321,#257,.T.);
#8215=EDGE_CURVE('',#6423,#6265,#258,.T.);
#8216=EDGE_CURVE('',#6397,#6428,#3986,.T.);
#8217=EDGE_CURVE('',#6429,#6428,#3987,.T.);
#8218=EDGE_CURVE('',#6327,#6429,#3988,.T.);
#8219=EDGE_CURVE('',#6429,#6328,#3989,.T.);
#8220=EDGE_CURVE('',#6428,#6396,#3990,.T.);
#8221=EDGE_CURVE('',#6395,#6430,#3991,.T.);
#8222=EDGE_CURVE('',#6431,#6430,#3992,.T.);
#8223=EDGE_CURVE('',#6329,#6431,#3993,.T.);
#8224=EDGE_CURVE('',#6431,#6330,#3994,.T.);
#8225=EDGE_CURVE('',#6430,#6394,#3995,.T.);
#8226=EDGE_CURVE('',#6393,#6432,#3996,.T.);
#8227=EDGE_CURVE('',#6433,#6432,#3997,.T.);
#8228=EDGE_CURVE('',#6331,#6433,#3998,.T.);
#8229=EDGE_CURVE('',#6433,#6332,#3999,.T.);
#8230=EDGE_CURVE('',#6432,#6392,#4000,.T.);
#8231=EDGE_CURVE('',#6391,#6434,#4001,.T.);
#8232=EDGE_CURVE('',#6435,#6434,#4002,.T.);
#8233=EDGE_CURVE('',#6333,#6435,#4003,.T.);
#8234=EDGE_CURVE('',#6435,#6334,#4004,.T.);
#8235=EDGE_CURVE('',#6434,#6390,#4005,.T.);
#8236=EDGE_CURVE('',#6389,#6436,#4006,.T.);
#8237=EDGE_CURVE('',#6437,#6436,#4007,.T.);
#8238=EDGE_CURVE('',#6335,#6437,#4008,.T.);
#8239=EDGE_CURVE('',#6437,#6336,#4009,.T.);
#8240=EDGE_CURVE('',#6436,#6388,#4010,.T.);
#8241=EDGE_CURVE('',#6387,#6438,#4011,.T.);
#8242=EDGE_CURVE('',#6439,#6438,#4012,.T.);
#8243=EDGE_CURVE('',#6337,#6439,#4013,.T.);
#8244=EDGE_CURVE('',#6439,#6338,#4014,.T.);
#8245=EDGE_CURVE('',#6438,#6386,#4015,.T.);
#8246=EDGE_CURVE('',#6385,#6440,#4016,.T.);
#8247=EDGE_CURVE('',#6441,#6440,#4017,.T.);
#8248=EDGE_CURVE('',#6339,#6441,#4018,.T.);
#8249=EDGE_CURVE('',#6441,#6340,#4019,.T.);
#8250=EDGE_CURVE('',#6440,#6384,#4020,.T.);
#8251=EDGE_CURVE('',#6383,#6442,#4021,.T.);
#8252=EDGE_CURVE('',#6443,#6442,#4022,.T.);
#8253=EDGE_CURVE('',#6341,#6443,#4023,.T.);
#8254=EDGE_CURVE('',#6443,#6342,#4024,.T.);
#8255=EDGE_CURVE('',#6442,#6382,#4025,.T.);
#8256=EDGE_CURVE('',#6381,#6444,#4026,.T.);
#8257=EDGE_CURVE('',#6445,#6444,#4027,.T.);
#8258=EDGE_CURVE('',#6343,#6445,#4028,.T.);
#8259=EDGE_CURVE('',#6445,#6344,#4029,.T.);
#8260=EDGE_CURVE('',#6444,#6380,#4030,.T.);
#8261=EDGE_CURVE('',#6379,#6446,#4031,.T.);
#8262=EDGE_CURVE('',#6447,#6446,#4032,.T.);
#8263=EDGE_CURVE('',#6345,#6447,#4033,.T.);
#8264=EDGE_CURVE('',#6447,#6346,#4034,.T.);
#8265=EDGE_CURVE('',#6446,#6378,#4035,.T.);
#8266=EDGE_CURVE('',#6377,#6448,#4036,.T.);
#8267=EDGE_CURVE('',#6449,#6448,#4037,.T.);
#8268=EDGE_CURVE('',#6347,#6449,#4038,.T.);
#8269=EDGE_CURVE('',#6449,#6348,#4039,.T.);
#8270=EDGE_CURVE('',#6448,#6376,#4040,.T.);
#8271=EDGE_CURVE('',#6375,#6450,#4041,.T.);
#8272=EDGE_CURVE('',#6451,#6450,#4042,.T.);
#8273=EDGE_CURVE('',#6349,#6451,#4043,.T.);
#8274=EDGE_CURVE('',#6451,#6350,#4044,.T.);
#8275=EDGE_CURVE('',#6450,#6422,#4045,.T.);
#8276=EDGE_CURVE('',#6421,#6452,#4046,.T.);
#8277=EDGE_CURVE('',#6453,#6452,#4047,.T.);
#8278=EDGE_CURVE('',#6351,#6453,#4048,.T.);
#8279=EDGE_CURVE('',#6453,#6352,#4049,.T.);
#8280=EDGE_CURVE('',#6452,#6420,#4050,.T.);
#8281=EDGE_CURVE('',#6419,#6454,#4051,.T.);
#8282=EDGE_CURVE('',#6455,#6454,#4052,.T.);
#8283=EDGE_CURVE('',#6353,#6455,#4053,.T.);
#8284=EDGE_CURVE('',#6455,#6354,#4054,.T.);
#8285=EDGE_CURVE('',#6454,#6418,#4055,.T.);
#8286=EDGE_CURVE('',#6417,#6456,#4056,.T.);
#8287=EDGE_CURVE('',#6457,#6456,#4057,.T.);
#8288=EDGE_CURVE('',#6355,#6457,#4058,.T.);
#8289=EDGE_CURVE('',#6457,#6356,#4059,.T.);
#8290=EDGE_CURVE('',#6456,#6416,#4060,.T.);
#8291=EDGE_CURVE('',#6415,#6458,#4061,.T.);
#8292=EDGE_CURVE('',#6459,#6458,#4062,.T.);
#8293=EDGE_CURVE('',#6357,#6459,#4063,.T.);
#8294=EDGE_CURVE('',#6459,#6358,#4064,.T.);
#8295=EDGE_CURVE('',#6458,#6414,#4065,.T.);
#8296=EDGE_CURVE('',#6413,#6460,#4066,.T.);
#8297=EDGE_CURVE('',#6461,#6460,#4067,.T.);
#8298=EDGE_CURVE('',#6359,#6461,#4068,.T.);
#8299=EDGE_CURVE('',#6461,#6360,#4069,.T.);
#8300=EDGE_CURVE('',#6460,#6412,#4070,.T.);
#8301=EDGE_CURVE('',#6411,#6462,#4071,.T.);
#8302=EDGE_CURVE('',#6463,#6462,#4072,.T.);
#8303=EDGE_CURVE('',#6361,#6463,#4073,.T.);
#8304=EDGE_CURVE('',#6463,#6362,#4074,.T.);
#8305=EDGE_CURVE('',#6462,#6410,#4075,.T.);
#8306=EDGE_CURVE('',#6409,#6464,#4076,.T.);
#8307=EDGE_CURVE('',#6465,#6464,#4077,.T.);
#8308=EDGE_CURVE('',#6363,#6465,#4078,.T.);
#8309=EDGE_CURVE('',#6465,#6364,#4079,.T.);
#8310=EDGE_CURVE('',#6464,#6408,#4080,.T.);
#8311=EDGE_CURVE('',#6407,#6466,#4081,.T.);
#8312=EDGE_CURVE('',#6467,#6466,#4082,.T.);
#8313=EDGE_CURVE('',#6365,#6467,#4083,.T.);
#8314=EDGE_CURVE('',#6467,#6366,#4084,.T.);
#8315=EDGE_CURVE('',#6466,#6406,#4085,.T.);
#8316=EDGE_CURVE('',#6405,#6468,#4086,.T.);
#8317=EDGE_CURVE('',#6469,#6468,#4087,.T.);
#8318=EDGE_CURVE('',#6367,#6469,#4088,.T.);
#8319=EDGE_CURVE('',#6469,#6368,#4089,.T.);
#8320=EDGE_CURVE('',#6468,#6404,#4090,.T.);
#8321=EDGE_CURVE('',#6403,#6470,#4091,.T.);
#8322=EDGE_CURVE('',#6471,#6470,#4092,.T.);
#8323=EDGE_CURVE('',#6369,#6471,#4093,.T.);
#8324=EDGE_CURVE('',#6471,#6370,#4094,.T.);
#8325=EDGE_CURVE('',#6470,#6402,#4095,.T.);
#8326=EDGE_CURVE('',#6401,#6472,#4096,.T.);
#8327=EDGE_CURVE('',#6473,#6472,#4097,.T.);
#8328=EDGE_CURVE('',#6371,#6473,#4098,.T.);
#8329=EDGE_CURVE('',#6473,#6372,#4099,.T.);
#8330=EDGE_CURVE('',#6472,#6400,#4100,.T.);
#8331=EDGE_CURVE('',#6399,#6474,#4101,.T.);
#8332=EDGE_CURVE('',#6475,#6474,#4102,.T.);
#8333=EDGE_CURVE('',#6323,#6475,#4103,.T.);
#8334=EDGE_CURVE('',#6475,#6326,#4104,.T.);
#8335=EDGE_CURVE('',#6474,#6398,#4105,.T.);
#8336=EDGE_CURVE('',#6476,#6476,#1178,.T.);
#8337=EDGE_CURVE('',#6426,#6476,#4106,.T.);
#8338=EDGE_CURVE('',#6477,#6477,#1179,.T.);
#8339=EDGE_CURVE('',#6477,#6373,#4107,.T.);
#8340=EDGE_CURVE('',#6478,#6478,#1180,.T.);
#8341=EDGE_CURVE('',#6478,#6479,#4108,.T.);
#8342=EDGE_CURVE('',#6479,#6479,#1181,.T.);
#10939=ORIENTED_EDGE('',*,*,#7911,.F.);
#10940=ORIENTED_EDGE('',*,*,#7912,.T.);
#10941=ORIENTED_EDGE('',*,*,#7913,.T.);
#10942=ORIENTED_EDGE('',*,*,#7914,.T.);
#10943=ORIENTED_EDGE('',*,*,#7915,.F.);
#10944=ORIENTED_EDGE('',*,*,#7916,.T.);
#10945=ORIENTED_EDGE('',*,*,#7911,.T.);
#10946=ORIENTED_EDGE('',*,*,#7917,.T.);
#10947=ORIENTED_EDGE('',*,*,#7918,.F.);
#10948=ORIENTED_EDGE('',*,*,#7919,.T.);
#10949=ORIENTED_EDGE('',*,*,#7915,.T.);
#10950=ORIENTED_EDGE('',*,*,#7920,.T.);
#10951=ORIENTED_EDGE('',*,*,#7921,.F.);
#10952=ORIENTED_EDGE('',*,*,#7922,.T.);
#10953=ORIENTED_EDGE('',*,*,#7918,.T.);
#10954=ORIENTED_EDGE('',*,*,#7923,.T.);
#10955=ORIENTED_EDGE('',*,*,#7924,.F.);
#10956=ORIENTED_EDGE('',*,*,#7925,.T.);
#10957=ORIENTED_EDGE('',*,*,#7921,.T.);
#10958=ORIENTED_EDGE('',*,*,#7926,.T.);
#10959=ORIENTED_EDGE('',*,*,#7927,.F.);
#10960=ORIENTED_EDGE('',*,*,#7928,.T.);
#10961=ORIENTED_EDGE('',*,*,#7924,.T.);
#10962=ORIENTED_EDGE('',*,*,#7929,.T.);
#10963=ORIENTED_EDGE('',*,*,#7930,.F.);
#10964=ORIENTED_EDGE('',*,*,#7931,.T.);
#10965=ORIENTED_EDGE('',*,*,#7927,.T.);
#10966=ORIENTED_EDGE('',*,*,#7932,.T.);
#10967=ORIENTED_EDGE('',*,*,#7933,.F.);
#10968=ORIENTED_EDGE('',*,*,#7934,.T.);
#10969=ORIENTED_EDGE('',*,*,#7930,.T.);
#10970=ORIENTED_EDGE('',*,*,#7935,.T.);
#10971=ORIENTED_EDGE('',*,*,#7936,.F.);
#10972=ORIENTED_EDGE('',*,*,#7937,.T.);
#10973=ORIENTED_EDGE('',*,*,#7933,.T.);
#10974=ORIENTED_EDGE('',*,*,#7938,.T.);
#10975=ORIENTED_EDGE('',*,*,#7939,.F.);
#10976=ORIENTED_EDGE('',*,*,#7940,.T.);
#10977=ORIENTED_EDGE('',*,*,#7936,.T.);
#10978=ORIENTED_EDGE('',*,*,#7941,.T.);
#10979=ORIENTED_EDGE('',*,*,#7942,.F.);
#10980=ORIENTED_EDGE('',*,*,#7943,.T.);
#10981=ORIENTED_EDGE('',*,*,#7939,.T.);
#10982=ORIENTED_EDGE('',*,*,#7944,.T.);
#10983=ORIENTED_EDGE('',*,*,#7945,.F.);
#10984=ORIENTED_EDGE('',*,*,#7946,.T.);
#10985=ORIENTED_EDGE('',*,*,#7942,.T.);
#10986=ORIENTED_EDGE('',*,*,#7947,.T.);
#10987=ORIENTED_EDGE('',*,*,#7948,.F.);
#10988=ORIENTED_EDGE('',*,*,#7949,.T.);
#10989=ORIENTED_EDGE('',*,*,#7945,.T.);
#10990=ORIENTED_EDGE('',*,*,#7950,.T.);
#10991=ORIENTED_EDGE('',*,*,#7951,.F.);
#10992=ORIENTED_EDGE('',*,*,#7952,.T.);
#10993=ORIENTED_EDGE('',*,*,#7948,.T.);
#10994=ORIENTED_EDGE('',*,*,#7953,.T.);
#10995=ORIENTED_EDGE('',*,*,#7954,.F.);
#10996=ORIENTED_EDGE('',*,*,#7955,.T.);
#10997=ORIENTED_EDGE('',*,*,#7951,.T.);
#10998=ORIENTED_EDGE('',*,*,#7956,.T.);
#10999=ORIENTED_EDGE('',*,*,#7957,.F.);
#11000=ORIENTED_EDGE('',*,*,#7958,.T.);
#11001=ORIENTED_EDGE('',*,*,#7954,.T.);
#11002=ORIENTED_EDGE('',*,*,#7959,.T.);
#11003=ORIENTED_EDGE('',*,*,#7960,.F.);
#11004=ORIENTED_EDGE('',*,*,#7961,.T.);
#11005=ORIENTED_EDGE('',*,*,#7957,.T.);
#11006=ORIENTED_EDGE('',*,*,#7962,.T.);
#11007=ORIENTED_EDGE('',*,*,#7963,.F.);
#11008=ORIENTED_EDGE('',*,*,#7964,.T.);
#11009=ORIENTED_EDGE('',*,*,#7960,.T.);
#11010=ORIENTED_EDGE('',*,*,#7965,.T.);
#11011=ORIENTED_EDGE('',*,*,#7966,.F.);
#11012=ORIENTED_EDGE('',*,*,#7967,.T.);
#11013=ORIENTED_EDGE('',*,*,#7963,.T.);
#11014=ORIENTED_EDGE('',*,*,#7968,.T.);
#11015=ORIENTED_EDGE('',*,*,#7969,.F.);
#11016=ORIENTED_EDGE('',*,*,#7970,.T.);
#11017=ORIENTED_EDGE('',*,*,#7966,.T.);
#11018=ORIENTED_EDGE('',*,*,#7971,.T.);
#11019=ORIENTED_EDGE('',*,*,#7972,.F.);
#11020=ORIENTED_EDGE('',*,*,#7973,.T.);
#11021=ORIENTED_EDGE('',*,*,#7969,.T.);
#11022=ORIENTED_EDGE('',*,*,#7974,.T.);
#11023=ORIENTED_EDGE('',*,*,#7975,.F.);
#11024=ORIENTED_EDGE('',*,*,#7976,.T.);
#11025=ORIENTED_EDGE('',*,*,#7972,.T.);
#11026=ORIENTED_EDGE('',*,*,#7977,.T.);
#11027=ORIENTED_EDGE('',*,*,#7978,.F.);
#11028=ORIENTED_EDGE('',*,*,#7979,.T.);
#11029=ORIENTED_EDGE('',*,*,#7975,.T.);
#11030=ORIENTED_EDGE('',*,*,#7980,.T.);
#11031=ORIENTED_EDGE('',*,*,#7981,.F.);
#11032=ORIENTED_EDGE('',*,*,#7982,.T.);
#11033=ORIENTED_EDGE('',*,*,#7978,.T.);
#11034=ORIENTED_EDGE('',*,*,#7983,.T.);
#11035=ORIENTED_EDGE('',*,*,#7984,.F.);
#11036=ORIENTED_EDGE('',*,*,#7985,.T.);
#11037=ORIENTED_EDGE('',*,*,#7981,.T.);
#11038=ORIENTED_EDGE('',*,*,#7986,.T.);
#11039=ORIENTED_EDGE('',*,*,#7987,.F.);
#11040=ORIENTED_EDGE('',*,*,#7988,.T.);
#11041=ORIENTED_EDGE('',*,*,#7984,.T.);
#11042=ORIENTED_EDGE('',*,*,#7989,.T.);
#11043=ORIENTED_EDGE('',*,*,#7990,.F.);
#11044=ORIENTED_EDGE('',*,*,#7991,.T.);
#11045=ORIENTED_EDGE('',*,*,#7987,.T.);
#11046=ORIENTED_EDGE('',*,*,#7992,.T.);
#11047=ORIENTED_EDGE('',*,*,#7993,.F.);
#11048=ORIENTED_EDGE('',*,*,#7994,.T.);
#11049=ORIENTED_EDGE('',*,*,#7990,.T.);
#11050=ORIENTED_EDGE('',*,*,#7995,.T.);
#11051=ORIENTED_EDGE('',*,*,#7996,.F.);
#11052=ORIENTED_EDGE('',*,*,#7997,.T.);
#11053=ORIENTED_EDGE('',*,*,#7998,.F.);
#11054=ORIENTED_EDGE('',*,*,#7999,.F.);
#11055=ORIENTED_EDGE('',*,*,#8000,.F.);
#11056=ORIENTED_EDGE('',*,*,#8001,.T.);
#11057=ORIENTED_EDGE('',*,*,#7996,.T.);
#11058=ORIENTED_EDGE('',*,*,#8002,.F.);
#11059=ORIENTED_EDGE('',*,*,#8003,.F.);
#11060=ORIENTED_EDGE('',*,*,#8004,.T.);
#11061=ORIENTED_EDGE('',*,*,#8000,.T.);
#11062=ORIENTED_EDGE('',*,*,#8005,.F.);
#11063=ORIENTED_EDGE('',*,*,#8006,.F.);
#11064=ORIENTED_EDGE('',*,*,#8007,.T.);
#11065=ORIENTED_EDGE('',*,*,#8003,.T.);
#11066=ORIENTED_EDGE('',*,*,#8008,.F.);
#11067=ORIENTED_EDGE('',*,*,#8009,.F.);
#11068=ORIENTED_EDGE('',*,*,#8010,.T.);
#11069=ORIENTED_EDGE('',*,*,#8006,.T.);
#11070=ORIENTED_EDGE('',*,*,#8011,.F.);
#11071=ORIENTED_EDGE('',*,*,#8012,.F.);
#11072=ORIENTED_EDGE('',*,*,#8013,.T.);
#11073=ORIENTED_EDGE('',*,*,#8009,.T.);
#11074=ORIENTED_EDGE('',*,*,#8014,.F.);
#11075=ORIENTED_EDGE('',*,*,#8015,.F.);
#11076=ORIENTED_EDGE('',*,*,#8016,.T.);
#11077=ORIENTED_EDGE('',*,*,#8012,.T.);
#11078=ORIENTED_EDGE('',*,*,#8017,.F.);
#11079=ORIENTED_EDGE('',*,*,#8018,.F.);
#11080=ORIENTED_EDGE('',*,*,#8019,.T.);
#11081=ORIENTED_EDGE('',*,*,#8015,.T.);
#11082=ORIENTED_EDGE('',*,*,#8020,.F.);
#11083=ORIENTED_EDGE('',*,*,#8021,.F.);
#11084=ORIENTED_EDGE('',*,*,#8022,.T.);
#11085=ORIENTED_EDGE('',*,*,#8018,.T.);
#11086=ORIENTED_EDGE('',*,*,#8023,.F.);
#11087=ORIENTED_EDGE('',*,*,#8024,.F.);
#11088=ORIENTED_EDGE('',*,*,#8025,.T.);
#11089=ORIENTED_EDGE('',*,*,#8021,.T.);
#11090=ORIENTED_EDGE('',*,*,#8026,.F.);
#11091=ORIENTED_EDGE('',*,*,#8027,.F.);
#11092=ORIENTED_EDGE('',*,*,#8028,.T.);
#11093=ORIENTED_EDGE('',*,*,#8024,.T.);
#11094=ORIENTED_EDGE('',*,*,#8029,.F.);
#11095=ORIENTED_EDGE('',*,*,#8030,.F.);
#11096=ORIENTED_EDGE('',*,*,#8031,.T.);
#11097=ORIENTED_EDGE('',*,*,#8027,.T.);
#11098=ORIENTED_EDGE('',*,*,#8032,.F.);
#11099=ORIENTED_EDGE('',*,*,#8033,.F.);
#11100=ORIENTED_EDGE('',*,*,#8034,.T.);
#11101=ORIENTED_EDGE('',*,*,#8030,.T.);
#11102=ORIENTED_EDGE('',*,*,#8035,.F.);
#11103=ORIENTED_EDGE('',*,*,#8036,.F.);
#11104=ORIENTED_EDGE('',*,*,#8037,.T.);
#11105=ORIENTED_EDGE('',*,*,#8033,.T.);
#11106=ORIENTED_EDGE('',*,*,#8038,.F.);
#11107=ORIENTED_EDGE('',*,*,#8039,.F.);
#11108=ORIENTED_EDGE('',*,*,#8040,.T.);
#11109=ORIENTED_EDGE('',*,*,#8036,.T.);
#11110=ORIENTED_EDGE('',*,*,#8041,.F.);
#11111=ORIENTED_EDGE('',*,*,#8042,.F.);
#11112=ORIENTED_EDGE('',*,*,#8043,.T.);
#11113=ORIENTED_EDGE('',*,*,#8039,.T.);
#11114=ORIENTED_EDGE('',*,*,#8044,.F.);
#11115=ORIENTED_EDGE('',*,*,#8045,.F.);
#11116=ORIENTED_EDGE('',*,*,#8046,.T.);
#11117=ORIENTED_EDGE('',*,*,#8042,.T.);
#11118=ORIENTED_EDGE('',*,*,#8047,.F.);
#11119=ORIENTED_EDGE('',*,*,#8048,.F.);
#11120=ORIENTED_EDGE('',*,*,#8049,.T.);
#11121=ORIENTED_EDGE('',*,*,#8045,.T.);
#11122=ORIENTED_EDGE('',*,*,#8050,.F.);
#11123=ORIENTED_EDGE('',*,*,#8051,.F.);
#11124=ORIENTED_EDGE('',*,*,#8052,.T.);
#11125=ORIENTED_EDGE('',*,*,#8048,.T.);
#11126=ORIENTED_EDGE('',*,*,#8053,.F.);
#11127=ORIENTED_EDGE('',*,*,#8054,.F.);
#11128=ORIENTED_EDGE('',*,*,#8055,.T.);
#11129=ORIENTED_EDGE('',*,*,#8051,.T.);
#11130=ORIENTED_EDGE('',*,*,#8056,.F.);
#11131=ORIENTED_EDGE('',*,*,#8057,.F.);
#11132=ORIENTED_EDGE('',*,*,#8058,.T.);
#11133=ORIENTED_EDGE('',*,*,#8054,.T.);
#11134=ORIENTED_EDGE('',*,*,#8059,.F.);
#11135=ORIENTED_EDGE('',*,*,#8060,.F.);
#11136=ORIENTED_EDGE('',*,*,#8061,.T.);
#11137=ORIENTED_EDGE('',*,*,#8057,.T.);
#11138=ORIENTED_EDGE('',*,*,#8062,.F.);
#11139=ORIENTED_EDGE('',*,*,#8063,.F.);
#11140=ORIENTED_EDGE('',*,*,#8064,.T.);
#11141=ORIENTED_EDGE('',*,*,#8060,.T.);
#11142=ORIENTED_EDGE('',*,*,#8065,.F.);
#11143=ORIENTED_EDGE('',*,*,#8066,.F.);
#11144=ORIENTED_EDGE('',*,*,#8067,.T.);
#11145=ORIENTED_EDGE('',*,*,#8063,.T.);
#11146=ORIENTED_EDGE('',*,*,#8068,.F.);
#11147=ORIENTED_EDGE('',*,*,#8069,.F.);
#11148=ORIENTED_EDGE('',*,*,#8070,.T.);
#11149=ORIENTED_EDGE('',*,*,#8066,.T.);
#11150=ORIENTED_EDGE('',*,*,#8071,.F.);
#11151=ORIENTED_EDGE('',*,*,#8072,.F.);
#11152=ORIENTED_EDGE('',*,*,#8073,.T.);
#11153=ORIENTED_EDGE('',*,*,#8069,.T.);
#11154=ORIENTED_EDGE('',*,*,#8074,.F.);
#11155=ORIENTED_EDGE('',*,*,#8075,.F.);
#11156=ORIENTED_EDGE('',*,*,#8076,.T.);
#11157=ORIENTED_EDGE('',*,*,#8072,.T.);
#11158=ORIENTED_EDGE('',*,*,#8077,.F.);
#11159=ORIENTED_EDGE('',*,*,#8078,.T.);
#11160=ORIENTED_EDGE('',*,*,#8079,.T.);
#11161=ORIENTED_EDGE('',*,*,#8080,.T.);
#11162=ORIENTED_EDGE('',*,*,#8079,.F.);
#11163=ORIENTED_EDGE('',*,*,#8081,.T.);
#11164=ORIENTED_EDGE('',*,*,#8082,.T.);
#11165=ORIENTED_EDGE('',*,*,#8083,.T.);
#11166=ORIENTED_EDGE('',*,*,#8084,.T.);
#11167=ORIENTED_EDGE('',*,*,#8085,.T.);
#11168=ORIENTED_EDGE('',*,*,#8086,.T.);
#11169=ORIENTED_EDGE('',*,*,#8087,.T.);
#11170=ORIENTED_EDGE('',*,*,#8088,.T.);
#11171=ORIENTED_EDGE('',*,*,#8089,.T.);
#11172=ORIENTED_EDGE('',*,*,#8090,.T.);
#11173=ORIENTED_EDGE('',*,*,#8091,.T.);
#11174=ORIENTED_EDGE('',*,*,#8092,.T.);
#11175=ORIENTED_EDGE('',*,*,#8093,.T.);
#11176=ORIENTED_EDGE('',*,*,#8094,.T.);
#11177=ORIENTED_EDGE('',*,*,#8095,.T.);
#11178=ORIENTED_EDGE('',*,*,#8096,.T.);
#11179=ORIENTED_EDGE('',*,*,#8097,.T.);
#11180=ORIENTED_EDGE('',*,*,#8098,.T.);
#11181=ORIENTED_EDGE('',*,*,#8099,.T.);
#11182=ORIENTED_EDGE('',*,*,#8100,.T.);
#11183=ORIENTED_EDGE('',*,*,#8101,.T.);
#11184=ORIENTED_EDGE('',*,*,#8102,.T.);
#11185=ORIENTED_EDGE('',*,*,#8103,.T.);
#11186=ORIENTED_EDGE('',*,*,#8104,.T.);
#11187=ORIENTED_EDGE('',*,*,#8105,.T.);
#11188=ORIENTED_EDGE('',*,*,#8106,.T.);
#11189=ORIENTED_EDGE('',*,*,#8107,.T.);
#11190=ORIENTED_EDGE('',*,*,#8108,.T.);
#11191=ORIENTED_EDGE('',*,*,#8109,.T.);
#11192=ORIENTED_EDGE('',*,*,#8110,.T.);
#11193=ORIENTED_EDGE('',*,*,#8111,.T.);
#11194=ORIENTED_EDGE('',*,*,#8112,.T.);
#11195=ORIENTED_EDGE('',*,*,#8113,.T.);
#11196=ORIENTED_EDGE('',*,*,#8114,.T.);
#11197=ORIENTED_EDGE('',*,*,#8115,.T.);
#11198=ORIENTED_EDGE('',*,*,#8116,.T.);
#11199=ORIENTED_EDGE('',*,*,#8117,.T.);
#11200=ORIENTED_EDGE('',*,*,#8118,.T.);
#11201=ORIENTED_EDGE('',*,*,#8119,.T.);
#11202=ORIENTED_EDGE('',*,*,#8120,.T.);
#11203=ORIENTED_EDGE('',*,*,#8121,.T.);
#11204=ORIENTED_EDGE('',*,*,#8122,.T.);
#11205=ORIENTED_EDGE('',*,*,#8123,.T.);
#11206=ORIENTED_EDGE('',*,*,#8124,.T.);
#11207=ORIENTED_EDGE('',*,*,#8125,.T.);
#11208=ORIENTED_EDGE('',*,*,#8126,.T.);
#11209=ORIENTED_EDGE('',*,*,#8127,.T.);
#11210=ORIENTED_EDGE('',*,*,#8128,.T.);
#11211=ORIENTED_EDGE('',*,*,#8129,.F.);
#11212=ORIENTED_EDGE('',*,*,#8130,.T.);
#11213=ORIENTED_EDGE('',*,*,#8131,.T.);
#11214=ORIENTED_EDGE('',*,*,#8132,.T.);
#11215=ORIENTED_EDGE('',*,*,#8104,.F.);
#11216=ORIENTED_EDGE('',*,*,#8133,.T.);
#11217=ORIENTED_EDGE('',*,*,#8134,.T.);
#11218=ORIENTED_EDGE('',*,*,#8135,.T.);
#11219=ORIENTED_EDGE('',*,*,#8102,.F.);
#11220=ORIENTED_EDGE('',*,*,#8136,.T.);
#11221=ORIENTED_EDGE('',*,*,#8137,.T.);
#11222=ORIENTED_EDGE('',*,*,#8138,.T.);
#11223=ORIENTED_EDGE('',*,*,#8100,.F.);
#11224=ORIENTED_EDGE('',*,*,#8139,.T.);
#11225=ORIENTED_EDGE('',*,*,#8140,.T.);
#11226=ORIENTED_EDGE('',*,*,#8141,.T.);
#11227=ORIENTED_EDGE('',*,*,#8098,.F.);
#11228=ORIENTED_EDGE('',*,*,#8142,.T.);
#11229=ORIENTED_EDGE('',*,*,#8143,.T.);
#11230=ORIENTED_EDGE('',*,*,#8144,.T.);
#11231=ORIENTED_EDGE('',*,*,#8096,.F.);
#11232=ORIENTED_EDGE('',*,*,#8145,.T.);
#11233=ORIENTED_EDGE('',*,*,#8146,.T.);
#11234=ORIENTED_EDGE('',*,*,#8147,.T.);
#11235=ORIENTED_EDGE('',*,*,#8094,.F.);
#11236=ORIENTED_EDGE('',*,*,#8148,.T.);
#11237=ORIENTED_EDGE('',*,*,#8149,.T.);
#11238=ORIENTED_EDGE('',*,*,#8150,.T.);
#11239=ORIENTED_EDGE('',*,*,#8092,.F.);
#11240=ORIENTED_EDGE('',*,*,#8151,.T.);
#11241=ORIENTED_EDGE('',*,*,#8152,.T.);
#11242=ORIENTED_EDGE('',*,*,#8153,.T.);
#11243=ORIENTED_EDGE('',*,*,#8090,.F.);
#11244=ORIENTED_EDGE('',*,*,#8154,.T.);
#11245=ORIENTED_EDGE('',*,*,#8155,.T.);
#11246=ORIENTED_EDGE('',*,*,#8156,.T.);
#11247=ORIENTED_EDGE('',*,*,#8088,.F.);
#11248=ORIENTED_EDGE('',*,*,#8157,.T.);
#11249=ORIENTED_EDGE('',*,*,#8158,.T.);
#11250=ORIENTED_EDGE('',*,*,#8159,.T.);
#11251=ORIENTED_EDGE('',*,*,#8086,.F.);
#11252=ORIENTED_EDGE('',*,*,#8160,.T.);
#11253=ORIENTED_EDGE('',*,*,#8161,.T.);
#11254=ORIENTED_EDGE('',*,*,#8162,.T.);
#11255=ORIENTED_EDGE('',*,*,#8084,.F.);
#11256=ORIENTED_EDGE('',*,*,#8163,.T.);
#11257=ORIENTED_EDGE('',*,*,#8164,.T.);
#11258=ORIENTED_EDGE('',*,*,#8165,.T.);
#11259=ORIENTED_EDGE('',*,*,#8082,.F.);
#11260=ORIENTED_EDGE('',*,*,#8166,.T.);
#11261=ORIENTED_EDGE('',*,*,#8167,.T.);
#11262=ORIENTED_EDGE('',*,*,#8168,.T.);
#11263=ORIENTED_EDGE('',*,*,#8128,.F.);
#11264=ORIENTED_EDGE('',*,*,#8169,.T.);
#11265=ORIENTED_EDGE('',*,*,#8170,.T.);
#11266=ORIENTED_EDGE('',*,*,#8171,.T.);
#11267=ORIENTED_EDGE('',*,*,#8126,.F.);
#11268=ORIENTED_EDGE('',*,*,#8172,.T.);
#11269=ORIENTED_EDGE('',*,*,#8173,.T.);
#11270=ORIENTED_EDGE('',*,*,#8174,.T.);
#11271=ORIENTED_EDGE('',*,*,#8124,.F.);
#11272=ORIENTED_EDGE('',*,*,#8175,.T.);
#11273=ORIENTED_EDGE('',*,*,#8176,.T.);
#11274=ORIENTED_EDGE('',*,*,#8177,.T.);
#11275=ORIENTED_EDGE('',*,*,#8122,.F.);
#11276=ORIENTED_EDGE('',*,*,#8178,.T.);
#11277=ORIENTED_EDGE('',*,*,#8179,.T.);
#11278=ORIENTED_EDGE('',*,*,#8180,.T.);
#11279=ORIENTED_EDGE('',*,*,#8120,.F.);
#11280=ORIENTED_EDGE('',*,*,#8181,.T.);
#11281=ORIENTED_EDGE('',*,*,#8182,.T.);
#11282=ORIENTED_EDGE('',*,*,#8183,.T.);
#11283=ORIENTED_EDGE('',*,*,#8118,.F.);
#11284=ORIENTED_EDGE('',*,*,#8184,.T.);
#11285=ORIENTED_EDGE('',*,*,#8185,.T.);
#11286=ORIENTED_EDGE('',*,*,#8186,.T.);
#11287=ORIENTED_EDGE('',*,*,#8116,.F.);
#11288=ORIENTED_EDGE('',*,*,#8187,.T.);
#11289=ORIENTED_EDGE('',*,*,#8188,.T.);
#11290=ORIENTED_EDGE('',*,*,#8189,.T.);
#11291=ORIENTED_EDGE('',*,*,#8114,.F.);
#11292=ORIENTED_EDGE('',*,*,#8190,.T.);
#11293=ORIENTED_EDGE('',*,*,#8191,.T.);
#11294=ORIENTED_EDGE('',*,*,#8192,.T.);
#11295=ORIENTED_EDGE('',*,*,#8112,.F.);
#11296=ORIENTED_EDGE('',*,*,#8193,.T.);
#11297=ORIENTED_EDGE('',*,*,#8194,.T.);
#11298=ORIENTED_EDGE('',*,*,#8195,.T.);
#11299=ORIENTED_EDGE('',*,*,#8110,.F.);
#11300=ORIENTED_EDGE('',*,*,#8196,.T.);
#11301=ORIENTED_EDGE('',*,*,#8197,.T.);
#11302=ORIENTED_EDGE('',*,*,#8198,.T.);
#11303=ORIENTED_EDGE('',*,*,#8108,.F.);
#11304=ORIENTED_EDGE('',*,*,#8199,.T.);
#11305=ORIENTED_EDGE('',*,*,#8200,.T.);
#11306=ORIENTED_EDGE('',*,*,#8201,.T.);
#11307=ORIENTED_EDGE('',*,*,#8106,.F.);
#11308=ORIENTED_EDGE('',*,*,#8202,.T.);
#11309=ORIENTED_EDGE('',*,*,#8203,.T.);
#11310=ORIENTED_EDGE('',*,*,#8130,.F.);
#11311=ORIENTED_EDGE('',*,*,#8080,.F.);
#11312=ORIENTED_EDGE('',*,*,#8204,.T.);
#11313=ORIENTED_EDGE('',*,*,#8205,.T.);
#11314=ORIENTED_EDGE('',*,*,#7998,.T.);
#11315=ORIENTED_EDGE('',*,*,#8206,.T.);
#11316=ORIENTED_EDGE('',*,*,#8205,.F.);
#11317=ORIENTED_EDGE('',*,*,#8207,.F.);
#11318=ORIENTED_EDGE('',*,*,#7995,.F.);
#11319=ORIENTED_EDGE('',*,*,#7992,.F.);
#11320=ORIENTED_EDGE('',*,*,#7989,.F.);
#11321=ORIENTED_EDGE('',*,*,#7986,.F.);
#11322=ORIENTED_EDGE('',*,*,#7983,.F.);
#11323=ORIENTED_EDGE('',*,*,#7980,.F.);
#11324=ORIENTED_EDGE('',*,*,#7977,.F.);
#11325=ORIENTED_EDGE('',*,*,#7974,.F.);
#11326=ORIENTED_EDGE('',*,*,#7971,.F.);
#11327=ORIENTED_EDGE('',*,*,#7968,.F.);
#11328=ORIENTED_EDGE('',*,*,#7965,.F.);
#11329=ORIENTED_EDGE('',*,*,#7962,.F.);
#11330=ORIENTED_EDGE('',*,*,#7959,.F.);
#11331=ORIENTED_EDGE('',*,*,#7956,.F.);
#11332=ORIENTED_EDGE('',*,*,#7953,.F.);
#11333=ORIENTED_EDGE('',*,*,#7950,.F.);
#11334=ORIENTED_EDGE('',*,*,#7947,.F.);
#11335=ORIENTED_EDGE('',*,*,#7944,.F.);
#11336=ORIENTED_EDGE('',*,*,#7941,.F.);
#11337=ORIENTED_EDGE('',*,*,#7938,.F.);
#11338=ORIENTED_EDGE('',*,*,#7935,.F.);
#11339=ORIENTED_EDGE('',*,*,#7932,.F.);
#11340=ORIENTED_EDGE('',*,*,#7929,.F.);
#11341=ORIENTED_EDGE('',*,*,#7926,.F.);
#11342=ORIENTED_EDGE('',*,*,#7923,.F.);
#11343=ORIENTED_EDGE('',*,*,#7920,.F.);
#11344=ORIENTED_EDGE('',*,*,#7917,.F.);
#11345=ORIENTED_EDGE('',*,*,#7914,.F.);
#11346=ORIENTED_EDGE('',*,*,#8208,.F.);
#11347=ORIENTED_EDGE('',*,*,#8209,.T.);
#11348=ORIENTED_EDGE('',*,*,#8077,.T.);
#11349=ORIENTED_EDGE('',*,*,#8074,.T.);
#11350=ORIENTED_EDGE('',*,*,#8071,.T.);
#11351=ORIENTED_EDGE('',*,*,#8068,.T.);
#11352=ORIENTED_EDGE('',*,*,#8065,.T.);
#11353=ORIENTED_EDGE('',*,*,#8062,.T.);
#11354=ORIENTED_EDGE('',*,*,#8059,.T.);
#11355=ORIENTED_EDGE('',*,*,#8056,.T.);
#11356=ORIENTED_EDGE('',*,*,#8053,.T.);
#11357=ORIENTED_EDGE('',*,*,#8050,.T.);
#11358=ORIENTED_EDGE('',*,*,#8047,.T.);
#11359=ORIENTED_EDGE('',*,*,#8044,.T.);
#11360=ORIENTED_EDGE('',*,*,#8041,.T.);
#11361=ORIENTED_EDGE('',*,*,#8038,.T.);
#11362=ORIENTED_EDGE('',*,*,#8035,.T.);
#11363=ORIENTED_EDGE('',*,*,#8032,.T.);
#11364=ORIENTED_EDGE('',*,*,#8029,.T.);
#11365=ORIENTED_EDGE('',*,*,#8026,.T.);
#11366=ORIENTED_EDGE('',*,*,#8023,.T.);
#11367=ORIENTED_EDGE('',*,*,#8020,.T.);
#11368=ORIENTED_EDGE('',*,*,#8017,.T.);
#11369=ORIENTED_EDGE('',*,*,#8014,.T.);
#11370=ORIENTED_EDGE('',*,*,#8011,.T.);
#11371=ORIENTED_EDGE('',*,*,#8008,.T.);
#11372=ORIENTED_EDGE('',*,*,#8005,.T.);
#11373=ORIENTED_EDGE('',*,*,#8002,.T.);
#11374=ORIENTED_EDGE('',*,*,#7999,.T.);
#11375=ORIENTED_EDGE('',*,*,#8210,.T.);
#11376=ORIENTED_EDGE('',*,*,#8211,.T.);
#11377=ORIENTED_EDGE('',*,*,#8212,.T.);
#11378=ORIENTED_EDGE('',*,*,#8213,.T.);
#11379=ORIENTED_EDGE('',*,*,#8208,.T.);
#11380=ORIENTED_EDGE('',*,*,#8075,.T.);
#11381=ORIENTED_EDGE('',*,*,#8209,.F.);
#11382=ORIENTED_EDGE('',*,*,#8213,.F.);
#11383=ORIENTED_EDGE('',*,*,#8214,.T.);
#11384=ORIENTED_EDGE('',*,*,#8206,.F.);
#11385=ORIENTED_EDGE('',*,*,#7997,.F.);
#11386=ORIENTED_EDGE('',*,*,#8001,.F.);
#11387=ORIENTED_EDGE('',*,*,#8004,.F.);
#11388=ORIENTED_EDGE('',*,*,#8007,.F.);
#11389=ORIENTED_EDGE('',*,*,#8010,.F.);
#11390=ORIENTED_EDGE('',*,*,#8013,.F.);
#11391=ORIENTED_EDGE('',*,*,#8016,.F.);
#11392=ORIENTED_EDGE('',*,*,#8019,.F.);
#11393=ORIENTED_EDGE('',*,*,#8022,.F.);
#11394=ORIENTED_EDGE('',*,*,#8025,.F.);
#11395=ORIENTED_EDGE('',*,*,#8028,.F.);
#11396=ORIENTED_EDGE('',*,*,#8031,.F.);
#11397=ORIENTED_EDGE('',*,*,#8034,.F.);
#11398=ORIENTED_EDGE('',*,*,#8037,.F.);
#11399=ORIENTED_EDGE('',*,*,#8040,.F.);
#11400=ORIENTED_EDGE('',*,*,#8043,.F.);
#11401=ORIENTED_EDGE('',*,*,#8046,.F.);
#11402=ORIENTED_EDGE('',*,*,#8049,.F.);
#11403=ORIENTED_EDGE('',*,*,#8052,.F.);
#11404=ORIENTED_EDGE('',*,*,#8055,.F.);
#11405=ORIENTED_EDGE('',*,*,#8058,.F.);
#11406=ORIENTED_EDGE('',*,*,#8061,.F.);
#11407=ORIENTED_EDGE('',*,*,#8064,.F.);
#11408=ORIENTED_EDGE('',*,*,#8067,.F.);
#11409=ORIENTED_EDGE('',*,*,#8070,.F.);
#11410=ORIENTED_EDGE('',*,*,#8073,.F.);
#11411=ORIENTED_EDGE('',*,*,#8076,.F.);
#11412=ORIENTED_EDGE('',*,*,#8214,.F.);
#11413=ORIENTED_EDGE('',*,*,#8212,.F.);
#11414=ORIENTED_EDGE('',*,*,#7912,.F.);
#11415=ORIENTED_EDGE('',*,*,#7916,.F.);
#11416=ORIENTED_EDGE('',*,*,#7919,.F.);
#11417=ORIENTED_EDGE('',*,*,#7922,.F.);
#11418=ORIENTED_EDGE('',*,*,#7925,.F.);
#11419=ORIENTED_EDGE('',*,*,#7928,.F.);
#11420=ORIENTED_EDGE('',*,*,#7931,.F.);
#11421=ORIENTED_EDGE('',*,*,#7934,.F.);
#11422=ORIENTED_EDGE('',*,*,#7937,.F.);
#11423=ORIENTED_EDGE('',*,*,#7940,.F.);
#11424=ORIENTED_EDGE('',*,*,#7943,.F.);
#11425=ORIENTED_EDGE('',*,*,#7946,.F.);
#11426=ORIENTED_EDGE('',*,*,#7949,.F.);
#11427=ORIENTED_EDGE('',*,*,#7952,.F.);
#11428=ORIENTED_EDGE('',*,*,#7955,.F.);
#11429=ORIENTED_EDGE('',*,*,#7958,.F.);
#11430=ORIENTED_EDGE('',*,*,#7961,.F.);
#11431=ORIENTED_EDGE('',*,*,#7964,.F.);
#11432=ORIENTED_EDGE('',*,*,#7967,.F.);
#11433=ORIENTED_EDGE('',*,*,#7970,.F.);
#11434=ORIENTED_EDGE('',*,*,#7973,.F.);
#11435=ORIENTED_EDGE('',*,*,#7976,.F.);
#11436=ORIENTED_EDGE('',*,*,#7979,.F.);
#11437=ORIENTED_EDGE('',*,*,#7982,.F.);
#11438=ORIENTED_EDGE('',*,*,#7985,.F.);
#11439=ORIENTED_EDGE('',*,*,#7988,.F.);
#11440=ORIENTED_EDGE('',*,*,#7991,.F.);
#11441=ORIENTED_EDGE('',*,*,#7994,.F.);
#11442=ORIENTED_EDGE('',*,*,#8215,.F.);
#11443=ORIENTED_EDGE('',*,*,#8165,.F.);
#11444=ORIENTED_EDGE('',*,*,#8216,.T.);
#11445=ORIENTED_EDGE('',*,*,#8217,.F.);
#11446=ORIENTED_EDGE('',*,*,#8218,.F.);
#11447=ORIENTED_EDGE('',*,*,#8083,.F.);
#11448=ORIENTED_EDGE('',*,*,#8218,.T.);
#11449=ORIENTED_EDGE('',*,*,#8219,.T.);
#11450=ORIENTED_EDGE('',*,*,#8163,.F.);
#11451=ORIENTED_EDGE('',*,*,#8219,.F.);
#11452=ORIENTED_EDGE('',*,*,#8217,.T.);
#11453=ORIENTED_EDGE('',*,*,#8220,.T.);
#11454=ORIENTED_EDGE('',*,*,#8164,.F.);
#11455=ORIENTED_EDGE('',*,*,#8220,.F.);
#11456=ORIENTED_EDGE('',*,*,#8216,.F.);
#11457=ORIENTED_EDGE('',*,*,#8162,.F.);
#11458=ORIENTED_EDGE('',*,*,#8221,.T.);
#11459=ORIENTED_EDGE('',*,*,#8222,.F.);
#11460=ORIENTED_EDGE('',*,*,#8223,.F.);
#11461=ORIENTED_EDGE('',*,*,#8085,.F.);
#11462=ORIENTED_EDGE('',*,*,#8223,.T.);
#11463=ORIENTED_EDGE('',*,*,#8224,.T.);
#11464=ORIENTED_EDGE('',*,*,#8160,.F.);
#11465=ORIENTED_EDGE('',*,*,#8224,.F.);
#11466=ORIENTED_EDGE('',*,*,#8222,.T.);
#11467=ORIENTED_EDGE('',*,*,#8225,.T.);
#11468=ORIENTED_EDGE('',*,*,#8161,.F.);
#11469=ORIENTED_EDGE('',*,*,#8225,.F.);
#11470=ORIENTED_EDGE('',*,*,#8221,.F.);
#11471=ORIENTED_EDGE('',*,*,#8159,.F.);
#11472=ORIENTED_EDGE('',*,*,#8226,.T.);
#11473=ORIENTED_EDGE('',*,*,#8227,.F.);
#11474=ORIENTED_EDGE('',*,*,#8228,.F.);
#11475=ORIENTED_EDGE('',*,*,#8087,.F.);
#11476=ORIENTED_EDGE('',*,*,#8228,.T.);
#11477=ORIENTED_EDGE('',*,*,#8229,.T.);
#11478=ORIENTED_EDGE('',*,*,#8157,.F.);
#11479=ORIENTED_EDGE('',*,*,#8229,.F.);
#11480=ORIENTED_EDGE('',*,*,#8227,.T.);
#11481=ORIENTED_EDGE('',*,*,#8230,.T.);
#11482=ORIENTED_EDGE('',*,*,#8158,.F.);
#11483=ORIENTED_EDGE('',*,*,#8230,.F.);
#11484=ORIENTED_EDGE('',*,*,#8226,.F.);
#11485=ORIENTED_EDGE('',*,*,#8156,.F.);
#11486=ORIENTED_EDGE('',*,*,#8231,.T.);
#11487=ORIENTED_EDGE('',*,*,#8232,.F.);
#11488=ORIENTED_EDGE('',*,*,#8233,.F.);
#11489=ORIENTED_EDGE('',*,*,#8089,.F.);
#11490=ORIENTED_EDGE('',*,*,#8233,.T.);
#11491=ORIENTED_EDGE('',*,*,#8234,.T.);
#11492=ORIENTED_EDGE('',*,*,#8154,.F.);
#11493=ORIENTED_EDGE('',*,*,#8234,.F.);
#11494=ORIENTED_EDGE('',*,*,#8232,.T.);
#11495=ORIENTED_EDGE('',*,*,#8235,.T.);
#11496=ORIENTED_EDGE('',*,*,#8155,.F.);
#11497=ORIENTED_EDGE('',*,*,#8235,.F.);
#11498=ORIENTED_EDGE('',*,*,#8231,.F.);
#11499=ORIENTED_EDGE('',*,*,#8153,.F.);
#11500=ORIENTED_EDGE('',*,*,#8236,.T.);
#11501=ORIENTED_EDGE('',*,*,#8237,.F.);
#11502=ORIENTED_EDGE('',*,*,#8238,.F.);
#11503=ORIENTED_EDGE('',*,*,#8091,.F.);
#11504=ORIENTED_EDGE('',*,*,#8238,.T.);
#11505=ORIENTED_EDGE('',*,*,#8239,.T.);
#11506=ORIENTED_EDGE('',*,*,#8151,.F.);
#11507=ORIENTED_EDGE('',*,*,#8239,.F.);
#11508=ORIENTED_EDGE('',*,*,#8237,.T.);
#11509=ORIENTED_EDGE('',*,*,#8240,.T.);
#11510=ORIENTED_EDGE('',*,*,#8152,.F.);
#11511=ORIENTED_EDGE('',*,*,#8240,.F.);
#11512=ORIENTED_EDGE('',*,*,#8236,.F.);
#11513=ORIENTED_EDGE('',*,*,#8150,.F.);
#11514=ORIENTED_EDGE('',*,*,#8241,.T.);
#11515=ORIENTED_EDGE('',*,*,#8242,.F.);
#11516=ORIENTED_EDGE('',*,*,#8243,.F.);
#11517=ORIENTED_EDGE('',*,*,#8093,.F.);
#11518=ORIENTED_EDGE('',*,*,#8243,.T.);
#11519=ORIENTED_EDGE('',*,*,#8244,.T.);
#11520=ORIENTED_EDGE('',*,*,#8148,.F.);
#11521=ORIENTED_EDGE('',*,*,#8244,.F.);
#11522=ORIENTED_EDGE('',*,*,#8242,.T.);
#11523=ORIENTED_EDGE('',*,*,#8245,.T.);
#11524=ORIENTED_EDGE('',*,*,#8149,.F.);
#11525=ORIENTED_EDGE('',*,*,#8245,.F.);
#11526=ORIENTED_EDGE('',*,*,#8241,.F.);
#11527=ORIENTED_EDGE('',*,*,#8147,.F.);
#11528=ORIENTED_EDGE('',*,*,#8246,.T.);
#11529=ORIENTED_EDGE('',*,*,#8247,.F.);
#11530=ORIENTED_EDGE('',*,*,#8248,.F.);
#11531=ORIENTED_EDGE('',*,*,#8095,.F.);
#11532=ORIENTED_EDGE('',*,*,#8248,.T.);
#11533=ORIENTED_EDGE('',*,*,#8249,.T.);
#11534=ORIENTED_EDGE('',*,*,#8145,.F.);
#11535=ORIENTED_EDGE('',*,*,#8249,.F.);
#11536=ORIENTED_EDGE('',*,*,#8247,.T.);
#11537=ORIENTED_EDGE('',*,*,#8250,.T.);
#11538=ORIENTED_EDGE('',*,*,#8146,.F.);
#11539=ORIENTED_EDGE('',*,*,#8250,.F.);
#11540=ORIENTED_EDGE('',*,*,#8246,.F.);
#11541=ORIENTED_EDGE('',*,*,#8144,.F.);
#11542=ORIENTED_EDGE('',*,*,#8251,.T.);
#11543=ORIENTED_EDGE('',*,*,#8252,.F.);
#11544=ORIENTED_EDGE('',*,*,#8253,.F.);
#11545=ORIENTED_EDGE('',*,*,#8097,.F.);
#11546=ORIENTED_EDGE('',*,*,#8253,.T.);
#11547=ORIENTED_EDGE('',*,*,#8254,.T.);
#11548=ORIENTED_EDGE('',*,*,#8142,.F.);
#11549=ORIENTED_EDGE('',*,*,#8254,.F.);
#11550=ORIENTED_EDGE('',*,*,#8252,.T.);
#11551=ORIENTED_EDGE('',*,*,#8255,.T.);
#11552=ORIENTED_EDGE('',*,*,#8143,.F.);
#11553=ORIENTED_EDGE('',*,*,#8255,.F.);
#11554=ORIENTED_EDGE('',*,*,#8251,.F.);
#11555=ORIENTED_EDGE('',*,*,#8141,.F.);
#11556=ORIENTED_EDGE('',*,*,#8256,.T.);
#11557=ORIENTED_EDGE('',*,*,#8257,.F.);
#11558=ORIENTED_EDGE('',*,*,#8258,.F.);
#11559=ORIENTED_EDGE('',*,*,#8099,.F.);
#11560=ORIENTED_EDGE('',*,*,#8258,.T.);
#11561=ORIENTED_EDGE('',*,*,#8259,.T.);
#11562=ORIENTED_EDGE('',*,*,#8139,.F.);
#11563=ORIENTED_EDGE('',*,*,#8259,.F.);
#11564=ORIENTED_EDGE('',*,*,#8257,.T.);
#11565=ORIENTED_EDGE('',*,*,#8260,.T.);
#11566=ORIENTED_EDGE('',*,*,#8140,.F.);
#11567=ORIENTED_EDGE('',*,*,#8260,.F.);
#11568=ORIENTED_EDGE('',*,*,#8256,.F.);
#11569=ORIENTED_EDGE('',*,*,#8138,.F.);
#11570=ORIENTED_EDGE('',*,*,#8261,.T.);
#11571=ORIENTED_EDGE('',*,*,#8262,.F.);
#11572=ORIENTED_EDGE('',*,*,#8263,.F.);
#11573=ORIENTED_EDGE('',*,*,#8101,.F.);
#11574=ORIENTED_EDGE('',*,*,#8263,.T.);
#11575=ORIENTED_EDGE('',*,*,#8264,.T.);
#11576=ORIENTED_EDGE('',*,*,#8136,.F.);
#11577=ORIENTED_EDGE('',*,*,#8264,.F.);
#11578=ORIENTED_EDGE('',*,*,#8262,.T.);
#11579=ORIENTED_EDGE('',*,*,#8265,.T.);
#11580=ORIENTED_EDGE('',*,*,#8137,.F.);
#11581=ORIENTED_EDGE('',*,*,#8265,.F.);
#11582=ORIENTED_EDGE('',*,*,#8261,.F.);
#11583=ORIENTED_EDGE('',*,*,#8135,.F.);
#11584=ORIENTED_EDGE('',*,*,#8266,.T.);
#11585=ORIENTED_EDGE('',*,*,#8267,.F.);
#11586=ORIENTED_EDGE('',*,*,#8268,.F.);
#11587=ORIENTED_EDGE('',*,*,#8103,.F.);
#11588=ORIENTED_EDGE('',*,*,#8268,.T.);
#11589=ORIENTED_EDGE('',*,*,#8269,.T.);
#11590=ORIENTED_EDGE('',*,*,#8133,.F.);
#11591=ORIENTED_EDGE('',*,*,#8269,.F.);
#11592=ORIENTED_EDGE('',*,*,#8267,.T.);
#11593=ORIENTED_EDGE('',*,*,#8270,.T.);
#11594=ORIENTED_EDGE('',*,*,#8134,.F.);
#11595=ORIENTED_EDGE('',*,*,#8270,.F.);
#11596=ORIENTED_EDGE('',*,*,#8266,.F.);
#11597=ORIENTED_EDGE('',*,*,#8132,.F.);
#11598=ORIENTED_EDGE('',*,*,#8271,.T.);
#11599=ORIENTED_EDGE('',*,*,#8272,.F.);
#11600=ORIENTED_EDGE('',*,*,#8273,.F.);
#11601=ORIENTED_EDGE('',*,*,#8105,.F.);
#11602=ORIENTED_EDGE('',*,*,#8273,.T.);
#11603=ORIENTED_EDGE('',*,*,#8274,.T.);
#11604=ORIENTED_EDGE('',*,*,#8202,.F.);
#11605=ORIENTED_EDGE('',*,*,#8274,.F.);
#11606=ORIENTED_EDGE('',*,*,#8272,.T.);
#11607=ORIENTED_EDGE('',*,*,#8275,.T.);
#11608=ORIENTED_EDGE('',*,*,#8203,.F.);
#11609=ORIENTED_EDGE('',*,*,#8275,.F.);
#11610=ORIENTED_EDGE('',*,*,#8271,.F.);
#11611=ORIENTED_EDGE('',*,*,#8131,.F.);
#11612=ORIENTED_EDGE('',*,*,#8201,.F.);
#11613=ORIENTED_EDGE('',*,*,#8276,.T.);
#11614=ORIENTED_EDGE('',*,*,#8277,.F.);
#11615=ORIENTED_EDGE('',*,*,#8278,.F.);
#11616=ORIENTED_EDGE('',*,*,#8107,.F.);
#11617=ORIENTED_EDGE('',*,*,#8278,.T.);
#11618=ORIENTED_EDGE('',*,*,#8279,.T.);
#11619=ORIENTED_EDGE('',*,*,#8199,.F.);
#11620=ORIENTED_EDGE('',*,*,#8279,.F.);
#11621=ORIENTED_EDGE('',*,*,#8277,.T.);
#11622=ORIENTED_EDGE('',*,*,#8280,.T.);
#11623=ORIENTED_EDGE('',*,*,#8200,.F.);
#11624=ORIENTED_EDGE('',*,*,#8280,.F.);
#11625=ORIENTED_EDGE('',*,*,#8276,.F.);
#11626=ORIENTED_EDGE('',*,*,#8198,.F.);
#11627=ORIENTED_EDGE('',*,*,#8281,.T.);
#11628=ORIENTED_EDGE('',*,*,#8282,.F.);
#11629=ORIENTED_EDGE('',*,*,#8283,.F.);
#11630=ORIENTED_EDGE('',*,*,#8109,.F.);
#11631=ORIENTED_EDGE('',*,*,#8283,.T.);
#11632=ORIENTED_EDGE('',*,*,#8284,.T.);
#11633=ORIENTED_EDGE('',*,*,#8196,.F.);
#11634=ORIENTED_EDGE('',*,*,#8284,.F.);
#11635=ORIENTED_EDGE('',*,*,#8282,.T.);
#11636=ORIENTED_EDGE('',*,*,#8285,.T.);
#11637=ORIENTED_EDGE('',*,*,#8197,.F.);
#11638=ORIENTED_EDGE('',*,*,#8285,.F.);
#11639=ORIENTED_EDGE('',*,*,#8281,.F.);
#11640=ORIENTED_EDGE('',*,*,#8195,.F.);
#11641=ORIENTED_EDGE('',*,*,#8286,.T.);
#11642=ORIENTED_EDGE('',*,*,#8287,.F.);
#11643=ORIENTED_EDGE('',*,*,#8288,.F.);
#11644=ORIENTED_EDGE('',*,*,#8111,.F.);
#11645=ORIENTED_EDGE('',*,*,#8288,.T.);
#11646=ORIENTED_EDGE('',*,*,#8289,.T.);
#11647=ORIENTED_EDGE('',*,*,#8193,.F.);
#11648=ORIENTED_EDGE('',*,*,#8289,.F.);
#11649=ORIENTED_EDGE('',*,*,#8287,.T.);
#11650=ORIENTED_EDGE('',*,*,#8290,.T.);
#11651=ORIENTED_EDGE('',*,*,#8194,.F.);
#11652=ORIENTED_EDGE('',*,*,#8290,.F.);
#11653=ORIENTED_EDGE('',*,*,#8286,.F.);
#11654=ORIENTED_EDGE('',*,*,#8192,.F.);
#11655=ORIENTED_EDGE('',*,*,#8291,.T.);
#11656=ORIENTED_EDGE('',*,*,#8292,.F.);
#11657=ORIENTED_EDGE('',*,*,#8293,.F.);
#11658=ORIENTED_EDGE('',*,*,#8113,.F.);
#11659=ORIENTED_EDGE('',*,*,#8293,.T.);
#11660=ORIENTED_EDGE('',*,*,#8294,.T.);
#11661=ORIENTED_EDGE('',*,*,#8190,.F.);
#11662=ORIENTED_EDGE('',*,*,#8294,.F.);
#11663=ORIENTED_EDGE('',*,*,#8292,.T.);
#11664=ORIENTED_EDGE('',*,*,#8295,.T.);
#11665=ORIENTED_EDGE('',*,*,#8191,.F.);
#11666=ORIENTED_EDGE('',*,*,#8295,.F.);
#11667=ORIENTED_EDGE('',*,*,#8291,.F.);
#11668=ORIENTED_EDGE('',*,*,#8189,.F.);
#11669=ORIENTED_EDGE('',*,*,#8296,.T.);
#11670=ORIENTED_EDGE('',*,*,#8297,.F.);
#11671=ORIENTED_EDGE('',*,*,#8298,.F.);
#11672=ORIENTED_EDGE('',*,*,#8115,.F.);
#11673=ORIENTED_EDGE('',*,*,#8298,.T.);
#11674=ORIENTED_EDGE('',*,*,#8299,.T.);
#11675=ORIENTED_EDGE('',*,*,#8187,.F.);
#11676=ORIENTED_EDGE('',*,*,#8299,.F.);
#11677=ORIENTED_EDGE('',*,*,#8297,.T.);
#11678=ORIENTED_EDGE('',*,*,#8300,.T.);
#11679=ORIENTED_EDGE('',*,*,#8188,.F.);
#11680=ORIENTED_EDGE('',*,*,#8300,.F.);
#11681=ORIENTED_EDGE('',*,*,#8296,.F.);
#11682=ORIENTED_EDGE('',*,*,#8186,.F.);
#11683=ORIENTED_EDGE('',*,*,#8301,.T.);
#11684=ORIENTED_EDGE('',*,*,#8302,.F.);
#11685=ORIENTED_EDGE('',*,*,#8303,.F.);
#11686=ORIENTED_EDGE('',*,*,#8117,.F.);
#11687=ORIENTED_EDGE('',*,*,#8303,.T.);
#11688=ORIENTED_EDGE('',*,*,#8304,.T.);
#11689=ORIENTED_EDGE('',*,*,#8184,.F.);
#11690=ORIENTED_EDGE('',*,*,#8304,.F.);
#11691=ORIENTED_EDGE('',*,*,#8302,.T.);
#11692=ORIENTED_EDGE('',*,*,#8305,.T.);
#11693=ORIENTED_EDGE('',*,*,#8185,.F.);
#11694=ORIENTED_EDGE('',*,*,#8305,.F.);
#11695=ORIENTED_EDGE('',*,*,#8301,.F.);
#11696=ORIENTED_EDGE('',*,*,#8183,.F.);
#11697=ORIENTED_EDGE('',*,*,#8306,.T.);
#11698=ORIENTED_EDGE('',*,*,#8307,.F.);
#11699=ORIENTED_EDGE('',*,*,#8308,.F.);
#11700=ORIENTED_EDGE('',*,*,#8119,.F.);
#11701=ORIENTED_EDGE('',*,*,#8308,.T.);
#11702=ORIENTED_EDGE('',*,*,#8309,.T.);
#11703=ORIENTED_EDGE('',*,*,#8181,.F.);
#11704=ORIENTED_EDGE('',*,*,#8309,.F.);
#11705=ORIENTED_EDGE('',*,*,#8307,.T.);
#11706=ORIENTED_EDGE('',*,*,#8310,.T.);
#11707=ORIENTED_EDGE('',*,*,#8182,.F.);
#11708=ORIENTED_EDGE('',*,*,#8310,.F.);
#11709=ORIENTED_EDGE('',*,*,#8306,.F.);
#11710=ORIENTED_EDGE('',*,*,#8180,.F.);
#11711=ORIENTED_EDGE('',*,*,#8311,.T.);
#11712=ORIENTED_EDGE('',*,*,#8312,.F.);
#11713=ORIENTED_EDGE('',*,*,#8313,.F.);
#11714=ORIENTED_EDGE('',*,*,#8121,.F.);
#11715=ORIENTED_EDGE('',*,*,#8313,.T.);
#11716=ORIENTED_EDGE('',*,*,#8314,.T.);
#11717=ORIENTED_EDGE('',*,*,#8178,.F.);
#11718=ORIENTED_EDGE('',*,*,#8314,.F.);
#11719=ORIENTED_EDGE('',*,*,#8312,.T.);
#11720=ORIENTED_EDGE('',*,*,#8315,.T.);
#11721=ORIENTED_EDGE('',*,*,#8179,.F.);
#11722=ORIENTED_EDGE('',*,*,#8315,.F.);
#11723=ORIENTED_EDGE('',*,*,#8311,.F.);
#11724=ORIENTED_EDGE('',*,*,#8177,.F.);
#11725=ORIENTED_EDGE('',*,*,#8316,.T.);
#11726=ORIENTED_EDGE('',*,*,#8317,.F.);
#11727=ORIENTED_EDGE('',*,*,#8318,.F.);
#11728=ORIENTED_EDGE('',*,*,#8123,.F.);
#11729=ORIENTED_EDGE('',*,*,#8318,.T.);
#11730=ORIENTED_EDGE('',*,*,#8319,.T.);
#11731=ORIENTED_EDGE('',*,*,#8175,.F.);
#11732=ORIENTED_EDGE('',*,*,#8319,.F.);
#11733=ORIENTED_EDGE('',*,*,#8317,.T.);
#11734=ORIENTED_EDGE('',*,*,#8320,.T.);
#11735=ORIENTED_EDGE('',*,*,#8176,.F.);
#11736=ORIENTED_EDGE('',*,*,#8320,.F.);
#11737=ORIENTED_EDGE('',*,*,#8316,.F.);
#11738=ORIENTED_EDGE('',*,*,#8174,.F.);
#11739=ORIENTED_EDGE('',*,*,#8321,.T.);
#11740=ORIENTED_EDGE('',*,*,#8322,.F.);
#11741=ORIENTED_EDGE('',*,*,#8323,.F.);
#11742=ORIENTED_EDGE('',*,*,#8125,.F.);
#11743=ORIENTED_EDGE('',*,*,#8323,.T.);
#11744=ORIENTED_EDGE('',*,*,#8324,.T.);
#11745=ORIENTED_EDGE('',*,*,#8172,.F.);
#11746=ORIENTED_EDGE('',*,*,#8324,.F.);
#11747=ORIENTED_EDGE('',*,*,#8322,.T.);
#11748=ORIENTED_EDGE('',*,*,#8325,.T.);
#11749=ORIENTED_EDGE('',*,*,#8173,.F.);
#11750=ORIENTED_EDGE('',*,*,#8325,.F.);
#11751=ORIENTED_EDGE('',*,*,#8321,.F.);
#11752=ORIENTED_EDGE('',*,*,#8171,.F.);
#11753=ORIENTED_EDGE('',*,*,#8326,.T.);
#11754=ORIENTED_EDGE('',*,*,#8327,.F.);
#11755=ORIENTED_EDGE('',*,*,#8328,.F.);
#11756=ORIENTED_EDGE('',*,*,#8127,.F.);
#11757=ORIENTED_EDGE('',*,*,#8328,.T.);
#11758=ORIENTED_EDGE('',*,*,#8329,.T.);
#11759=ORIENTED_EDGE('',*,*,#8169,.F.);
#11760=ORIENTED_EDGE('',*,*,#8329,.F.);
#11761=ORIENTED_EDGE('',*,*,#8327,.T.);
#11762=ORIENTED_EDGE('',*,*,#8330,.T.);
#11763=ORIENTED_EDGE('',*,*,#8170,.F.);
#11764=ORIENTED_EDGE('',*,*,#8330,.F.);
#11765=ORIENTED_EDGE('',*,*,#8326,.F.);
#11766=ORIENTED_EDGE('',*,*,#8168,.F.);
#11767=ORIENTED_EDGE('',*,*,#8331,.T.);
#11768=ORIENTED_EDGE('',*,*,#8332,.F.);
#11769=ORIENTED_EDGE('',*,*,#8333,.F.);
#11770=ORIENTED_EDGE('',*,*,#8078,.F.);
#11771=ORIENTED_EDGE('',*,*,#8333,.T.);
#11772=ORIENTED_EDGE('',*,*,#8334,.T.);
#11773=ORIENTED_EDGE('',*,*,#8081,.F.);
#11774=ORIENTED_EDGE('',*,*,#8166,.F.);
#11775=ORIENTED_EDGE('',*,*,#8334,.F.);
#11776=ORIENTED_EDGE('',*,*,#8332,.T.);
#11777=ORIENTED_EDGE('',*,*,#8335,.T.);
#11778=ORIENTED_EDGE('',*,*,#8167,.F.);
#11779=ORIENTED_EDGE('',*,*,#8335,.F.);
#11780=ORIENTED_EDGE('',*,*,#8331,.F.);
#11781=ORIENTED_EDGE('',*,*,#8336,.F.);
#11782=ORIENTED_EDGE('',*,*,#8210,.F.);
#11783=ORIENTED_EDGE('',*,*,#7913,.F.);
#11784=ORIENTED_EDGE('',*,*,#8211,.F.);
#11785=ORIENTED_EDGE('',*,*,#8337,.T.);
#11786=ORIENTED_EDGE('',*,*,#8336,.T.);
#11787=ORIENTED_EDGE('',*,*,#8337,.F.);
#11788=ORIENTED_EDGE('',*,*,#7993,.T.);
#11789=ORIENTED_EDGE('',*,*,#8207,.T.);
#11790=ORIENTED_EDGE('',*,*,#8204,.F.);
#11791=ORIENTED_EDGE('',*,*,#8215,.T.);
#11792=ORIENTED_EDGE('',*,*,#8338,.F.);
#11793=ORIENTED_EDGE('',*,*,#8339,.T.);
#11794=ORIENTED_EDGE('',*,*,#8129,.T.);
#11795=ORIENTED_EDGE('',*,*,#8339,.F.);
#11796=ORIENTED_EDGE('',*,*,#8338,.T.);
#11797=ORIENTED_EDGE('',*,*,#8340,.F.);
#11798=ORIENTED_EDGE('',*,*,#8340,.T.);
#11799=ORIENTED_EDGE('',*,*,#8341,.T.);
#11800=ORIENTED_EDGE('',*,*,#8342,.F.);
#11801=ORIENTED_EDGE('',*,*,#8341,.F.);
#11802=ORIENTED_EDGE('',*,*,#8342,.T.);
#13726=PLANE('',#15591);
#13727=PLANE('',#15593);
#13728=PLANE('',#15598);
#13729=PLANE('',#15599);
#13730=PLANE('',#15600);
#13731=PLANE('',#15601);
#13732=PLANE('',#15602);
#13733=PLANE('',#15603);
#13734=PLANE('',#15604);
#13735=PLANE('',#15605);
#13736=PLANE('',#15606);
#13737=PLANE('',#15607);
#13738=PLANE('',#15608);
#13739=PLANE('',#15609);
#13740=PLANE('',#15610);
#13741=PLANE('',#15611);
#13742=PLANE('',#15612);
#13743=PLANE('',#15613);
#13744=PLANE('',#15614);
#13745=PLANE('',#15615);
#13746=PLANE('',#15616);
#13747=PLANE('',#15617);
#13748=PLANE('',#15618);
#13749=PLANE('',#15619);
#13750=PLANE('',#15620);
#13751=PLANE('',#15621);
#13752=PLANE('',#15622);
#13753=PLANE('',#15623);
#13754=PLANE('',#15624);
#13755=PLANE('',#15625);
#13756=PLANE('',#15626);
#13757=PLANE('',#15627);
#13758=PLANE('',#15628);
#13759=PLANE('',#15629);
#13760=PLANE('',#15630);
#13761=PLANE('',#15631);
#13762=PLANE('',#15632);
#13763=PLANE('',#15633);
#13764=PLANE('',#15634);
#13765=PLANE('',#15635);
#13766=PLANE('',#15636);
#13767=PLANE('',#15637);
#13768=PLANE('',#15638);
#13769=PLANE('',#15639);
#13770=PLANE('',#15640);
#13771=PLANE('',#15641);
#13772=PLANE('',#15642);
#13773=PLANE('',#15643);
#13774=PLANE('',#15644);
#13775=PLANE('',#15645);
#13776=PLANE('',#15646);
#13777=PLANE('',#15647);
#13778=PLANE('',#15648);
#13779=PLANE('',#15649);
#13780=PLANE('',#15650);
#13781=PLANE('',#15651);
#13782=PLANE('',#15652);
#13783=PLANE('',#15653);
#13784=PLANE('',#15654);
#13785=PLANE('',#15655);
#13786=PLANE('',#15656);
#13787=PLANE('',#15657);
#13788=PLANE('',#15658);
#13789=PLANE('',#15659);
#13790=PLANE('',#15660);
#13791=PLANE('',#15661);
#13792=PLANE('',#15662);
#13793=PLANE('',#15663);
#13794=PLANE('',#15664);
#13795=PLANE('',#15665);
#13796=PLANE('',#15666);
#13797=PLANE('',#15667);
#13798=PLANE('',#15668);
#13799=PLANE('',#15669);
#13800=PLANE('',#15670);
#13801=PLANE('',#15671);
#13802=PLANE('',#15672);
#13803=PLANE('',#15673);
#13804=PLANE('',#15674);
#13805=PLANE('',#15675);
#13806=PLANE('',#15676);
#13807=PLANE('',#15677);
#13808=PLANE('',#15678);
#13809=PLANE('',#15679);
#13810=PLANE('',#15680);
#13811=PLANE('',#15681);
#13812=PLANE('',#15682);
#13813=PLANE('',#15683);
#13814=PLANE('',#15684);
#13815=PLANE('',#15685);
#13816=PLANE('',#15686);
#13817=PLANE('',#15687);
#13818=PLANE('',#15688);
#13819=PLANE('',#15689);
#13820=PLANE('',#15690);
#13821=PLANE('',#15691);
#13822=PLANE('',#15692);
#13823=PLANE('',#15693);
#13824=PLANE('',#15694);
#13825=PLANE('',#15700);
#13826=PLANE('',#15704);
#14312=ADVANCED_FACE('',(#1744),#727,.T.);
#14313=ADVANCED_FACE('',(#1745),#728,.T.);
#14314=ADVANCED_FACE('',(#1746),#729,.T.);
#14315=ADVANCED_FACE('',(#1747),#730,.T.);
#14316=ADVANCED_FACE('',(#1748),#731,.T.);
#14317=ADVANCED_FACE('',(#1749),#732,.T.);
#14318=ADVANCED_FACE('',(#1750),#733,.T.);
#14319=ADVANCED_FACE('',(#1751),#734,.T.);
#14320=ADVANCED_FACE('',(#1752),#735,.T.);
#14321=ADVANCED_FACE('',(#1753),#736,.T.);
#14322=ADVANCED_FACE('',(#1754),#737,.T.);
#14323=ADVANCED_FACE('',(#1755),#738,.T.);
#14324=ADVANCED_FACE('',(#1756),#739,.T.);
#14325=ADVANCED_FACE('',(#1757),#740,.T.);
#14326=ADVANCED_FACE('',(#1758),#741,.T.);
#14327=ADVANCED_FACE('',(#1759),#742,.T.);
#14328=ADVANCED_FACE('',(#1760),#743,.T.);
#14329=ADVANCED_FACE('',(#1761),#744,.T.);
#14330=ADVANCED_FACE('',(#1762),#745,.T.);
#14331=ADVANCED_FACE('',(#1763),#746,.T.);
#14332=ADVANCED_FACE('',(#1764),#747,.T.);
#14333=ADVANCED_FACE('',(#1765),#748,.T.);
#14334=ADVANCED_FACE('',(#1766),#749,.T.);
#14335=ADVANCED_FACE('',(#1767),#750,.T.);
#14336=ADVANCED_FACE('',(#1768),#751,.T.);
#14337=ADVANCED_FACE('',(#1769),#752,.T.);
#14338=ADVANCED_FACE('',(#1770),#753,.T.);
#14339=ADVANCED_FACE('',(#1771),#754,.T.);
#14340=ADVANCED_FACE('',(#1772),#755,.T.);
#14341=ADVANCED_FACE('',(#1773),#756,.T.);
#14342=ADVANCED_FACE('',(#1774),#757,.T.);
#14343=ADVANCED_FACE('',(#1775),#758,.T.);
#14344=ADVANCED_FACE('',(#1776),#759,.T.);
#14345=ADVANCED_FACE('',(#1777),#760,.T.);
#14346=ADVANCED_FACE('',(#1778),#761,.T.);
#14347=ADVANCED_FACE('',(#1779),#762,.T.);
#14348=ADVANCED_FACE('',(#1780),#763,.T.);
#14349=ADVANCED_FACE('',(#1781),#764,.T.);
#14350=ADVANCED_FACE('',(#1782),#765,.T.);
#14351=ADVANCED_FACE('',(#1783),#766,.T.);
#14352=ADVANCED_FACE('',(#1784),#767,.T.);
#14353=ADVANCED_FACE('',(#1785),#768,.T.);
#14354=ADVANCED_FACE('',(#1786),#769,.T.);
#14355=ADVANCED_FACE('',(#1787),#770,.T.);
#14356=ADVANCED_FACE('',(#1788),#771,.T.);
#14357=ADVANCED_FACE('',(#1789),#772,.T.);
#14358=ADVANCED_FACE('',(#1790),#773,.T.);
#14359=ADVANCED_FACE('',(#1791),#774,.T.);
#14360=ADVANCED_FACE('',(#1792),#775,.T.);
#14361=ADVANCED_FACE('',(#1793),#776,.T.);
#14362=ADVANCED_FACE('',(#1794),#777,.T.);
#14363=ADVANCED_FACE('',(#1795),#778,.T.);
#14364=ADVANCED_FACE('',(#1796),#779,.T.);
#14365=ADVANCED_FACE('',(#1797),#780,.T.);
#14366=ADVANCED_FACE('',(#1798),#781,.T.);
#14367=ADVANCED_FACE('',(#1799),#1349,.T.);
#14368=ADVANCED_FACE('',(#1800),#782,.T.);
#14369=ADVANCED_FACE('',(#1801,#676),#13726,.T.);
#14370=ADVANCED_FACE('',(#1802),#111,.F.);
#14371=ADVANCED_FACE('',(#1803),#13727,.T.);
#14372=ADVANCED_FACE('',(#1804),#783,.T.);
#14373=ADVANCED_FACE('',(#1805),#112,.F.);
#14374=ADVANCED_FACE('',(#1806),#13728,.F.);
#14375=ADVANCED_FACE('',(#1807),#13729,.T.);
#14376=ADVANCED_FACE('',(#1808),#13730,.F.);
#14377=ADVANCED_FACE('',(#1809),#13731,.F.);
#14378=ADVANCED_FACE('',(#1810),#13732,.F.);
#14379=ADVANCED_FACE('',(#1811),#13733,.T.);
#14380=ADVANCED_FACE('',(#1812),#13734,.F.);
#14381=ADVANCED_FACE('',(#1813),#13735,.F.);
#14382=ADVANCED_FACE('',(#1814),#13736,.F.);
#14383=ADVANCED_FACE('',(#1815),#13737,.T.);
#14384=ADVANCED_FACE('',(#1816),#13738,.F.);
#14385=ADVANCED_FACE('',(#1817),#13739,.F.);
#14386=ADVANCED_FACE('',(#1818),#13740,.F.);
#14387=ADVANCED_FACE('',(#1819),#13741,.T.);
#14388=ADVANCED_FACE('',(#1820),#13742,.F.);
#14389=ADVANCED_FACE('',(#1821),#13743,.F.);
#14390=ADVANCED_FACE('',(#1822),#13744,.F.);
#14391=ADVANCED_FACE('',(#1823),#13745,.T.);
#14392=ADVANCED_FACE('',(#1824),#13746,.F.);
#14393=ADVANCED_FACE('',(#1825),#13747,.F.);
#14394=ADVANCED_FACE('',(#1826),#13748,.F.);
#14395=ADVANCED_FACE('',(#1827),#13749,.T.);
#14396=ADVANCED_FACE('',(#1828),#13750,.F.);
#14397=ADVANCED_FACE('',(#1829),#13751,.F.);
#14398=ADVANCED_FACE('',(#1830),#13752,.F.);
#14399=ADVANCED_FACE('',(#1831),#13753,.T.);
#14400=ADVANCED_FACE('',(#1832),#13754,.F.);
#14401=ADVANCED_FACE('',(#1833),#13755,.F.);
#14402=ADVANCED_FACE('',(#1834),#13756,.F.);
#14403=ADVANCED_FACE('',(#1835),#13757,.T.);
#14404=ADVANCED_FACE('',(#1836),#13758,.F.);
#14405=ADVANCED_FACE('',(#1837),#13759,.F.);
#14406=ADVANCED_FACE('',(#1838),#13760,.F.);
#14407=ADVANCED_FACE('',(#1839),#13761,.T.);
#14408=ADVANCED_FACE('',(#1840),#13762,.F.);
#14409=ADVANCED_FACE('',(#1841),#13763,.F.);
#14410=ADVANCED_FACE('',(#1842),#13764,.F.);
#14411=ADVANCED_FACE('',(#1843),#13765,.T.);
#14412=ADVANCED_FACE('',(#1844),#13766,.F.);
#14413=ADVANCED_FACE('',(#1845),#13767,.F.);
#14414=ADVANCED_FACE('',(#1846),#13768,.F.);
#14415=ADVANCED_FACE('',(#1847),#13769,.T.);
#14416=ADVANCED_FACE('',(#1848),#13770,.F.);
#14417=ADVANCED_FACE('',(#1849),#13771,.F.);
#14418=ADVANCED_FACE('',(#1850),#13772,.F.);
#14419=ADVANCED_FACE('',(#1851),#13773,.T.);
#14420=ADVANCED_FACE('',(#1852),#13774,.F.);
#14421=ADVANCED_FACE('',(#1853),#13775,.F.);
#14422=ADVANCED_FACE('',(#1854),#13776,.F.);
#14423=ADVANCED_FACE('',(#1855),#13777,.T.);
#14424=ADVANCED_FACE('',(#1856),#13778,.F.);
#14425=ADVANCED_FACE('',(#1857),#13779,.F.);
#14426=ADVANCED_FACE('',(#1858),#13780,.F.);
#14427=ADVANCED_FACE('',(#1859),#13781,.T.);
#14428=ADVANCED_FACE('',(#1860),#13782,.F.);
#14429=ADVANCED_FACE('',(#1861),#13783,.F.);
#14430=ADVANCED_FACE('',(#1862),#13784,.F.);
#14431=ADVANCED_FACE('',(#1863),#13785,.T.);
#14432=ADVANCED_FACE('',(#1864),#13786,.F.);
#14433=ADVANCED_FACE('',(#1865),#13787,.F.);
#14434=ADVANCED_FACE('',(#1866),#13788,.F.);
#14435=ADVANCED_FACE('',(#1867),#13789,.T.);
#14436=ADVANCED_FACE('',(#1868),#13790,.F.);
#14437=ADVANCED_FACE('',(#1869),#13791,.F.);
#14438=ADVANCED_FACE('',(#1870),#13792,.F.);
#14439=ADVANCED_FACE('',(#1871),#13793,.T.);
#14440=ADVANCED_FACE('',(#1872),#13794,.F.);
#14441=ADVANCED_FACE('',(#1873),#13795,.F.);
#14442=ADVANCED_FACE('',(#1874),#13796,.F.);
#14443=ADVANCED_FACE('',(#1875),#13797,.T.);
#14444=ADVANCED_FACE('',(#1876),#13798,.F.);
#14445=ADVANCED_FACE('',(#1877),#13799,.F.);
#14446=ADVANCED_FACE('',(#1878),#13800,.F.);
#14447=ADVANCED_FACE('',(#1879),#13801,.T.);
#14448=ADVANCED_FACE('',(#1880),#13802,.F.);
#14449=ADVANCED_FACE('',(#1881),#13803,.F.);
#14450=ADVANCED_FACE('',(#1882),#13804,.F.);
#14451=ADVANCED_FACE('',(#1883),#13805,.T.);
#14452=ADVANCED_FACE('',(#1884),#13806,.F.);
#14453=ADVANCED_FACE('',(#1885),#13807,.F.);
#14454=ADVANCED_FACE('',(#1886),#13808,.F.);
#14455=ADVANCED_FACE('',(#1887),#13809,.T.);
#14456=ADVANCED_FACE('',(#1888),#13810,.F.);
#14457=ADVANCED_FACE('',(#1889),#13811,.F.);
#14458=ADVANCED_FACE('',(#1890),#13812,.F.);
#14459=ADVANCED_FACE('',(#1891),#13813,.T.);
#14460=ADVANCED_FACE('',(#1892),#13814,.F.);
#14461=ADVANCED_FACE('',(#1893),#13815,.F.);
#14462=ADVANCED_FACE('',(#1894),#13816,.F.);
#14463=ADVANCED_FACE('',(#1895),#13817,.T.);
#14464=ADVANCED_FACE('',(#1896),#13818,.F.);
#14465=ADVANCED_FACE('',(#1897),#13819,.F.);
#14466=ADVANCED_FACE('',(#1898),#13820,.F.);
#14467=ADVANCED_FACE('',(#1899),#13821,.T.);
#14468=ADVANCED_FACE('',(#1900),#13822,.F.);
#14469=ADVANCED_FACE('',(#1901),#13823,.F.);
#14470=ADVANCED_FACE('',(#1902),#13824,.T.);
#14471=ADVANCED_FACE('',(#1903),#1350,.T.);
#14472=ADVANCED_FACE('',(#1904),#784,.T.);
#14473=ADVANCED_FACE('',(#1905),#1351,.T.);
#14474=ADVANCED_FACE('',(#1906,#677),#13825,.T.);
#14475=ADVANCED_FACE('',(#1907),#785,.F.);
#14476=ADVANCED_FACE('',(#1908),#13826,.T.);
#14782=CLOSED_SHELL('',(#14312,#14313,#14314,#14315,#14316,#14317,#14318,
#14319,#14320,#14321,#14322,#14323,#14324,#14325,#14326,#14327,#14328,#14329,
#14330,#14331,#14332,#14333,#14334,#14335,#14336,#14337,#14338,#14339,#14340,
#14341,#14342,#14343,#14344,#14345,#14346,#14347,#14348,#14349,#14350,#14351,
#14352,#14353,#14354,#14355,#14356,#14357,#14358,#14359,#14360,#14361,#14362,
#14363,#14364,#14365,#14366,#14367,#14368,#14369,#14370,#14371,#14372,#14373,
#14374,#14375,#14376,#14377,#14378,#14379,#14380,#14381,#14382,#14383,#14384,
#14385,#14386,#14387,#14388,#14389,#14390,#14391,#14392,#14393,#14394,#14395,
#14396,#14397,#14398,#14399,#14400,#14401,#14402,#14403,#14404,#14405,#14406,
#14407,#14408,#14409,#14410,#14411,#14412,#14413,#14414,#14415,#14416,#14417,
#14418,#14419,#14420,#14421,#14422,#14423,#14424,#14425,#14426,#14427,#14428,
#14429,#14430,#14431,#14432,#14433,#14434,#14435,#14436,#14437,#14438,#14439,
#14440,#14441,#14442,#14443,#14444,#14445,#14446,#14447,#14448,#14449,#14450,
#14451,#14452,#14453,#14454,#14455,#14456,#14457,#14458,#14459,#14460,#14461,
#14462,#14463,#14464,#14465,#14466,#14467,#14468,#14469,#14470,#14471,#14472,
#14473,#14474,#14475,#14476));
#15455=AXIS2_PLACEMENT_3D('',#21798,#17847,#17848);
#15456=AXIS2_PLACEMENT_3D('',#21799,#17849,#17850);
#15457=AXIS2_PLACEMENT_3D('',#21815,#17852,#17853);
#15458=AXIS2_PLACEMENT_3D('',#21823,#17854,#17855);
#15459=AXIS2_PLACEMENT_3D('',#21871,#17857,#17858);
#15460=AXIS2_PLACEMENT_3D('',#21919,#17860,#17861);
#15461=AXIS2_PLACEMENT_3D('',#21973,#17863,#17864);
#15462=AXIS2_PLACEMENT_3D('',#22021,#17866,#17867);
#15463=AXIS2_PLACEMENT_3D('',#22069,#17869,#17870);
#15464=AXIS2_PLACEMENT_3D('',#22123,#17872,#17873);
#15465=AXIS2_PLACEMENT_3D('',#22171,#17875,#17876);
#15466=AXIS2_PLACEMENT_3D('',#22219,#17878,#17879);
#15467=AXIS2_PLACEMENT_3D('',#22267,#17881,#17882);
#15468=AXIS2_PLACEMENT_3D('',#22321,#17884,#17885);
#15469=AXIS2_PLACEMENT_3D('',#22369,#17887,#17888);
#15470=AXIS2_PLACEMENT_3D('',#22417,#17890,#17891);
#15471=AXIS2_PLACEMENT_3D('',#22471,#17893,#17894);
#15472=AXIS2_PLACEMENT_3D('',#22519,#17896,#17897);
#15473=AXIS2_PLACEMENT_3D('',#22567,#17899,#17900);
#15474=AXIS2_PLACEMENT_3D('',#22621,#17902,#17903);
#15475=AXIS2_PLACEMENT_3D('',#22669,#17905,#17906);
#15476=AXIS2_PLACEMENT_3D('',#22717,#17908,#17909);
#15477=AXIS2_PLACEMENT_3D('',#22771,#17911,#17912);
#15478=AXIS2_PLACEMENT_3D('',#22819,#17914,#17915);
#15479=AXIS2_PLACEMENT_3D('',#22867,#17917,#17918);
#15480=AXIS2_PLACEMENT_3D('',#22921,#17920,#17921);
#15481=AXIS2_PLACEMENT_3D('',#22969,#17923,#17924);
#15482=AXIS2_PLACEMENT_3D('',#23017,#17926,#17927);
#15483=AXIS2_PLACEMENT_3D('',#23071,#17929,#17930);
#15484=AXIS2_PLACEMENT_3D('',#23119,#17932,#17933);
#15485=AXIS2_PLACEMENT_3D('',#23167,#17935,#17936);
#15486=AXIS2_PLACEMENT_3D('',#23182,#17938,#17939);
#15487=AXIS2_PLACEMENT_3D('',#23191,#17940,#17941);
#15488=AXIS2_PLACEMENT_3D('',#23215,#17943,#17944);
#15489=AXIS2_PLACEMENT_3D('',#23240,#17946,#17947);
#15490=AXIS2_PLACEMENT_3D('',#23265,#17949,#17950);
#15491=AXIS2_PLACEMENT_3D('',#23289,#17952,#17953);
#15492=AXIS2_PLACEMENT_3D('',#23314,#17955,#17956);
#15493=AXIS2_PLACEMENT_3D('',#23339,#17958,#17959);
#15494=AXIS2_PLACEMENT_3D('',#23363,#17961,#17962);
#15495=AXIS2_PLACEMENT_3D('',#23388,#17964,#17965);
#15496=AXIS2_PLACEMENT_3D('',#23413,#17967,#17968);
#15497=AXIS2_PLACEMENT_3D('',#23437,#17970,#17971);
#15498=AXIS2_PLACEMENT_3D('',#23462,#17973,#17974);
#15499=AXIS2_PLACEMENT_3D('',#23487,#17976,#17977);
#15500=AXIS2_PLACEMENT_3D('',#23511,#17979,#17980);
#15501=AXIS2_PLACEMENT_3D('',#23536,#17982,#17983);
#15502=AXIS2_PLACEMENT_3D('',#23561,#17985,#17986);
#15503=AXIS2_PLACEMENT_3D('',#23585,#17988,#17989);
#15504=AXIS2_PLACEMENT_3D('',#23610,#17991,#17992);
#15505=AXIS2_PLACEMENT_3D('',#23635,#17994,#17995);
#15506=AXIS2_PLACEMENT_3D('',#23659,#17997,#17998);
#15507=AXIS2_PLACEMENT_3D('',#23683,#18000,#18001);
#15508=AXIS2_PLACEMENT_3D('',#23708,#18003,#18004);
#15509=AXIS2_PLACEMENT_3D('',#23733,#18006,#18007);
#15510=AXIS2_PLACEMENT_3D('',#23757,#18009,#18010);
#15511=AXIS2_PLACEMENT_3D('',#23782,#18012,#18013);
#15512=AXIS2_PLACEMENT_3D('',#23807,#18015,#18016);
#15513=AXIS2_PLACEMENT_3D('',#23831,#18018,#18019);
#15514=AXIS2_PLACEMENT_3D('',#23834,#18020,#18021);
#15515=AXIS2_PLACEMENT_3D('',#23837,#18023,#18024);
#15516=AXIS2_PLACEMENT_3D('',#23839,#18025,#18026);
#15517=AXIS2_PLACEMENT_3D('',#23841,#18027,#18028);
#15518=AXIS2_PLACEMENT_3D('',#23843,#18029,#18030);
#15519=AXIS2_PLACEMENT_3D('',#23845,#18031,#18032);
#15520=AXIS2_PLACEMENT_3D('',#23847,#18033,#18034);
#15521=AXIS2_PLACEMENT_3D('',#23849,#18035,#18036);
#15522=AXIS2_PLACEMENT_3D('',#23851,#18037,#18038);
#15523=AXIS2_PLACEMENT_3D('',#23853,#18039,#18040);
#15524=AXIS2_PLACEMENT_3D('',#23855,#18041,#18042);
#15525=AXIS2_PLACEMENT_3D('',#23857,#18043,#18044);
#15526=AXIS2_PLACEMENT_3D('',#23859,#18045,#18046);
#15527=AXIS2_PLACEMENT_3D('',#23861,#18047,#18048);
#15528=AXIS2_PLACEMENT_3D('',#23863,#18049,#18050);
#15529=AXIS2_PLACEMENT_3D('',#23865,#18051,#18052);
#15530=AXIS2_PLACEMENT_3D('',#23867,#18053,#18054);
#15531=AXIS2_PLACEMENT_3D('',#23869,#18055,#18056);
#15532=AXIS2_PLACEMENT_3D('',#23871,#18057,#18058);
#15533=AXIS2_PLACEMENT_3D('',#23873,#18059,#18060);
#15534=AXIS2_PLACEMENT_3D('',#23875,#18061,#18062);
#15535=AXIS2_PLACEMENT_3D('',#23877,#18063,#18064);
#15536=AXIS2_PLACEMENT_3D('',#23879,#18065,#18066);
#15537=AXIS2_PLACEMENT_3D('',#23881,#18067,#18068);
#15538=AXIS2_PLACEMENT_3D('',#23883,#18069,#18070);
#15539=AXIS2_PLACEMENT_3D('',#23885,#18071,#18072);
#15540=AXIS2_PLACEMENT_3D('',#23887,#18073,#18074);
#15541=AXIS2_PLACEMENT_3D('',#23889,#18075,#18076);
#15542=AXIS2_PLACEMENT_3D('',#23891,#18077,#18078);
#15543=AXIS2_PLACEMENT_3D('',#23893,#18079,#18080);
#15544=AXIS2_PLACEMENT_3D('',#23895,#18081,#18082);
#15545=AXIS2_PLACEMENT_3D('',#23897,#18083,#18084);
#15546=AXIS2_PLACEMENT_3D('',#23899,#18085,#18086);
#15547=AXIS2_PLACEMENT_3D('',#23901,#18087,#18088);
#15548=AXIS2_PLACEMENT_3D('',#23903,#18089,#18090);
#15549=AXIS2_PLACEMENT_3D('',#23905,#18091,#18092);
#15550=AXIS2_PLACEMENT_3D('',#23907,#18093,#18094);
#15551=AXIS2_PLACEMENT_3D('',#23909,#18095,#18096);
#15552=AXIS2_PLACEMENT_3D('',#23911,#18097,#18098);
#15553=AXIS2_PLACEMENT_3D('',#23913,#18099,#18100);
#15554=AXIS2_PLACEMENT_3D('',#23915,#18101,#18102);
#15555=AXIS2_PLACEMENT_3D('',#23917,#18103,#18104);
#15556=AXIS2_PLACEMENT_3D('',#23919,#18105,#18106);
#15557=AXIS2_PLACEMENT_3D('',#23921,#18107,#18108);
#15558=AXIS2_PLACEMENT_3D('',#23923,#18109,#18110);
#15559=AXIS2_PLACEMENT_3D('',#23925,#18111,#18112);
#15560=AXIS2_PLACEMENT_3D('',#23927,#18113,#18114);
#15561=AXIS2_PLACEMENT_3D('',#23929,#18115,#18116);
#15562=AXIS2_PLACEMENT_3D('',#23931,#18117,#18118);
#15563=AXIS2_PLACEMENT_3D('',#23932,#18119,#18120);
#15564=AXIS2_PLACEMENT_3D('',#23933,#18121,#18122);
#15565=AXIS2_PLACEMENT_3D('',#23935,#18123,#18124);
#15566=AXIS2_PLACEMENT_3D('',#23939,#18126,#18127);
#15567=AXIS2_PLACEMENT_3D('',#23944,#18130,#18131);
#15568=AXIS2_PLACEMENT_3D('',#23949,#18134,#18135);
#15569=AXIS2_PLACEMENT_3D('',#23954,#18138,#18139);
#15570=AXIS2_PLACEMENT_3D('',#23959,#18142,#18143);
#15571=AXIS2_PLACEMENT_3D('',#23964,#18146,#18147);
#15572=AXIS2_PLACEMENT_3D('',#23969,#18150,#18151);
#15573=AXIS2_PLACEMENT_3D('',#23974,#18154,#18155);
#15574=AXIS2_PLACEMENT_3D('',#23979,#18158,#18159);
#15575=AXIS2_PLACEMENT_3D('',#23984,#18162,#18163);
#15576=AXIS2_PLACEMENT_3D('',#23989,#18166,#18167);
#15577=AXIS2_PLACEMENT_3D('',#23994,#18170,#18171);
#15578=AXIS2_PLACEMENT_3D('',#23999,#18174,#18175);
#15579=AXIS2_PLACEMENT_3D('',#24004,#18178,#18179);
#15580=AXIS2_PLACEMENT_3D('',#24009,#18182,#18183);
#15581=AXIS2_PLACEMENT_3D('',#24014,#18186,#18187);
#15582=AXIS2_PLACEMENT_3D('',#24019,#18190,#18191);
#15583=AXIS2_PLACEMENT_3D('',#24024,#18194,#18195);
#15584=AXIS2_PLACEMENT_3D('',#24029,#18198,#18199);
#15585=AXIS2_PLACEMENT_3D('',#24034,#18202,#18203);
#15586=AXIS2_PLACEMENT_3D('',#24039,#18206,#18207);
#15587=AXIS2_PLACEMENT_3D('',#24044,#18210,#18211);
#15588=AXIS2_PLACEMENT_3D('',#24049,#18214,#18215);
#15589=AXIS2_PLACEMENT_3D('',#24054,#18218,#18219);
#15590=AXIS2_PLACEMENT_3D('',#24058,#18222,#18223);
#15591=AXIS2_PLACEMENT_3D('',#24059,#18224,#18225);
#15592=AXIS2_PLACEMENT_3D('',#24062,#18226,#18227);
#15593=AXIS2_PLACEMENT_3D('',#25090,#18228,#18229);
#15594=AXIS2_PLACEMENT_3D('',#25092,#18230,#18231);
#15595=AXIS2_PLACEMENT_3D('',#25093,#18232,#18233);
#15596=AXIS2_PLACEMENT_3D('',#25192,#18234,#18235);
#15597=AXIS2_PLACEMENT_3D('',#25193,#18236,#18237);
#15598=AXIS2_PLACEMENT_3D('',#25925,#18238,#18239);
#15599=AXIS2_PLACEMENT_3D('',#25931,#18243,#18244);
#15600=AXIS2_PLACEMENT_3D('',#25933,#18246,#18247);
#15601=AXIS2_PLACEMENT_3D('',#25935,#18249,#18250);
#15602=AXIS2_PLACEMENT_3D('',#25936,#18251,#18252);
#15603=AXIS2_PLACEMENT_3D('',#25942,#18256,#18257);
#15604=AXIS2_PLACEMENT_3D('',#25944,#18259,#18260);
#15605=AXIS2_PLACEMENT_3D('',#25946,#18262,#18263);
#15606=AXIS2_PLACEMENT_3D('',#25947,#18264,#18265);
#15607=AXIS2_PLACEMENT_3D('',#25953,#18269,#18270);
#15608=AXIS2_PLACEMENT_3D('',#25955,#18272,#18273);
#15609=AXIS2_PLACEMENT_3D('',#25957,#18275,#18276);
#15610=AXIS2_PLACEMENT_3D('',#25958,#18277,#18278);
#15611=AXIS2_PLACEMENT_3D('',#25964,#18282,#18283);
#15612=AXIS2_PLACEMENT_3D('',#25966,#18285,#18286);
#15613=AXIS2_PLACEMENT_3D('',#25968,#18288,#18289);
#15614=AXIS2_PLACEMENT_3D('',#25969,#18290,#18291);
#15615=AXIS2_PLACEMENT_3D('',#25975,#18295,#18296);
#15616=AXIS2_PLACEMENT_3D('',#25977,#18298,#18299);
#15617=AXIS2_PLACEMENT_3D('',#25979,#18301,#18302);
#15618=AXIS2_PLACEMENT_3D('',#25980,#18303,#18304);
#15619=AXIS2_PLACEMENT_3D('',#25986,#18308,#18309);
#15620=AXIS2_PLACEMENT_3D('',#25988,#18311,#18312);
#15621=AXIS2_PLACEMENT_3D('',#25990,#18314,#18315);
#15622=AXIS2_PLACEMENT_3D('',#25991,#18316,#18317);
#15623=AXIS2_PLACEMENT_3D('',#25997,#18321,#18322);
#15624=AXIS2_PLACEMENT_3D('',#25999,#18324,#18325);
#15625=AXIS2_PLACEMENT_3D('',#26001,#18327,#18328);
#15626=AXIS2_PLACEMENT_3D('',#26002,#18329,#18330);
#15627=AXIS2_PLACEMENT_3D('',#26008,#18334,#18335);
#15628=AXIS2_PLACEMENT_3D('',#26010,#18337,#18338);
#15629=AXIS2_PLACEMENT_3D('',#26012,#18340,#18341);
#15630=AXIS2_PLACEMENT_3D('',#26013,#18342,#18343);
#15631=AXIS2_PLACEMENT_3D('',#26019,#18347,#18348);
#15632=AXIS2_PLACEMENT_3D('',#26021,#18350,#18351);
#15633=AXIS2_PLACEMENT_3D('',#26023,#18353,#18354);
#15634=AXIS2_PLACEMENT_3D('',#26024,#18355,#18356);
#15635=AXIS2_PLACEMENT_3D('',#26030,#18360,#18361);
#15636=AXIS2_PLACEMENT_3D('',#26032,#18363,#18364);
#15637=AXIS2_PLACEMENT_3D('',#26034,#18366,#18367);
#15638=AXIS2_PLACEMENT_3D('',#26035,#18368,#18369);
#15639=AXIS2_PLACEMENT_3D('',#26041,#18373,#18374);
#15640=AXIS2_PLACEMENT_3D('',#26043,#18376,#18377);
#15641=AXIS2_PLACEMENT_3D('',#26045,#18379,#18380);
#15642=AXIS2_PLACEMENT_3D('',#26046,#18381,#18382);
#15643=AXIS2_PLACEMENT_3D('',#26052,#18386,#18387);
#15644=AXIS2_PLACEMENT_3D('',#26054,#18389,#18390);
#15645=AXIS2_PLACEMENT_3D('',#26056,#18392,#18393);
#15646=AXIS2_PLACEMENT_3D('',#26057,#18394,#18395);
#15647=AXIS2_PLACEMENT_3D('',#26063,#18399,#18400);
#15648=AXIS2_PLACEMENT_3D('',#26065,#18402,#18403);
#15649=AXIS2_PLACEMENT_3D('',#26067,#18405,#18406);
#15650=AXIS2_PLACEMENT_3D('',#26068,#18407,#18408);
#15651=AXIS2_PLACEMENT_3D('',#26074,#18412,#18413);
#15652=AXIS2_PLACEMENT_3D('',#26076,#18415,#18416);
#15653=AXIS2_PLACEMENT_3D('',#26078,#18418,#18419);
#15654=AXIS2_PLACEMENT_3D('',#26079,#18420,#18421);
#15655=AXIS2_PLACEMENT_3D('',#26085,#18425,#18426);
#15656=AXIS2_PLACEMENT_3D('',#26087,#18428,#18429);
#15657=AXIS2_PLACEMENT_3D('',#26089,#18431,#18432);
#15658=AXIS2_PLACEMENT_3D('',#26090,#18433,#18434);
#15659=AXIS2_PLACEMENT_3D('',#26096,#18438,#18439);
#15660=AXIS2_PLACEMENT_3D('',#26098,#18441,#18442);
#15661=AXIS2_PLACEMENT_3D('',#26100,#18444,#18445);
#15662=AXIS2_PLACEMENT_3D('',#26101,#18446,#18447);
#15663=AXIS2_PLACEMENT_3D('',#26107,#18451,#18452);
#15664=AXIS2_PLACEMENT_3D('',#26109,#18454,#18455);
#15665=AXIS2_PLACEMENT_3D('',#26111,#18457,#18458);
#15666=AXIS2_PLACEMENT_3D('',#26112,#18459,#18460);
#15667=AXIS2_PLACEMENT_3D('',#26118,#18464,#18465);
#15668=AXIS2_PLACEMENT_3D('',#26120,#18467,#18468);
#15669=AXIS2_PLACEMENT_3D('',#26122,#18470,#18471);
#15670=AXIS2_PLACEMENT_3D('',#26123,#18472,#18473);
#15671=AXIS2_PLACEMENT_3D('',#26129,#18477,#18478);
#15672=AXIS2_PLACEMENT_3D('',#26131,#18480,#18481);
#15673=AXIS2_PLACEMENT_3D('',#26133,#18483,#18484);
#15674=AXIS2_PLACEMENT_3D('',#26134,#18485,#18486);
#15675=AXIS2_PLACEMENT_3D('',#26140,#18490,#18491);
#15676=AXIS2_PLACEMENT_3D('',#26142,#18493,#18494);
#15677=AXIS2_PLACEMENT_3D('',#26144,#18496,#18497);
#15678=AXIS2_PLACEMENT_3D('',#26145,#18498,#18499);
#15679=AXIS2_PLACEMENT_3D('',#26151,#18503,#18504);
#15680=AXIS2_PLACEMENT_3D('',#26153,#18506,#18507);
#15681=AXIS2_PLACEMENT_3D('',#26155,#18509,#18510);
#15682=AXIS2_PLACEMENT_3D('',#26156,#18511,#18512);
#15683=AXIS2_PLACEMENT_3D('',#26162,#18516,#18517);
#15684=AXIS2_PLACEMENT_3D('',#26164,#18519,#18520);
#15685=AXIS2_PLACEMENT_3D('',#26166,#18522,#18523);
#15686=AXIS2_PLACEMENT_3D('',#26167,#18524,#18525);
#15687=AXIS2_PLACEMENT_3D('',#26173,#18529,#18530);
#15688=AXIS2_PLACEMENT_3D('',#26175,#18532,#18533);
#15689=AXIS2_PLACEMENT_3D('',#26177,#18535,#18536);
#15690=AXIS2_PLACEMENT_3D('',#26178,#18537,#18538);
#15691=AXIS2_PLACEMENT_3D('',#26184,#18542,#18543);
#15692=AXIS2_PLACEMENT_3D('',#26186,#18545,#18546);
#15693=AXIS2_PLACEMENT_3D('',#26188,#18548,#18549);
#15694=AXIS2_PLACEMENT_3D('',#26189,#18550,#18551);
#15695=AXIS2_PLACEMENT_3D('',#26191,#18552,#18553);
#15696=AXIS2_PLACEMENT_3D('',#26192,#18554,#18555);
#15697=AXIS2_PLACEMENT_3D('',#26194,#18557,#18558);
#15698=AXIS2_PLACEMENT_3D('',#26195,#18559,#18560);
#15699=AXIS2_PLACEMENT_3D('',#26197,#18561,#18562);
#15700=AXIS2_PLACEMENT_3D('',#26199,#18564,#18565);
#15701=AXIS2_PLACEMENT_3D('',#26201,#18566,#18567);
#15702=AXIS2_PLACEMENT_3D('',#26202,#18568,#18569);
#15703=AXIS2_PLACEMENT_3D('',#26205,#18571,#18572);
#15704=AXIS2_PLACEMENT_3D('',#26206,#18573,#18574);
#17847=DIRECTION('axis',(0.,0.,1.));
#17848=DIRECTION('refdir',(1.,0.,0.));
#17849=DIRECTION('center_axis',(1.,0.,0.));
#17850=DIRECTION('ref_axis',(0.,1.,0.));
#17851=DIRECTION('',(-1.,0.,0.));
#17852=DIRECTION('center_axis',(1.,0.,0.));
#17853=DIRECTION('ref_axis',(0.,1.,0.));
#17854=DIRECTION('center_axis',(1.,0.,0.));
#17855=DIRECTION('ref_axis',(0.,1.,0.));
#17856=DIRECTION('',(-1.,0.,0.));
#17857=DIRECTION('center_axis',(1.,0.,0.));
#17858=DIRECTION('ref_axis',(0.,1.,0.));
#17859=DIRECTION('',(-1.,0.,0.));
#17860=DIRECTION('center_axis',(1.,0.,0.));
#17861=DIRECTION('ref_axis',(0.,1.,0.));
#17862=DIRECTION('',(-1.,0.,0.));
#17863=DIRECTION('center_axis',(1.,0.,0.));
#17864=DIRECTION('ref_axis',(0.,1.,0.));
#17865=DIRECTION('',(-1.,0.,0.));
#17866=DIRECTION('center_axis',(1.,0.,0.));
#17867=DIRECTION('ref_axis',(0.,1.,0.));
#17868=DIRECTION('',(-1.,0.,0.));
#17869=DIRECTION('center_axis',(1.,0.,0.));
#17870=DIRECTION('ref_axis',(0.,1.,0.));
#17871=DIRECTION('',(-1.,0.,0.));
#17872=DIRECTION('center_axis',(1.,0.,0.));
#17873=DIRECTION('ref_axis',(0.,1.,0.));
#17874=DIRECTION('',(-1.,0.,0.));
#17875=DIRECTION('center_axis',(1.,0.,0.));
#17876=DIRECTION('ref_axis',(0.,1.,0.));
#17877=DIRECTION('',(-1.,0.,0.));
#17878=DIRECTION('center_axis',(1.,0.,0.));
#17879=DIRECTION('ref_axis',(0.,1.,0.));
#17880=DIRECTION('',(-1.,0.,0.));
#17881=DIRECTION('center_axis',(1.,0.,0.));
#17882=DIRECTION('ref_axis',(0.,1.,0.));
#17883=DIRECTION('',(-1.,0.,0.));
#17884=DIRECTION('center_axis',(1.,0.,0.));
#17885=DIRECTION('ref_axis',(0.,1.,0.));
#17886=DIRECTION('',(-1.,0.,0.));
#17887=DIRECTION('center_axis',(1.,0.,0.));
#17888=DIRECTION('ref_axis',(0.,1.,0.));
#17889=DIRECTION('',(-1.,0.,0.));
#17890=DIRECTION('center_axis',(1.,0.,0.));
#17891=DIRECTION('ref_axis',(0.,1.,0.));
#17892=DIRECTION('',(-1.,0.,0.));
#17893=DIRECTION('center_axis',(1.,0.,0.));
#17894=DIRECTION('ref_axis',(0.,1.,0.));
#17895=DIRECTION('',(-1.,0.,0.));
#17896=DIRECTION('center_axis',(1.,0.,0.));
#17897=DIRECTION('ref_axis',(0.,1.,0.));
#17898=DIRECTION('',(-1.,0.,0.));
#17899=DIRECTION('center_axis',(1.,0.,0.));
#17900=DIRECTION('ref_axis',(0.,1.,0.));
#17901=DIRECTION('',(-1.,0.,0.));
#17902=DIRECTION('center_axis',(1.,0.,0.));
#17903=DIRECTION('ref_axis',(0.,1.,0.));
#17904=DIRECTION('',(-1.,0.,0.));
#17905=DIRECTION('center_axis',(1.,0.,0.));
#17906=DIRECTION('ref_axis',(0.,1.,0.));
#17907=DIRECTION('',(-1.,0.,0.));
#17908=DIRECTION('center_axis',(1.,0.,0.));
#17909=DIRECTION('ref_axis',(0.,1.,0.));
#17910=DIRECTION('',(-1.,0.,0.));
#17911=DIRECTION('center_axis',(1.,0.,0.));
#17912=DIRECTION('ref_axis',(0.,1.,0.));
#17913=DIRECTION('',(-1.,0.,0.));
#17914=DIRECTION('center_axis',(1.,0.,0.));
#17915=DIRECTION('ref_axis',(0.,1.,0.));
#17916=DIRECTION('',(-1.,0.,0.));
#17917=DIRECTION('center_axis',(1.,0.,0.));
#17918=DIRECTION('ref_axis',(0.,1.,0.));
#17919=DIRECTION('',(-1.,0.,0.));
#17920=DIRECTION('center_axis',(1.,0.,0.));
#17921=DIRECTION('ref_axis',(0.,1.,0.));
#17922=DIRECTION('',(-1.,0.,0.));
#17923=DIRECTION('center_axis',(1.,0.,0.));
#17924=DIRECTION('ref_axis',(0.,1.,0.));
#17925=DIRECTION('',(-1.,0.,0.));
#17926=DIRECTION('center_axis',(1.,0.,0.));
#17927=DIRECTION('ref_axis',(0.,1.,0.));
#17928=DIRECTION('',(-1.,0.,0.));
#17929=DIRECTION('center_axis',(1.,0.,0.));
#17930=DIRECTION('ref_axis',(0.,1.,0.));
#17931=DIRECTION('',(-1.,0.,0.));
#17932=DIRECTION('center_axis',(1.,0.,0.));
#17933=DIRECTION('ref_axis',(0.,1.,0.));
#17934=DIRECTION('',(-1.,0.,0.));
#17935=DIRECTION('center_axis',(1.,0.,0.));
#17936=DIRECTION('ref_axis',(0.,0.925734886529886,-0.378173134769644));
#17937=DIRECTION('',(1.,0.,0.));
#17938=DIRECTION('center_axis',(1.,0.,0.));
#17939=DIRECTION('ref_axis',(0.,1.,-9.1414668091865E-14));
#17940=DIRECTION('center_axis',(1.,0.,0.));
#17941=DIRECTION('ref_axis',(0.,1.,-9.1414668091865E-14));
#17942=DIRECTION('',(1.,0.,0.));
#17943=DIRECTION('center_axis',(1.,0.,0.));
#17944=DIRECTION('ref_axis',(0.,1.,-9.1414668091865E-14));
#17945=DIRECTION('',(1.,0.,0.));
#17946=DIRECTION('center_axis',(1.,0.,0.));
#17947=DIRECTION('ref_axis',(0.,1.,-9.1414668091865E-14));
#17948=DIRECTION('',(1.,0.,0.));
#17949=DIRECTION('center_axis',(1.,0.,0.));
#17950=DIRECTION('ref_axis',(0.,1.,-9.1414668091865E-14));
#17951=DIRECTION('',(1.,0.,0.));
#17952=DIRECTION('center_axis',(1.,0.,0.));
#17953=DIRECTION('ref_axis',(0.,1.,-9.1414668091865E-14));
#17954=DIRECTION('',(1.,0.,0.));
#17955=DIRECTION('center_axis',(1.,0.,0.));
#17956=DIRECTION('ref_axis',(0.,1.,-9.1414668091865E-14));
#17957=DIRECTION('',(1.,0.,0.));
#17958=DIRECTION('center_axis',(1.,0.,0.));
#17959=DIRECTION('ref_axis',(0.,1.,-9.1414668091865E-14));
#17960=DIRECTION('',(1.,0.,0.));
#17961=DIRECTION('center_axis',(1.,0.,0.));
#17962=DIRECTION('ref_axis',(0.,1.,-9.1414668091865E-14));
#17963=DIRECTION('',(1.,0.,0.));
#17964=DIRECTION('center_axis',(1.,0.,0.));
#17965=DIRECTION('ref_axis',(0.,1.,-9.1414668091865E-14));
#17966=DIRECTION('',(1.,0.,0.));
#17967=DIRECTION('center_axis',(1.,0.,0.));
#17968=DIRECTION('ref_axis',(0.,1.,-9.1414668091865E-14));
#17969=DIRECTION('',(1.,0.,0.));
#17970=DIRECTION('center_axis',(1.,0.,0.));
#17971=DIRECTION('ref_axis',(0.,1.,-9.1414668091865E-14));
#17972=DIRECTION('',(1.,0.,0.));
#17973=DIRECTION('center_axis',(1.,0.,0.));
#17974=DIRECTION('ref_axis',(0.,1.,-9.1414668091865E-14));
#17975=DIRECTION('',(1.,0.,0.));
#17976=DIRECTION('center_axis',(1.,0.,0.));
#17977=DIRECTION('ref_axis',(0.,1.,-9.1414668091865E-14));
#17978=DIRECTION('',(1.,0.,0.));
#17979=DIRECTION('center_axis',(1.,0.,0.));
#17980=DIRECTION('ref_axis',(0.,1.,-9.1414668091865E-14));
#17981=DIRECTION('',(1.,0.,0.));
#17982=DIRECTION('center_axis',(1.,0.,0.));
#17983=DIRECTION('ref_axis',(0.,1.,-9.1414668091865E-14));
#17984=DIRECTION('',(1.,0.,0.));
#17985=DIRECTION('center_axis',(1.,0.,0.));
#17986=DIRECTION('ref_axis',(0.,1.,-9.1414668091865E-14));
#17987=DIRECTION('',(1.,0.,0.));
#17988=DIRECTION('center_axis',(1.,0.,0.));
#17989=DIRECTION('ref_axis',(0.,1.,-9.1414668091865E-14));
#17990=DIRECTION('',(1.,0.,0.));
#17991=DIRECTION('center_axis',(1.,0.,0.));
#17992=DIRECTION('ref_axis',(0.,1.,-9.1414668091865E-14));
#17993=DIRECTION('',(1.,0.,0.));
#17994=DIRECTION('center_axis',(1.,0.,0.));
#17995=DIRECTION('ref_axis',(0.,1.,-9.1414668091865E-14));
#17996=DIRECTION('',(1.,0.,0.));
#17997=DIRECTION('center_axis',(1.,0.,0.));
#17998=DIRECTION('ref_axis',(0.,1.,-9.1414668091865E-14));
#17999=DIRECTION('',(1.,0.,0.));
#18000=DIRECTION('center_axis',(1.,0.,0.));
#18001=DIRECTION('ref_axis',(0.,1.,-9.1414668091865E-14));
#18002=DIRECTION('',(1.,0.,0.));
#18003=DIRECTION('center_axis',(1.,0.,0.));
#18004=DIRECTION('ref_axis',(0.,1.,-9.1414668091865E-14));
#18005=DIRECTION('',(1.,0.,0.));
#18006=DIRECTION('center_axis',(1.,0.,0.));
#18007=DIRECTION('ref_axis',(0.,1.,-9.1414668091865E-14));
#18008=DIRECTION('',(1.,0.,0.));
#18009=DIRECTION('center_axis',(1.,0.,0.));
#18010=DIRECTION('ref_axis',(0.,1.,-9.1414668091865E-14));
#18011=DIRECTION('',(1.,0.,0.));
#18012=DIRECTION('center_axis',(1.,0.,0.));
#18013=DIRECTION('ref_axis',(0.,1.,-9.1414668091865E-14));
#18014=DIRECTION('',(1.,0.,0.));
#18015=DIRECTION('center_axis',(1.,0.,0.));
#18016=DIRECTION('ref_axis',(0.,1.,-9.1414668091865E-14));
#18017=DIRECTION('',(1.,0.,0.));
#18018=DIRECTION('center_axis',(1.,0.,0.));
#18019=DIRECTION('ref_axis',(0.,-1.,0.));
#18020=DIRECTION('center_axis',(-1.,0.,0.));
#18021=DIRECTION('ref_axis',(0.,1.,0.));
#18022=DIRECTION('',(-0.707106781186547,-0.707106781186547,-8.65956056235493E-17));
#18023=DIRECTION('center_axis',(1.,0.,0.));
#18024=DIRECTION('ref_axis',(0.,-1.,0.));
#18025=DIRECTION('center_axis',(-1.,0.,0.));
#18026=DIRECTION('ref_axis',(0.,1.,0.));
#18027=DIRECTION('center_axis',(-1.,0.,0.));
#18028=DIRECTION('ref_axis',(0.,-1.,0.));
#18029=DIRECTION('center_axis',(-1.,0.,0.));
#18030=DIRECTION('ref_axis',(0.,1.,0.));
#18031=DIRECTION('center_axis',(-1.,0.,0.));
#18032=DIRECTION('ref_axis',(0.,-1.,0.));
#18033=DIRECTION('center_axis',(-1.,0.,0.));
#18034=DIRECTION('ref_axis',(0.,1.,0.));
#18035=DIRECTION('center_axis',(-1.,0.,0.));
#18036=DIRECTION('ref_axis',(0.,-1.,0.));
#18037=DIRECTION('center_axis',(-1.,0.,0.));
#18038=DIRECTION('ref_axis',(0.,1.,0.));
#18039=DIRECTION('center_axis',(-1.,0.,0.));
#18040=DIRECTION('ref_axis',(0.,-1.,0.));
#18041=DIRECTION('center_axis',(-1.,0.,0.));
#18042=DIRECTION('ref_axis',(0.,1.,0.));
#18043=DIRECTION('center_axis',(-1.,0.,0.));
#18044=DIRECTION('ref_axis',(0.,-1.,0.));
#18045=DIRECTION('center_axis',(-1.,0.,0.));
#18046=DIRECTION('ref_axis',(0.,1.,0.));
#18047=DIRECTION('center_axis',(-1.,0.,0.));
#18048=DIRECTION('ref_axis',(0.,-1.,0.));
#18049=DIRECTION('center_axis',(-1.,0.,0.));
#18050=DIRECTION('ref_axis',(0.,1.,0.));
#18051=DIRECTION('center_axis',(-1.,0.,0.));
#18052=DIRECTION('ref_axis',(0.,-1.,0.));
#18053=DIRECTION('center_axis',(-1.,0.,0.));
#18054=DIRECTION('ref_axis',(0.,1.,0.));
#18055=DIRECTION('center_axis',(-1.,0.,0.));
#18056=DIRECTION('ref_axis',(0.,-1.,0.));
#18057=DIRECTION('center_axis',(-1.,0.,0.));
#18058=DIRECTION('ref_axis',(0.,1.,0.));
#18059=DIRECTION('center_axis',(-1.,0.,0.));
#18060=DIRECTION('ref_axis',(0.,-1.,0.));
#18061=DIRECTION('center_axis',(-1.,0.,0.));
#18062=DIRECTION('ref_axis',(0.,1.,0.));
#18063=DIRECTION('center_axis',(-1.,0.,0.));
#18064=DIRECTION('ref_axis',(0.,-1.,0.));
#18065=DIRECTION('center_axis',(-1.,0.,0.));
#18066=DIRECTION('ref_axis',(0.,1.,0.));
#18067=DIRECTION('center_axis',(-1.,0.,0.));
#18068=DIRECTION('ref_axis',(0.,-1.,0.));
#18069=DIRECTION('center_axis',(-1.,0.,0.));
#18070=DIRECTION('ref_axis',(0.,1.,0.));
#18071=DIRECTION('center_axis',(-1.,0.,0.));
#18072=DIRECTION('ref_axis',(0.,-1.,0.));
#18073=DIRECTION('center_axis',(-1.,0.,0.));
#18074=DIRECTION('ref_axis',(0.,1.,0.));
#18075=DIRECTION('center_axis',(-1.,0.,0.));
#18076=DIRECTION('ref_axis',(0.,-1.,0.));
#18077=DIRECTION('center_axis',(-1.,0.,0.));
#18078=DIRECTION('ref_axis',(0.,1.,0.));
#18079=DIRECTION('center_axis',(-1.,0.,0.));
#18080=DIRECTION('ref_axis',(0.,-1.,0.));
#18081=DIRECTION('center_axis',(-1.,0.,0.));
#18082=DIRECTION('ref_axis',(0.,1.,0.));
#18083=DIRECTION('center_axis',(-1.,0.,0.));
#18084=DIRECTION('ref_axis',(0.,-1.,0.));
#18085=DIRECTION('center_axis',(-1.,0.,0.));
#18086=DIRECTION('ref_axis',(0.,1.,0.));
#18087=DIRECTION('center_axis',(-1.,0.,0.));
#18088=DIRECTION('ref_axis',(0.,-1.,0.));
#18089=DIRECTION('center_axis',(-1.,0.,0.));
#18090=DIRECTION('ref_axis',(0.,1.,0.));
#18091=DIRECTION('center_axis',(-1.,0.,0.));
#18092=DIRECTION('ref_axis',(0.,-1.,0.));
#18093=DIRECTION('center_axis',(-1.,0.,0.));
#18094=DIRECTION('ref_axis',(0.,1.,0.));
#18095=DIRECTION('center_axis',(-1.,0.,0.));
#18096=DIRECTION('ref_axis',(0.,-1.,0.));
#18097=DIRECTION('center_axis',(-1.,0.,0.));
#18098=DIRECTION('ref_axis',(0.,1.,0.));
#18099=DIRECTION('center_axis',(-1.,0.,0.));
#18100=DIRECTION('ref_axis',(0.,-1.,0.));
#18101=DIRECTION('center_axis',(-1.,0.,0.));
#18102=DIRECTION('ref_axis',(0.,1.,0.));
#18103=DIRECTION('center_axis',(-1.,0.,0.));
#18104=DIRECTION('ref_axis',(0.,-1.,0.));
#18105=DIRECTION('center_axis',(-1.,0.,0.));
#18106=DIRECTION('ref_axis',(0.,1.,0.));
#18107=DIRECTION('center_axis',(-1.,0.,0.));
#18108=DIRECTION('ref_axis',(0.,-1.,0.));
#18109=DIRECTION('center_axis',(-1.,0.,0.));
#18110=DIRECTION('ref_axis',(0.,1.,0.));
#18111=DIRECTION('center_axis',(-1.,0.,0.));
#18112=DIRECTION('ref_axis',(0.,-1.,0.));
#18113=DIRECTION('center_axis',(-1.,0.,0.));
#18114=DIRECTION('ref_axis',(0.,1.,0.));
#18115=DIRECTION('center_axis',(-1.,0.,0.));
#18116=DIRECTION('ref_axis',(0.,-1.,0.));
#18117=DIRECTION('center_axis',(-1.,0.,0.));
#18118=DIRECTION('ref_axis',(0.,1.,0.));
#18119=DIRECTION('center_axis',(-1.,0.,0.));
#18120=DIRECTION('ref_axis',(0.,-1.,0.));
#18121=DIRECTION('center_axis',(1.,0.,0.));
#18122=DIRECTION('ref_axis',(0.,1.,0.));
#18123=DIRECTION('center_axis',(1.,0.,0.));
#18124=DIRECTION('ref_axis',(0.,0.,-1.));
#18125=DIRECTION('',(-1.,0.,0.));
#18126=DIRECTION('center_axis',(1.,0.,0.));
#18127=DIRECTION('ref_axis',(0.,1.,0.));
#18128=DIRECTION('',(-1.,0.,0.));
#18129=DIRECTION('',(1.,0.,0.));
#18130=DIRECTION('center_axis',(1.,0.,0.));
#18131=DIRECTION('ref_axis',(0.,1.,0.));
#18132=DIRECTION('',(-1.,0.,0.));
#18133=DIRECTION('',(1.,0.,0.));
#18134=DIRECTION('center_axis',(1.,0.,0.));
#18135=DIRECTION('ref_axis',(0.,1.,0.));
#18136=DIRECTION('',(-1.,0.,0.));
#18137=DIRECTION('',(1.,0.,0.));
#18138=DIRECTION('center_axis',(1.,0.,0.));
#18139=DIRECTION('ref_axis',(0.,1.,0.));
#18140=DIRECTION('',(-1.,0.,0.));
#18141=DIRECTION('',(1.,0.,0.));
#18142=DIRECTION('center_axis',(1.,0.,0.));
#18143=DIRECTION('ref_axis',(0.,1.,0.));
#18144=DIRECTION('',(-1.,0.,0.));
#18145=DIRECTION('',(1.,0.,0.));
#18146=DIRECTION('center_axis',(1.,0.,0.));
#18147=DIRECTION('ref_axis',(0.,1.,0.));
#18148=DIRECTION('',(-1.,0.,0.));
#18149=DIRECTION('',(1.,0.,0.));
#18150=DIRECTION('center_axis',(1.,0.,0.));
#18151=DIRECTION('ref_axis',(0.,1.,0.));
#18152=DIRECTION('',(-1.,0.,0.));
#18153=DIRECTION('',(1.,0.,0.));
#18154=DIRECTION('center_axis',(1.,0.,0.));
#18155=DIRECTION('ref_axis',(0.,1.,0.));
#18156=DIRECTION('',(-1.,0.,0.));
#18157=DIRECTION('',(1.,0.,0.));
#18158=DIRECTION('center_axis',(1.,0.,0.));
#18159=DIRECTION('ref_axis',(0.,1.,0.));
#18160=DIRECTION('',(-1.,0.,0.));
#18161=DIRECTION('',(1.,0.,0.));
#18162=DIRECTION('center_axis',(1.,0.,0.));
#18163=DIRECTION('ref_axis',(0.,1.,0.));
#18164=DIRECTION('',(-1.,0.,0.));
#18165=DIRECTION('',(1.,0.,0.));
#18166=DIRECTION('center_axis',(1.,0.,0.));
#18167=DIRECTION('ref_axis',(0.,1.,0.));
#18168=DIRECTION('',(-1.,0.,0.));
#18169=DIRECTION('',(1.,0.,0.));
#18170=DIRECTION('center_axis',(1.,0.,0.));
#18171=DIRECTION('ref_axis',(0.,1.,0.));
#18172=DIRECTION('',(-1.,0.,0.));
#18173=DIRECTION('',(1.,0.,0.));
#18174=DIRECTION('center_axis',(1.,0.,0.));
#18175=DIRECTION('ref_axis',(0.,1.,0.));
#18176=DIRECTION('',(-1.,0.,0.));
#18177=DIRECTION('',(1.,0.,0.));
#18178=DIRECTION('center_axis',(1.,0.,0.));
#18179=DIRECTION('ref_axis',(0.,1.,0.));
#18180=DIRECTION('',(-1.,0.,0.));
#18181=DIRECTION('',(1.,0.,0.));
#18182=DIRECTION('center_axis',(1.,0.,0.));
#18183=DIRECTION('ref_axis',(0.,1.,0.));
#18184=DIRECTION('',(-1.,0.,0.));
#18185=DIRECTION('',(1.,0.,0.));
#18186=DIRECTION('center_axis',(1.,0.,0.));
#18187=DIRECTION('ref_axis',(0.,1.,0.));
#18188=DIRECTION('',(-1.,0.,0.));
#18189=DIRECTION('',(1.,0.,0.));
#18190=DIRECTION('center_axis',(1.,0.,0.));
#18191=DIRECTION('ref_axis',(0.,1.,0.));
#18192=DIRECTION('',(-1.,0.,0.));
#18193=DIRECTION('',(1.,0.,0.));
#18194=DIRECTION('center_axis',(1.,0.,0.));
#18195=DIRECTION('ref_axis',(0.,1.,0.));
#18196=DIRECTION('',(-1.,0.,0.));
#18197=DIRECTION('',(1.,0.,0.));
#18198=DIRECTION('center_axis',(1.,0.,0.));
#18199=DIRECTION('ref_axis',(0.,1.,0.));
#18200=DIRECTION('',(-1.,0.,0.));
#18201=DIRECTION('',(1.,0.,0.));
#18202=DIRECTION('center_axis',(1.,0.,0.));
#18203=DIRECTION('ref_axis',(0.,1.,0.));
#18204=DIRECTION('',(-1.,0.,0.));
#18205=DIRECTION('',(1.,0.,0.));
#18206=DIRECTION('center_axis',(1.,0.,0.));
#18207=DIRECTION('ref_axis',(0.,1.,0.));
#18208=DIRECTION('',(-1.,0.,0.));
#18209=DIRECTION('',(1.,0.,0.));
#18210=DIRECTION('center_axis',(1.,0.,0.));
#18211=DIRECTION('ref_axis',(0.,1.,0.));
#18212=DIRECTION('',(-1.,0.,0.));
#18213=DIRECTION('',(1.,0.,0.));
#18214=DIRECTION('center_axis',(1.,0.,0.));
#18215=DIRECTION('ref_axis',(0.,1.,0.));
#18216=DIRECTION('',(-1.,0.,0.));
#18217=DIRECTION('',(1.,0.,0.));
#18218=DIRECTION('center_axis',(1.,0.,0.));
#18219=DIRECTION('ref_axis',(0.,1.,0.));
#18220=DIRECTION('',(-1.,0.,0.));
#18221=DIRECTION('',(1.,0.,0.));
#18222=DIRECTION('center_axis',(1.,0.,0.));
#18223=DIRECTION('ref_axis',(0.,1.,0.));
#18224=DIRECTION('center_axis',(-1.,0.,0.));
#18225=DIRECTION('ref_axis',(0.,0.,1.));
#18226=DIRECTION('center_axis',(1.,0.,0.));
#18227=DIRECTION('ref_axis',(0.,1.,0.));
#18228=DIRECTION('center_axis',(1.,0.,0.));
#18229=DIRECTION('ref_axis',(0.,0.,-1.));
#18230=DIRECTION('center_axis',(1.,0.,0.));
#18231=DIRECTION('ref_axis',(0.,1.,0.));
#18232=DIRECTION('center_axis',(1.,0.,0.));
#18233=DIRECTION('ref_axis',(0.,1.,0.));
#18234=DIRECTION('center_axis',(-1.,0.,0.));
#18235=DIRECTION('ref_axis',(0.,1.,-9.1414668091865E-14));
#18236=DIRECTION('center_axis',(1.,0.,0.));
#18237=DIRECTION('ref_axis',(0.,1.,-9.1414668091865E-14));
#18238=DIRECTION('center_axis',(0.,-0.372500259691423,0.928032088092768));
#18239=DIRECTION('ref_axis',(0.,-0.928032088092767,-0.372500259691423));
#18240=DIRECTION('',(0.,-0.928032088092767,-0.372500259691423));
#18241=DIRECTION('',(1.,0.,0.));
#18242=DIRECTION('',(0.,-0.928032088092767,-0.372500259691423));
#18243=DIRECTION('center_axis',(1.,0.,0.));
#18244=DIRECTION('ref_axis',(0.,-0.258819045102522,-0.965925826289068));
#18245=DIRECTION('',(0.,0.617449233969742,-0.786610731855458));
#18246=DIRECTION('center_axis',(0.,-0.786610731855458,-0.617449233969742));
#18247=DIRECTION('ref_axis',(0.,0.617449233969742,-0.786610731855458));
#18248=DIRECTION('',(0.,0.617449233969742,-0.786610731855458));
#18249=DIRECTION('center_axis',(1.,0.,0.));
#18250=DIRECTION('ref_axis',(0.,-0.258819045102522,-0.965925826289068));
#18251=DIRECTION('center_axis',(0.,-0.119615242270662,0.992820323027551));
#18252=DIRECTION('ref_axis',(0.,-0.992820323027551,-0.119615242270662));
#18253=DIRECTION('',(0.,-0.992820323027551,-0.119615242270662));
#18254=DIRECTION('',(1.,0.,0.));
#18255=DIRECTION('',(0.,-0.992820323027551,-0.119615242270662));
#18256=DIRECTION('center_axis',(1.,0.,0.));
#18257=DIRECTION('ref_axis',(0.,-0.5,-0.866025403784438));
#18258=DIRECTION('',(0.,0.392820323027551,-0.919615242270663));
#18259=DIRECTION('center_axis',(0.,-0.919615242270663,-0.392820323027551));
#18260=DIRECTION('ref_axis',(0.,0.392820323027551,-0.919615242270663));
#18261=DIRECTION('',(0.,0.392820323027551,-0.919615242270663));
#18262=DIRECTION('center_axis',(1.,0.,0.));
#18263=DIRECTION('ref_axis',(0.,-0.5,-0.866025403784438));
#18264=DIRECTION('center_axis',(0.,0.14142135623731,0.989949493661166));
#18265=DIRECTION('ref_axis',(0.,-0.989949493661166,0.14142135623731));
#18266=DIRECTION('',(0.,-0.989949493661166,0.14142135623731));
#18267=DIRECTION('',(1.,0.,0.));
#18268=DIRECTION('',(0.,-0.989949493661166,0.14142135623731));
#18269=DIRECTION('center_axis',(1.,0.,0.));
#18270=DIRECTION('ref_axis',(0.,-0.707106781186548,-0.707106781186547));
#18271=DIRECTION('',(0.,0.14142135623731,-0.989949493661167));
#18272=DIRECTION('center_axis',(0.,-0.989949493661167,-0.14142135623731));
#18273=DIRECTION('ref_axis',(0.,0.14142135623731,-0.989949493661167));
#18274=DIRECTION('',(0.,0.14142135623731,-0.989949493661167));
#18275=DIRECTION('center_axis',(1.,0.,0.));
#18276=DIRECTION('ref_axis',(0.,-0.707106781186548,-0.707106781186547));
#18277=DIRECTION('center_axis',(0.,0.392820323027552,0.919615242270663));
#18278=DIRECTION('ref_axis',(0.,-0.919615242270663,0.392820323027552));
#18279=DIRECTION('',(0.,-0.919615242270663,0.392820323027552));
#18280=DIRECTION('',(1.,0.,0.));
#18281=DIRECTION('',(0.,-0.919615242270663,0.392820323027552));
#18282=DIRECTION('center_axis',(1.,0.,0.));
#18283=DIRECTION('ref_axis',(0.,-0.866025403784439,-0.499999999999999));
#18284=DIRECTION('',(0.,-0.119615242270664,-0.992820323027551));
#18285=DIRECTION('center_axis',(0.,-0.992820323027551,0.119615242270664));
#18286=DIRECTION('ref_axis',(0.,-0.119615242270664,-0.992820323027551));
#18287=DIRECTION('',(0.,-0.119615242270664,-0.992820323027551));
#18288=DIRECTION('center_axis',(1.,0.,0.));
#18289=DIRECTION('ref_axis',(0.,-0.866025403784439,-0.499999999999999));
#18290=DIRECTION('center_axis',(0.,0.617449233969743,0.786610731855457));
#18291=DIRECTION('ref_axis',(0.,-0.786610731855457,0.617449233969743));
#18292=DIRECTION('',(0.,-0.786610731855457,0.617449233969743));
#18293=DIRECTION('',(1.,0.,0.));
#18294=DIRECTION('',(0.,-0.786610731855457,0.617449233969743));
#18295=DIRECTION('center_axis',(1.,0.,0.));
#18296=DIRECTION('ref_axis',(0.,-0.965925826289068,-0.25881904510252));
#18297=DIRECTION('',(0.,-0.372500259691424,-0.928032088092767));
#18298=DIRECTION('center_axis',(0.,-0.928032088092767,0.372500259691424));
#18299=DIRECTION('ref_axis',(0.,-0.372500259691424,-0.928032088092767));
#18300=DIRECTION('',(0.,-0.372500259691424,-0.928032088092767));
#18301=DIRECTION('center_axis',(1.,0.,0.));
#18302=DIRECTION('ref_axis',(0.,-0.965925826289068,-0.25881904510252));
#18303=DIRECTION('center_axis',(0.,0.8,0.6));
#18304=DIRECTION('ref_axis',(0.,-0.6,0.8));
#18305=DIRECTION('',(0.,-0.6,0.8));
#18306=DIRECTION('',(1.,0.,0.));
#18307=DIRECTION('',(0.,-0.6,0.8));
#18308=DIRECTION('center_axis',(1.,0.,0.));
#18309=DIRECTION('ref_axis',(0.,-1.,1.83697019872103E-16));
#18310=DIRECTION('',(0.,-0.6,-0.8));
#18311=DIRECTION('center_axis',(0.,-0.8,0.6));
#18312=DIRECTION('ref_axis',(0.,-0.6,-0.8));
#18313=DIRECTION('',(0.,-0.6,-0.8));
#18314=DIRECTION('center_axis',(1.,0.,0.));
#18315=DIRECTION('ref_axis',(0.,-1.,1.83697019872103E-16));
#18316=DIRECTION('center_axis',(0.,0.928032088092767,0.372500259691423));
#18317=DIRECTION('ref_axis',(0.,-0.372500259691423,0.928032088092767));
#18318=DIRECTION('',(0.,-0.372500259691423,0.928032088092767));
#18319=DIRECTION('',(1.,0.,0.));
#18320=DIRECTION('',(0.,-0.372500259691423,0.928032088092767));
#18321=DIRECTION('center_axis',(1.,0.,0.));
#18322=DIRECTION('ref_axis',(0.,-0.965925826289068,0.258819045102522));
#18323=DIRECTION('',(0.,-0.786610731855458,-0.617449233969742));
#18324=DIRECTION('center_axis',(0.,-0.617449233969742,0.786610731855458));
#18325=DIRECTION('ref_axis',(0.,-0.786610731855458,-0.617449233969742));
#18326=DIRECTION('',(0.,-0.786610731855458,-0.617449233969742));
#18327=DIRECTION('center_axis',(1.,0.,0.));
#18328=DIRECTION('ref_axis',(0.,-0.965925826289068,0.258819045102522));
#18329=DIRECTION('center_axis',(0.,0.992820323027551,0.119615242270662));
#18330=DIRECTION('ref_axis',(0.,-0.119615242270662,0.992820323027551));
#18331=DIRECTION('',(0.,-0.119615242270662,0.992820323027551));
#18332=DIRECTION('',(1.,0.,0.));
#18333=DIRECTION('',(0.,-0.119615242270662,0.992820323027551));
#18334=DIRECTION('center_axis',(1.,0.,0.));
#18335=DIRECTION('ref_axis',(0.,-0.866025403784438,0.5));
#18336=DIRECTION('',(0.,-0.919615242270663,-0.392820323027551));
#18337=DIRECTION('center_axis',(0.,-0.392820323027551,0.919615242270663));
#18338=DIRECTION('ref_axis',(0.,-0.919615242270663,-0.392820323027551));
#18339=DIRECTION('',(0.,-0.919615242270663,-0.392820323027551));
#18340=DIRECTION('center_axis',(1.,0.,0.));
#18341=DIRECTION('ref_axis',(0.,-0.866025403784438,0.5));
#18342=DIRECTION('center_axis',(0.,0.989949493661166,-0.14142135623731));
#18343=DIRECTION('ref_axis',(0.,0.14142135623731,0.989949493661166));
#18344=DIRECTION('',(0.,0.14142135623731,0.989949493661166));
#18345=DIRECTION('',(1.,0.,0.));
#18346=DIRECTION('',(0.,0.14142135623731,0.989949493661166));
#18347=DIRECTION('center_axis',(1.,0.,0.));
#18348=DIRECTION('ref_axis',(0.,-0.707106781186547,0.707106781186548));
#18349=DIRECTION('',(0.,-0.989949493661167,-0.141421356237309));
#18350=DIRECTION('center_axis',(0.,-0.141421356237309,0.989949493661167));
#18351=DIRECTION('ref_axis',(0.,-0.989949493661167,-0.141421356237309));
#18352=DIRECTION('',(0.,-0.989949493661167,-0.141421356237309));
#18353=DIRECTION('center_axis',(1.,0.,0.));
#18354=DIRECTION('ref_axis',(0.,-0.707106781186547,0.707106781186548));
#18355=DIRECTION('center_axis',(0.,0.919615242270663,-0.392820323027552));
#18356=DIRECTION('ref_axis',(0.,0.392820323027552,0.919615242270663));
#18357=DIRECTION('',(0.,0.392820323027552,0.919615242270663));
#18358=DIRECTION('',(1.,0.,0.));
#18359=DIRECTION('',(0.,0.392820323027552,0.919615242270663));
#18360=DIRECTION('center_axis',(1.,0.,0.));
#18361=DIRECTION('ref_axis',(0.,-0.5,0.866025403784439));
#18362=DIRECTION('',(0.,-0.992820323027551,0.119615242270663));
#18363=DIRECTION('center_axis',(0.,0.119615242270663,0.992820323027551));
#18364=DIRECTION('ref_axis',(0.,-0.992820323027551,0.119615242270663));
#18365=DIRECTION('',(0.,-0.992820323027551,0.119615242270663));
#18366=DIRECTION('center_axis',(1.,0.,0.));
#18367=DIRECTION('ref_axis',(0.,-0.5,0.866025403784439));
#18368=DIRECTION('center_axis',(0.,0.786610731855457,-0.617449233969743));
#18369=DIRECTION('ref_axis',(0.,0.617449233969743,0.786610731855457));
#18370=DIRECTION('',(0.,0.617449233969743,0.786610731855457));
#18371=DIRECTION('',(1.,0.,0.));
#18372=DIRECTION('',(0.,0.617449233969743,0.786610731855457));
#18373=DIRECTION('center_axis',(1.,0.,0.));
#18374=DIRECTION('ref_axis',(0.,-0.25881904510252,0.965925826289068));
#18375=DIRECTION('',(0.,-0.928032088092767,0.372500259691424));
#18376=DIRECTION('center_axis',(0.,0.372500259691424,0.928032088092767));
#18377=DIRECTION('ref_axis',(0.,-0.928032088092767,0.372500259691424));
#18378=DIRECTION('',(0.,-0.928032088092767,0.372500259691424));
#18379=DIRECTION('center_axis',(1.,0.,0.));
#18380=DIRECTION('ref_axis',(0.,-0.25881904510252,0.965925826289068));
#18381=DIRECTION('center_axis',(0.,0.6,-0.8));
#18382=DIRECTION('ref_axis',(0.,0.8,0.6));
#18383=DIRECTION('',(0.,0.8,0.6));
#18384=DIRECTION('',(1.,0.,0.));
#18385=DIRECTION('',(0.,0.8,0.6));
#18386=DIRECTION('center_axis',(1.,0.,0.));
#18387=DIRECTION('ref_axis',(0.,1.22464679914735E-16,1.));
#18388=DIRECTION('',(0.,-0.8,0.6));
#18389=DIRECTION('center_axis',(0.,0.6,0.8));
#18390=DIRECTION('ref_axis',(0.,-0.8,0.6));
#18391=DIRECTION('',(0.,-0.8,0.6));
#18392=DIRECTION('center_axis',(1.,0.,0.));
#18393=DIRECTION('ref_axis',(0.,1.22464679914735E-16,1.));
#18394=DIRECTION('center_axis',(0.,0.372500259691424,-0.928032088092767));
#18395=DIRECTION('ref_axis',(0.,0.928032088092767,0.372500259691424));
#18396=DIRECTION('',(0.,0.928032088092767,0.372500259691424));
#18397=DIRECTION('',(1.,0.,0.));
#18398=DIRECTION('',(0.,0.928032088092767,0.372500259691424));
#18399=DIRECTION('center_axis',(1.,0.,0.));
#18400=DIRECTION('ref_axis',(0.,0.258819045102521,0.965925826289068));
#18401=DIRECTION('',(0.,-0.617449233969742,0.786610731855457));
#18402=DIRECTION('center_axis',(0.,0.786610731855457,0.617449233969742));
#18403=DIRECTION('ref_axis',(0.,-0.617449233969742,0.786610731855457));
#18404=DIRECTION('',(0.,-0.617449233969742,0.786610731855457));
#18405=DIRECTION('center_axis',(1.,0.,0.));
#18406=DIRECTION('ref_axis',(0.,0.258819045102521,0.965925826289068));
#18407=DIRECTION('center_axis',(0.,0.119615242270662,-0.992820323027551));
#18408=DIRECTION('ref_axis',(0.,0.992820323027551,0.119615242270662));
#18409=DIRECTION('',(0.,0.992820323027551,0.119615242270662));
#18410=DIRECTION('',(1.,0.,0.));
#18411=DIRECTION('',(0.,0.992820323027551,0.119615242270662));
#18412=DIRECTION('center_axis',(1.,0.,0.));
#18413=DIRECTION('ref_axis',(0.,0.5,0.866025403784438));
#18414=DIRECTION('',(0.,-0.392820323027551,0.919615242270663));
#18415=DIRECTION('center_axis',(0.,0.919615242270663,0.392820323027551));
#18416=DIRECTION('ref_axis',(0.,-0.392820323027551,0.919615242270663));
#18417=DIRECTION('',(0.,-0.392820323027551,0.919615242270663));
#18418=DIRECTION('center_axis',(1.,0.,0.));
#18419=DIRECTION('ref_axis',(0.,0.5,0.866025403784438));
#18420=DIRECTION('center_axis',(0.,-0.14142135623731,-0.989949493661166));
#18421=DIRECTION('ref_axis',(0.,0.989949493661166,-0.14142135623731));
#18422=DIRECTION('',(0.,0.989949493661166,-0.14142135623731));
#18423=DIRECTION('',(1.,0.,0.));
#18424=DIRECTION('',(0.,0.989949493661166,-0.14142135623731));
#18425=DIRECTION('center_axis',(1.,0.,0.));
#18426=DIRECTION('ref_axis',(0.,0.707106781186548,0.707106781186547));
#18427=DIRECTION('',(0.,-0.14142135623731,0.989949493661167));
#18428=DIRECTION('center_axis',(0.,0.989949493661166,0.14142135623731));
#18429=DIRECTION('ref_axis',(0.,-0.14142135623731,0.989949493661167));
#18430=DIRECTION('',(0.,-0.14142135623731,0.989949493661167));
#18431=DIRECTION('center_axis',(1.,0.,0.));
#18432=DIRECTION('ref_axis',(0.,0.707106781186548,0.707106781186547));
#18433=DIRECTION('center_axis',(0.,-0.392820323027552,-0.919615242270663));
#18434=DIRECTION('ref_axis',(0.,0.919615242270663,-0.392820323027551));
#18435=DIRECTION('',(0.,0.919615242270663,-0.392820323027551));
#18436=DIRECTION('',(1.,0.,0.));
#18437=DIRECTION('',(0.,0.919615242270663,-0.392820323027551));
#18438=DIRECTION('center_axis',(1.,0.,0.));
#18439=DIRECTION('ref_axis',(0.,0.866025403784439,0.5));
#18440=DIRECTION('',(0.,0.119615242270663,0.992820323027551));
#18441=DIRECTION('center_axis',(0.,0.992820323027551,-0.119615242270663));
#18442=DIRECTION('ref_axis',(0.,0.119615242270663,0.992820323027551));
#18443=DIRECTION('',(0.,0.119615242270663,0.992820323027551));
#18444=DIRECTION('center_axis',(1.,0.,0.));
#18445=DIRECTION('ref_axis',(0.,0.866025403784439,0.5));
#18446=DIRECTION('center_axis',(0.,-0.617449233969743,-0.786610731855457));
#18447=DIRECTION('ref_axis',(0.,0.786610731855457,-0.617449233969743));
#18448=DIRECTION('',(0.,0.786610731855457,-0.617449233969743));
#18449=DIRECTION('',(1.,0.,0.));
#18450=DIRECTION('',(0.,0.786610731855457,-0.617449233969743));
#18451=DIRECTION('center_axis',(1.,0.,0.));
#18452=DIRECTION('ref_axis',(0.,0.965925826289068,0.258819045102521));
#18453=DIRECTION('',(0.,0.372500259691424,0.928032088092767));
#18454=DIRECTION('center_axis',(0.,0.928032088092767,-0.372500259691424));
#18455=DIRECTION('ref_axis',(0.,0.372500259691424,0.928032088092767));
#18456=DIRECTION('',(0.,0.372500259691424,0.928032088092767));
#18457=DIRECTION('center_axis',(1.,0.,0.));
#18458=DIRECTION('ref_axis',(0.,0.965925826289068,0.258819045102521));
#18459=DIRECTION('center_axis',(0.,-0.8,-0.6));
#18460=DIRECTION('ref_axis',(0.,0.6,-0.8));
#18461=DIRECTION('',(0.,0.6,-0.8));
#18462=DIRECTION('',(1.,0.,0.));
#18463=DIRECTION('',(0.,0.6,-0.8));
#18464=DIRECTION('center_axis',(1.,0.,0.));
#18465=DIRECTION('ref_axis',(0.,1.,-6.12323399573677E-17));
#18466=DIRECTION('',(0.,0.6,0.8));
#18467=DIRECTION('center_axis',(0.,0.8,-0.6));
#18468=DIRECTION('ref_axis',(0.,0.6,0.8));
#18469=DIRECTION('',(0.,0.6,0.8));
#18470=DIRECTION('center_axis',(1.,0.,0.));
#18471=DIRECTION('ref_axis',(0.,1.,-6.12323399573677E-17));
#18472=DIRECTION('center_axis',(0.,-0.928032088092767,-0.372500259691424));
#18473=DIRECTION('ref_axis',(0.,0.372500259691424,-0.928032088092767));
#18474=DIRECTION('',(0.,0.372500259691424,-0.928032088092767));
#18475=DIRECTION('',(1.,0.,0.));
#18476=DIRECTION('',(0.,0.372500259691424,-0.928032088092767));
#18477=DIRECTION('center_axis',(1.,0.,0.));
#18478=DIRECTION('ref_axis',(0.,0.965925826289068,-0.258819045102521));
#18479=DIRECTION('',(0.,0.786610731855457,0.617449233969742));
#18480=DIRECTION('center_axis',(0.,0.617449233969742,-0.786610731855457));
#18481=DIRECTION('ref_axis',(0.,0.786610731855457,0.617449233969742));
#18482=DIRECTION('',(0.,0.786610731855457,0.617449233969742));
#18483=DIRECTION('center_axis',(1.,0.,0.));
#18484=DIRECTION('ref_axis',(0.,0.965925826289068,-0.258819045102521));
#18485=DIRECTION('center_axis',(0.,-0.992820323027551,-0.119615242270663));
#18486=DIRECTION('ref_axis',(0.,0.119615242270663,-0.992820323027551));
#18487=DIRECTION('',(0.,0.119615242270663,-0.992820323027551));
#18488=DIRECTION('',(1.,0.,0.));
#18489=DIRECTION('',(0.,0.119615242270663,-0.992820323027551));
#18490=DIRECTION('center_axis',(1.,0.,0.));
#18491=DIRECTION('ref_axis',(0.,0.866025403784439,-0.5));
#18492=DIRECTION('',(0.,0.919615242270663,0.392820323027551));
#18493=DIRECTION('center_axis',(0.,0.392820323027551,-0.919615242270663));
#18494=DIRECTION('ref_axis',(0.,0.919615242270663,0.392820323027551));
#18495=DIRECTION('',(0.,0.919615242270663,0.392820323027551));
#18496=DIRECTION('center_axis',(1.,0.,0.));
#18497=DIRECTION('ref_axis',(0.,0.866025403784439,-0.5));
#18498=DIRECTION('center_axis',(0.,-0.989949493661167,0.14142135623731));
#18499=DIRECTION('ref_axis',(0.,-0.14142135623731,-0.989949493661167));
#18500=DIRECTION('',(0.,-0.14142135623731,-0.989949493661167));
#18501=DIRECTION('',(1.,0.,0.));
#18502=DIRECTION('',(0.,-0.14142135623731,-0.989949493661167));
#18503=DIRECTION('center_axis',(1.,0.,0.));
#18504=DIRECTION('ref_axis',(0.,0.707106781186548,-0.707106781186548));
#18505=DIRECTION('',(0.,0.989949493661167,0.14142135623731));
#18506=DIRECTION('center_axis',(0.,0.14142135623731,-0.989949493661167));
#18507=DIRECTION('ref_axis',(0.,0.989949493661167,0.14142135623731));
#18508=DIRECTION('',(0.,0.989949493661167,0.14142135623731));
#18509=DIRECTION('center_axis',(1.,0.,0.));
#18510=DIRECTION('ref_axis',(0.,0.707106781186548,-0.707106781186548));
#18511=DIRECTION('center_axis',(0.,-0.919615242270663,0.392820323027551));
#18512=DIRECTION('ref_axis',(0.,-0.392820323027551,-0.919615242270663));
#18513=DIRECTION('',(0.,-0.392820323027551,-0.919615242270663));
#18514=DIRECTION('',(1.,0.,0.));
#18515=DIRECTION('',(0.,-0.392820323027551,-0.919615242270663));
#18516=DIRECTION('center_axis',(1.,0.,0.));
#18517=DIRECTION('ref_axis',(0.,0.5,-0.866025403784439));
#18518=DIRECTION('',(0.,0.992820323027551,-0.119615242270663));
#18519=DIRECTION('center_axis',(0.,-0.119615242270663,-0.992820323027551));
#18520=DIRECTION('ref_axis',(0.,0.992820323027551,-0.119615242270663));
#18521=DIRECTION('',(0.,0.992820323027551,-0.119615242270663));
#18522=DIRECTION('center_axis',(1.,0.,0.));
#18523=DIRECTION('ref_axis',(0.,0.5,-0.866025403784439));
#18524=DIRECTION('center_axis',(0.,-0.786610731855457,0.617449233969743));
#18525=DIRECTION('ref_axis',(0.,-0.617449233969742,-0.786610731855457));
#18526=DIRECTION('',(0.,-0.617449233969742,-0.786610731855457));
#18527=DIRECTION('',(1.,0.,0.));
#18528=DIRECTION('',(0.,-0.617449233969742,-0.786610731855457));
#18529=DIRECTION('center_axis',(1.,0.,0.));
#18530=DIRECTION('ref_axis',(0.,0.258819045102521,-0.965925826289068));
#18531=DIRECTION('',(0.,0.928032088092767,-0.372500259691424));
#18532=DIRECTION('center_axis',(0.,-0.372500259691424,-0.928032088092767));
#18533=DIRECTION('ref_axis',(0.,0.928032088092767,-0.372500259691424));
#18534=DIRECTION('',(0.,0.928032088092767,-0.372500259691424));
#18535=DIRECTION('center_axis',(1.,0.,0.));
#18536=DIRECTION('ref_axis',(0.,0.258819045102521,-0.965925826289068));
#18537=DIRECTION('center_axis',(0.,-0.6,0.8));
#18538=DIRECTION('ref_axis',(0.,-0.8,-0.6));
#18539=DIRECTION('',(0.,-0.8,-0.6));
#18540=DIRECTION('',(1.,0.,0.));
#18541=DIRECTION('',(0.,-0.8,-0.6));
#18542=DIRECTION('center_axis',(1.,0.,0.));
#18543=DIRECTION('ref_axis',(0.,0.,-1.));
#18544=DIRECTION('',(0.,0.8,-0.6));
#18545=DIRECTION('center_axis',(0.,-0.6,-0.8));
#18546=DIRECTION('ref_axis',(0.,0.8,-0.6));
#18547=DIRECTION('',(0.,0.8,-0.6));
#18548=DIRECTION('center_axis',(1.,0.,0.));
#18549=DIRECTION('ref_axis',(0.,0.,-1.));
#18550=DIRECTION('center_axis',(-1.,0.,0.));
#18551=DIRECTION('ref_axis',(0.,0.,1.));
#18552=DIRECTION('center_axis',(1.,0.,0.));
#18553=DIRECTION('ref_axis',(0.,0.,-1.));
#18554=DIRECTION('center_axis',(1.,0.,0.));
#18555=DIRECTION('ref_axis',(0.,1.,0.));
#18556=DIRECTION('',(-0.707106781186548,0.707106781186548,8.65956056235494E-17));
#18557=DIRECTION('center_axis',(1.,0.,0.));
#18558=DIRECTION('ref_axis',(0.,1.,0.));
#18559=DIRECTION('center_axis',(-1.,0.,0.));
#18560=DIRECTION('ref_axis',(0.,1.,0.));
#18561=DIRECTION('center_axis',(1.,0.,0.));
#18562=DIRECTION('ref_axis',(0.,0.,-1.));
#18563=DIRECTION('',(-0.707106781186549,-0.707106781186546,-8.65956056235491E-17));
#18564=DIRECTION('center_axis',(1.,0.,0.));
#18565=DIRECTION('ref_axis',(0.,0.,-1.));
#18566=DIRECTION('center_axis',(1.,0.,0.));
#18567=DIRECTION('ref_axis',(0.,0.,-1.));
#18568=DIRECTION('center_axis',(1.,0.,0.));
#18569=DIRECTION('ref_axis',(0.,1.,0.));
#18570=DIRECTION('',(-1.,0.,0.));
#18571=DIRECTION('center_axis',(1.,0.,0.));
#18572=DIRECTION('ref_axis',(0.,0.,-1.));
#18573=DIRECTION('center_axis',(1.,0.,0.));
#18574=DIRECTION('ref_axis',(0.,0.,-1.));
#21798=CARTESIAN_POINT('',(0.,0.,0.));
#21799=CARTESIAN_POINT('Origin',(4.7,0.,0.));
#21800=CARTESIAN_POINT('',(-5.40584015536924,-3.95830846622076,0.00274910382348996));
#21801=CARTESIAN_POINT('',(-5.51115984463076,-3.9570708572248,0.00447188352567895));
#21802=CARTESIAN_POINT('',(4.7,-3.954,-4.84225344382863E-16));
#21803=CARTESIAN_POINT('',(-5.646,1.69040986975532,3.57773147777698));
#21804=CARTESIAN_POINT('Ctrl Pts',(-5.40584015536924,-3.95830846622076,
0.00274910382348996));
#21805=CARTESIAN_POINT('Ctrl Pts',(-5.41040414140305,-3.9594161894576,0.153448192401004));
#21806=CARTESIAN_POINT('Ctrl Pts',(-5.41496812743687,-3.9515526888245,0.304023613068971));
#21807=CARTESIAN_POINT('Ctrl Pts',(-5.41953211347068,-3.93433121121586,
0.45351211176479));
#21808=CARTESIAN_POINT('Ctrl Pts',(-5.4591048501247,-3.78500976431612,1.74967492818534));
#21809=CARTESIAN_POINT('Ctrl Pts',(-5.49867758677871,-2.93215360777617,
2.96412271836921));
#21810=CARTESIAN_POINT('Ctrl Pts',(-5.53825032343272,-1.76367516250592,
3.54561744325898));
#21811=CARTESIAN_POINT('Ctrl Pts',(-5.57416688228848,-0.703153995669211,
4.07338709673073));
#21812=CARTESIAN_POINT('Ctrl Pts',(-5.61008344114424,0.617362135119781,
4.07975944947112));
#21813=CARTESIAN_POINT('Ctrl Pts',(-5.646,1.69249901178079,3.58003443294051));
#21814=CARTESIAN_POINT('',(-5.646,-1.6883207277298,3.57542852261347));
#21815=CARTESIAN_POINT('Origin',(-5.646,0.,0.));
#21816=CARTESIAN_POINT('Ctrl Pts',(-5.646,-1.68832072772979,3.57542852261347));
#21817=CARTESIAN_POINT('Ctrl Pts',(-5.60642726334599,-2.87366031862924,
3.01571004745528));
#21818=CARTESIAN_POINT('Ctrl Pts',(-5.56685452669198,-3.74882603463833,
1.82534319022921));
#21819=CARTESIAN_POINT('Ctrl Pts',(-5.52728179003796,-3.92388973907126,
0.534376331785177));
#21820=CARTESIAN_POINT('Ctrl Pts',(-5.52190780823556,-3.94766340855763,
0.359062896542186));
#21821=CARTESIAN_POINT('Ctrl Pts',(-5.51653382643316,-3.95852602877135,
0.18189422941716));
#21822=CARTESIAN_POINT('Ctrl Pts',(-5.51115984463076,-3.9570708572248,0.00447188352567895));
#21823=CARTESIAN_POINT('Origin',(4.7,0.,0.));
#21824=CARTESIAN_POINT('',(-4.65584015536924,-3.94807202781677,0.00139985687555771));
#21825=CARTESIAN_POINT('',(-4.76115984463076,-3.94781927952859,0.001010842389746));
#21826=CARTESIAN_POINT('',(4.7,-3.954,-4.84225344382863E-16));
#21827=CARTESIAN_POINT('Ctrl Pts',(-4.65584015536924,-3.94807202781677,
0.00139985687555771));
#21828=CARTESIAN_POINT('Ctrl Pts',(-4.67296772147897,-3.94988746363517,
0.570738284822051));
#21829=CARTESIAN_POINT('Ctrl Pts',(-4.69009528758871,-3.83478261226913,
1.1393760863107));
#21830=CARTESIAN_POINT('Ctrl Pts',(-4.70722285369845,-3.599099248183,1.65264375078517));
#21831=CARTESIAN_POINT('Ctrl Pts',(-4.74679559035246,-3.05455978233268,
2.83853356076355));
#21832=CARTESIAN_POINT('Ctrl Pts',(-4.78636832700647,-1.86633917166041,
3.72884240545855));
#21833=CARTESIAN_POINT('Ctrl Pts',(-4.82594106366049,-0.575235943424667,
3.91838868771338));
#21834=CARTESIAN_POINT('Ctrl Pts',(-4.8655138003145,0.715867284811076,4.10793496996821));
#21835=CARTESIAN_POINT('Ctrl Pts',(-4.90508653696851,2.10985313061029,3.59671868978285));
#21836=CARTESIAN_POINT('Ctrl Pts',(-4.94465927362253,2.97225595093563,2.61735378803508));
#21837=CARTESIAN_POINT('Ctrl Pts',(-4.98423201027654,3.83465877126098,1.6379888862873));
#21838=CARTESIAN_POINT('Ctrl Pts',(-5.02380474693055,4.16547856611245,0.190475362977117));
#21839=CARTESIAN_POINT('Ctrl Pts',(-5.06337748358456,3.81416626107115,-1.06625514220163));
#21840=CARTESIAN_POINT('Ctrl Pts',(-5.10295022023858,3.46285395602986,-2.32298564738038));
#21841=CARTESIAN_POINT('Ctrl Pts',(-5.14252295689259,2.42940955109579,-3.38893313442769));
#21842=CARTESIAN_POINT('Ctrl Pts',(-5.1820956935466,1.18415546882936,-3.77916117270054));
#21843=CARTESIAN_POINT('Ctrl Pts',(-5.22166843020061,-0.0610986134370675,
-4.16938921097339));
#21844=CARTESIAN_POINT('Ctrl Pts',(-5.26124116685463,-1.51816237303585,
-3.88389780047179));
#21845=CARTESIAN_POINT('Ctrl Pts',(-5.30081390350864,-2.52380088420549,
-3.05221317389238));
#21846=CARTESIAN_POINT('Ctrl Pts',(-5.33582265412884,-3.41345752229485,
-2.31644804495686));
#21847=CARTESIAN_POINT('Ctrl Pts',(-5.37083140474904,-3.94981150626788,
-1.15321122813476));
#21848=CARTESIAN_POINT('Ctrl Pts',(-5.40584015536924,-3.95830846622076,
0.00274910382348996));
#21849=CARTESIAN_POINT('Ctrl Pts',(-5.51115984463076,-3.9570708572248,0.00447188352567895));
#21850=CARTESIAN_POINT('Ctrl Pts',(-5.47696108977915,-3.94781048813209,
-1.12460215048567));
#21851=CARTESIAN_POINT('Ctrl Pts',(-5.44276233492753,-3.43971035750927,
-2.26394954012984));
#21852=CARTESIAN_POINT('Ctrl Pts',(-5.40856358007592,-2.58566274428266,
-3.00082354295664));
#21853=CARTESIAN_POINT('Ctrl Pts',(-5.36899084342191,-1.59741035220436,
-3.85348969959244));
#21854=CARTESIAN_POINT('Ctrl Pts',(-5.3294181067679,-0.145943875190994,
-4.16725515320204));
#21855=CARTESIAN_POINT('Ctrl Pts',(-5.28984537011389,1.10711897366749,-3.80213656168223));
#21856=CARTESIAN_POINT('Ctrl Pts',(-5.25027263345987,2.36018182252598,-3.43701797016241));
#21857=CARTESIAN_POINT('Ctrl Pts',(-5.21069989680586,3.41484104322959,-2.39301533351318));
#21858=CARTESIAN_POINT('Ctrl Pts',(-5.17112716015184,3.79159857088148,-1.14386006663144));
#21859=CARTESIAN_POINT('Ctrl Pts',(-5.13155442349783,4.16835609853338,0.105295200250295));
#21860=CARTESIAN_POINT('Ctrl Pts',(-5.09198168684382,3.86721193313355,1.55960309736453));
#21861=CARTESIAN_POINT('Ctrl Pts',(-5.0524089501898,3.02495731201586,2.55640561878531));
#21862=CARTESIAN_POINT('Ctrl Pts',(-5.01283621353579,2.18270269089815,3.5532081402061));
#21863=CARTESIAN_POINT('Ctrl Pts',(-4.97326347688178,0.799337614062568,
4.09250528593342));
#21864=CARTESIAN_POINT('Ctrl Pts',(-4.93369074022777,-0.495374153645519,
3.92923511481126));
#21865=CARTESIAN_POINT('Ctrl Pts',(-4.89411800357376,-1.7900859213536,3.76596494368911));
#21866=CARTESIAN_POINT('Ctrl Pts',(-4.85454526691974,-2.99614437993419,
2.9001274557175));
#21867=CARTESIAN_POINT('Ctrl Pts',(-4.81497253026573,-3.5647017355765,1.72559158222104));
#21868=CARTESIAN_POINT('Ctrl Pts',(-4.7970349683874,-3.82241787073735,1.19319701741357));
#21869=CARTESIAN_POINT('Ctrl Pts',(-4.77909740650908,-3.94915080627378,
0.597376205861484));
#21870=CARTESIAN_POINT('Ctrl Pts',(-4.76115984463076,-3.94781927952859,
0.001010842389746));
#21871=CARTESIAN_POINT('Origin',(4.7,0.,0.));
#21872=CARTESIAN_POINT('',(-3.90584015536924,-3.95333922947531,-0.00355421683578439));
#21873=CARTESIAN_POINT('',(-4.01115984463076,-3.95413953703022,-0.00354925354858068));
#21874=CARTESIAN_POINT('',(4.7,-3.954,-4.84225344382863E-16));
#21875=CARTESIAN_POINT('Ctrl Pts',(-3.90584015536924,-3.95333922947531,
-0.00355421683578439));
#21876=CARTESIAN_POINT('Ctrl Pts',(-3.9355313015549,-3.94453230977388,0.980091333856488));
#21877=CARTESIAN_POINT('Ctrl Pts',(-3.96522244774056,-3.57263269613905,
1.96968142938521));
#21878=CARTESIAN_POINT('Ctrl Pts',(-3.99491359392622,-2.90796156736813,
2.68858637312984));
#21879=CARTESIAN_POINT('Ctrl Pts',(-4.03448633058023,-2.02207944695739,
3.64675201079778));
#21880=CARTESIAN_POINT('Ctrl Pts',(-4.07405906723424,-0.616121026144095,
4.12407533616519));
#21881=CARTESIAN_POINT('Ctrl Pts',(-4.11363180388825,0.670009230171976,
3.90330920884321));
#21882=CARTESIAN_POINT('Ctrl Pts',(-4.15320454054227,1.95613948648805,3.68254308152123));
#21883=CARTESIAN_POINT('Ctrl Pts',(-4.19277727719628,3.12244157830689,2.76368750150988));
#21884=CARTESIAN_POINT('Ctrl Pts',(-4.23235001385029,3.63808732338842,1.56494695195733));
#21885=CARTESIAN_POINT('Ctrl Pts',(-4.27192275050431,4.15373306846994,0.366206402404782));
#21886=CARTESIAN_POINT('Ctrl Pts',(-4.31149548715832,4.01872246681414,-1.11241911668896));
#21887=CARTESIAN_POINT('Ctrl Pts',(-4.35106822381233,3.29450433464159,-2.19794909096417));
#21888=CARTESIAN_POINT('Ctrl Pts',(-4.39064096046634,2.57028620246903,-3.28347906523937));
#21889=CARTESIAN_POINT('Ctrl Pts',(-4.43021369712036,1.25686053977973,-3.97591349469604));
#21890=CARTESIAN_POINT('Ctrl Pts',(-4.46978643377437,-0.0479839970950056,
-3.96010399035171));
#21891=CARTESIAN_POINT('Ctrl Pts',(-4.50935917042838,-1.35282853396974,
-3.94429448600738));
#21892=CARTESIAN_POINT('Ctrl Pts',(-4.5489319070824,-2.64909194502991,-3.22024104786205));
#21893=CARTESIAN_POINT('Ctrl Pts',(-4.58850464373641,-3.3467944900458,-2.1174789411585));
#21894=CARTESIAN_POINT('Ctrl Pts',(-4.61094981428069,-3.74252281050475,
-1.49200580870543));
#21895=CARTESIAN_POINT('Ctrl Pts',(-4.63339498482496,-3.94569295268753,
-0.744701371448065));
#21896=CARTESIAN_POINT('Ctrl Pts',(-4.65584015536924,-3.94807202781677,
0.00139985687555771));
#21897=CARTESIAN_POINT('Ctrl Pts',(-4.76115984463076,-3.94781927952859,
0.001010842389746));
#21898=CARTESIAN_POINT('Ctrl Pts',(-4.73952466985507,-3.94621327454049,
-0.718288076627242));
#21899=CARTESIAN_POINT('Ctrl Pts',(-4.71788949507938,-3.75830307984049,
-1.43837919281071));
#21900=CARTESIAN_POINT('Ctrl Pts',(-4.69625432030369,-3.3892100636415,-2.04892701679288));
#21901=CARTESIAN_POINT('Ctrl Pts',(-4.65668158364968,-2.71410478336013,
-3.16567548328903));
#21902=CARTESIAN_POINT('Ctrl Pts',(-4.61710884699566,-1.43283797009337,
-3.91593815726002));
#21903=CARTESIAN_POINT('Ctrl Pts',(-4.57753611034165,-0.128583036525032,
-3.95829929255482));
#21904=CARTESIAN_POINT('Ctrl Pts',(-4.53796337368764,1.1756718970433,-4.00066042784961));
#21905=CARTESIAN_POINT('Ctrl Pts',(-4.49839063703363,2.50291495091321,-3.33512002446819));
#21906=CARTESIAN_POINT('Ctrl Pts',(-4.45881790037961,3.24907874340357,-2.26456057724478));
#21907=CARTESIAN_POINT('Ctrl Pts',(-4.4192451637256,3.99524253589392,-1.19400113002136));
#21908=CARTESIAN_POINT('Ctrl Pts',(-4.37967242707158,4.16032706700472,0.281577361044059));
#21909=CARTESIAN_POINT('Ctrl Pts',(-4.34009969041757,3.66919043867727,1.49056783765062));
#21910=CARTESIAN_POINT('Ctrl Pts',(-4.30052695376356,3.17805381034982,2.69955831425719));
#21911=CARTESIAN_POINT('Ctrl Pts',(-4.26095421710955,2.03069602258413,3.6419607764049));
#21912=CARTESIAN_POINT('Ctrl Pts',(-4.22138148045554,0.749325781401231,
3.88886069412444));
#21913=CARTESIAN_POINT('Ctrl Pts',(-4.18180874380152,-0.532044459781662,
4.13576061184399));
#21914=CARTESIAN_POINT('Ctrl Pts',(-4.14223600714751,-1.94742715438175,
3.68715798513539));
#21915=CARTESIAN_POINT('Ctrl Pts',(-4.1026632704935,-2.85262996255091,2.74722438990827));
#21916=CARTESIAN_POINT('Ctrl Pts',(-4.07216212853925,-3.550325438877,2.02275975997274));
#21917=CARTESIAN_POINT('Ctrl Pts',(-4.04166098658501,-3.94493666981705,
1.00640852339343));
#21918=CARTESIAN_POINT('Ctrl Pts',(-4.01115984463076,-3.95413953703022,
-0.00354925354858068));
#21919=CARTESIAN_POINT('Origin',(4.7,0.,0.));
#21920=CARTESIAN_POINT('',(-3.15584015536924,-3.95962261149855,0.00156596972554903));
#21921=CARTESIAN_POINT('',(-3.26115984463076,-3.9591353959144,0.00198372275667011));
#21922=CARTESIAN_POINT('',(4.7,-3.954,-4.84225344382863E-16));
#21923=CARTESIAN_POINT('Ctrl Pts',(-3.15584015536924,-3.95962261149855,
0.00156596972554903));
#21924=CARTESIAN_POINT('Ctrl Pts',(-3.15852214497681,-3.96007009395101,
0.0900527454151371));
#21925=CARTESIAN_POINT('Ctrl Pts',(-3.16120413458437,-3.95735922725396,
0.178511619278897));
#21926=CARTESIAN_POINT('Ctrl Pts',(-3.16388612419194,-3.951402336726,0.26675136050462));
#21927=CARTESIAN_POINT('Ctrl Pts',(-3.20345886084596,-3.86350846141984,
1.56872808408672));
#21928=CARTESIAN_POINT('Ctrl Pts',(-3.24303159749997,-3.06892337125733,
2.82299748379964));
#21929=CARTESIAN_POINT('Ctrl Pts',(-3.28260433415398,-1.92929263952253,
3.4586943546257));
#21930=CARTESIAN_POINT('Ctrl Pts',(-3.32217707080799,-0.789661907787753,
4.09439122545175));
#21931=CARTESIAN_POINT('Ctrl Pts',(-3.36174980746201,0.695014465519304,
4.11151556739096));
#21932=CARTESIAN_POINT('Ctrl Pts',(-3.40132254411602,1.84900440207876,3.50227346215549));
#21933=CARTESIAN_POINT('Ctrl Pts',(-3.44089528077003,3.00299433863823,2.89303135692001));
#21934=CARTESIAN_POINT('Ctrl Pts',(-3.48046801742405,3.82629783845009,1.65742280450983));
#21935=CARTESIAN_POINT('Ctrl Pts',(-3.52004075407806,3.94419849611561,0.357819722064362));
#21936=CARTESIAN_POINT('Ctrl Pts',(-3.55961349073207,4.06209915378113,-0.941783360381109));
#21937=CARTESIAN_POINT('Ctrl Pts',(-3.59918622738609,3.47459696930029,-2.30538097286188));
#21938=CARTESIAN_POINT('Ctrl Pts',(-3.6387589640401,2.4490863012015,-3.11234848363658));
#21939=CARTESIAN_POINT('Ctrl Pts',(-3.67833170069411,1.4235756331027,-3.91931599441128));
#21940=CARTESIAN_POINT('Ctrl Pts',(-3.71790443734813,-0.0399435186140502,
-4.16965340347993));
#21941=CARTESIAN_POINT('Ctrl Pts',(-3.75747717400214,-1.27536853738317,
-3.74942283333533));
#21942=CARTESIAN_POINT('Ctrl Pts',(-3.79704991065615,-2.51079355615229,
-3.32919226319073));
#21943=CARTESIAN_POINT('Ctrl Pts',(-3.83662264731016,-3.51812444197377,
-2.23839371383289));
#21944=CARTESIAN_POINT('Ctrl Pts',(-3.87619538396417,-3.83888697488042,
-0.973490464169738));
#21945=CARTESIAN_POINT('Ctrl Pts',(-3.88607697443253,-3.91898363373643,
-0.657635232712209));
#21946=CARTESIAN_POINT('Ctrl Pts',(-3.89595856490088,-3.95627028418209,
-0.330923946423857));
#21947=CARTESIAN_POINT('Ctrl Pts',(-3.90584015536924,-3.95333922947531,
-0.00355421683578439));
#21948=CARTESIAN_POINT('Ctrl Pts',(-4.01115984463076,-3.95413953703022,
-0.00354925354858068));
#21949=CARTESIAN_POINT('Ctrl Pts',(-4.00208824993099,-3.95687663722007,
-0.303929076377534));
#21950=CARTESIAN_POINT('Ctrl Pts',(-3.99301665523123,-3.92552144433661,
-0.603743349207523));
#21951=CARTESIAN_POINT('Ctrl Pts',(-3.98394506053146,-3.85790810174668,
-0.895144652921099));
#21952=CARTESIAN_POINT('Ctrl Pts',(-3.94437232387744,-3.56296051103506,
-2.16631553677773));
#21953=CARTESIAN_POINT('Ctrl Pts',(-3.90479958722343,-2.57804240787361,
-3.27739274074537));
#21954=CARTESIAN_POINT('Ctrl Pts',(-3.86522685056942,-1.35142751700913,
-3.72268442840996));
#21955=CARTESIAN_POINT('Ctrl Pts',(-3.82565411391541,-0.12481262614466,
-4.16797611607455));
#21956=CARTESIAN_POINT('Ctrl Pts',(-3.78608137726139,1.34349905242283,-3.94748228743609));
#21957=CARTESIAN_POINT('Ctrl Pts',(-3.74650864060738,2.3852238560361,-3.16155734667935));
#21958=CARTESIAN_POINT('Ctrl Pts',(-3.70693590395337,3.42694865964938,-2.37563240592262));
#21959=CARTESIAN_POINT('Ctrl Pts',(-3.66736316729935,4.04208658830845,-1.02427635304761));
#21960=CARTESIAN_POINT('Ctrl Pts',(-3.62779043064534,3.95066510436862,0.27745749225628));
#21961=CARTESIAN_POINT('Ctrl Pts',(-3.58821769399133,3.85924362042878,1.57919133756016));
#21962=CARTESIAN_POINT('Ctrl Pts',(-3.54864495733732,3.06126272389006,2.83130297529291));
#21963=CARTESIAN_POINT('Ctrl Pts',(-3.5090722206833,1.91991360954393,3.4639094616809));
#21964=CARTESIAN_POINT('Ctrl Pts',(-3.46949948402929,0.7785644951978,4.09651594806888));
#21965=CARTESIAN_POINT('Ctrl Pts',(-3.42992674737528,-0.706152836955741,
4.10961728311208));
#21966=CARTESIAN_POINT('Ctrl Pts',(-3.39035401072126,-1.85848769767767,
3.49725046416115));
#21967=CARTESIAN_POINT('Ctrl Pts',(-3.35078127406725,-3.01082255839962,
2.88488364521021));
#21968=CARTESIAN_POINT('Ctrl Pts',(-3.31120853741323,-3.83077494768995,
1.64704867226511));
#21969=CARTESIAN_POINT('Ctrl Pts',(-3.27163580075922,-3.94515366365166,
0.347130865392129));
#21970=CARTESIAN_POINT('Ctrl Pts',(-3.26814381538307,-3.95524669327894,
0.232423257184699));
#21971=CARTESIAN_POINT('Ctrl Pts',(-3.26465183000691,-3.95984564225403,
0.117232229442771));
#21972=CARTESIAN_POINT('Ctrl Pts',(-3.26115984463076,-3.9591353959144,0.00198372275667011));
#21973=CARTESIAN_POINT('Origin',(4.7,0.,0.));
#21974=CARTESIAN_POINT('',(-2.40584015536924,-3.94895503742539,0.00226341524845186));
#21975=CARTESIAN_POINT('',(-2.51115984463076,-3.94852321086993,0.00190807621368246));
#21976=CARTESIAN_POINT('',(4.7,-3.954,-4.84225344382863E-16));
#21977=CARTESIAN_POINT('Ctrl Pts',(-2.40584015536924,-3.94895503742539,
0.00226341524845186));
#21978=CARTESIAN_POINT('Ctrl Pts',(-2.42108572505273,-3.95161164091452,
0.508757332831716));
#21979=CARTESIAN_POINT('Ctrl Pts',(-2.43633129473622,-3.86116503322235,
1.0143385318084));
#21980=CARTESIAN_POINT('Ctrl Pts',(-2.45157686441971,-3.67321498688243,
1.48061756513418));
#21981=CARTESIAN_POINT('Ctrl Pts',(-2.49114960107372,-3.18535537636404,
2.69093228450277));
#21982=CARTESIAN_POINT('Ctrl Pts',(-2.53072233772774,-2.04055715558632,
3.63644495749262));
#21983=CARTESIAN_POINT('Ctrl Pts',(-2.57029507438175,-0.759861069646289,
3.88681719010075));
#21984=CARTESIAN_POINT('Ctrl Pts',(-2.60986781103576,0.520835016293738,
4.13718942270888));
#21985=CARTESIAN_POINT('Ctrl Pts',(-2.64944054768977,1.93742896739607,3.69242121493529));
#21986=CARTESIAN_POINT('Ctrl Pts',(-2.68901328434379,2.84517557503799,2.75494331352305));
#21987=CARTESIAN_POINT('Ctrl Pts',(-2.7285860209978,3.7529221826799,1.81746541211081));
#21988=CARTESIAN_POINT('Ctrl Pts',(-2.76815875765182,4.15182144686141,0.387277817059935));
#21989=CARTESIAN_POINT('Ctrl Pts',(-2.80773149430583,3.86031930315829,-0.884687284678487));
#21990=CARTESIAN_POINT('Ctrl Pts',(-2.84730423095984,3.56881715945518,-2.15665238641692));
#21991=CARTESIAN_POINT('Ctrl Pts',(-2.88687696761385,2.58691360786742,-3.27039499484289));
#21992=CARTESIAN_POINT('Ctrl Pts',(-2.92644970426786,1.3615099005383,-3.71900894150773));
#21993=CARTESIAN_POINT('Ctrl Pts',(-2.96602244092188,0.136106193209184,
-4.16762288817257));
#21994=CARTESIAN_POINT('Ctrl Pts',(-3.00559517757589,-1.3327976698613,-3.95110817307629));
#21995=CARTESIAN_POINT('Ctrl Pts',(-3.0451679142299,-2.37664827117163,-3.16800879180251));
#21996=CARTESIAN_POINT('Ctrl Pts',(-3.08205866127635,-3.34975328596754,
-2.43798292982139));
#21997=CARTESIAN_POINT('Ctrl Pts',(-3.11894940832279,-3.95346749370281,
-1.21556896983858));
#21998=CARTESIAN_POINT('Ctrl Pts',(-3.15584015536924,-3.95962261149855,
0.00156596972554903));
#21999=CARTESIAN_POINT('Ctrl Pts',(-3.26115984463076,-3.9591353959144,0.00198372275667011));
#22000=CARTESIAN_POINT('Ctrl Pts',(-3.2250790933529,-3.9517968137711,-1.18881528037774));
#22001=CARTESIAN_POINT('Ctrl Pts',(-3.18899834207504,-3.37765148143732,
-2.38575070374499));
#22002=CARTESIAN_POINT('Ctrl Pts',(-3.15291759079718,-2.44064387050199,
-3.11897334347904));
#22003=CARTESIAN_POINT('Ctrl Pts',(-3.11334485414317,-1.41295031875755,
-3.92315910467638));
#22004=CARTESIAN_POINT('Ctrl Pts',(-3.07377211748916,0.051241827364419,
-4.16952998627021));
#22005=CARTESIAN_POINT('Ctrl Pts',(-3.03419938083514,1.28552363453667,-3.74595331657321));
#22006=CARTESIAN_POINT('Ctrl Pts',(-2.99462664418113,2.51980544170892,-3.32237664687621));
#22007=CARTESIAN_POINT('Ctrl Pts',(-2.95505390752712,3.52417690993145,-2.22885242588837));
#22008=CARTESIAN_POINT('Ctrl Pts',(-2.91548117087311,3.84151079044162,-0.963084679153289));
#22009=CARTESIAN_POINT('Ctrl Pts',(-2.87590843421909,4.15884467095179,0.302683067581793));
#22010=CARTESIAN_POINT('Ctrl Pts',(-2.83633569756508,3.78914096374961,1.74069434006411));
#22011=CARTESIAN_POINT('Ctrl Pts',(-2.79676296091107,2.90066573799585,2.69645610450251));
#22012=CARTESIAN_POINT('Ctrl Pts',(-2.75719022425705,2.01219051224209,3.6522178689409));
#22013=CARTESIAN_POINT('Ctrl Pts',(-2.71761748760304,0.604943767936768,
4.12573012533537));
#22014=CARTESIAN_POINT('Ctrl Pts',(-2.67804475094903,-0.680583552468711,
3.90147962722707));
#22015=CARTESIAN_POINT('Ctrl Pts',(-2.63847201429502,-1.96611087287421,
3.67722912911877));
#22016=CARTESIAN_POINT('Ctrl Pts',(-2.598899277641,-3.12991876937986,2.75521587650767));
#22017=CARTESIAN_POINT('Ctrl Pts',(-2.55932654098699,-3.64231447785219,
1.55508279384779));
#22018=CARTESIAN_POINT('Ctrl Pts',(-2.54327097553491,-3.85020515032875,
1.06816131989674));
#22019=CARTESIAN_POINT('Ctrl Pts',(-2.52721541008284,-3.95086616481225,
0.535458242830061));
#22020=CARTESIAN_POINT('Ctrl Pts',(-2.51115984463076,-3.94852321086993,
0.00190807621368246));
#22021=CARTESIAN_POINT('Origin',(4.7,0.,0.));
#22022=CARTESIAN_POINT('',(-1.65584015536924,-3.95156722446408,-0.00334773101343278));
#22023=CARTESIAN_POINT('',(-1.76115984463076,-3.95230955109532,-0.00347299664959956));
#22024=CARTESIAN_POINT('',(4.7,-3.954,-4.84225344382863E-16));
#22025=CARTESIAN_POINT('Ctrl Pts',(-1.65584015536924,-3.95156722446408,
-0.00334773101343277));
#22026=CARTESIAN_POINT('Ctrl Pts',(-1.68364930512865,-3.94407310588175,
0.918999373347058));
#22027=CARTESIAN_POINT('Ctrl Pts',(-1.71145845488806,-3.62183865226459,
1.84606618164852));
#22028=CARTESIAN_POINT('Ctrl Pts',(-1.73926760464748,-3.03183124106019,
2.54808477877248));
#22029=CARTESIAN_POINT('Ctrl Pts',(-1.77884034130149,-2.19224397897198,
3.54706523342667));
#22030=CARTESIAN_POINT('Ctrl Pts',(-1.8184130779555,-0.810426814979439,
4.09033174829379));
#22031=CARTESIAN_POINT('Ctrl Pts',(-1.85798581460952,0.484703266587122,
3.93062329121606));
#22032=CARTESIAN_POINT('Ctrl Pts',(-1.89755855126353,1.77983334815371,3.77091483413833));
#22033=CARTESIAN_POINT('Ctrl Pts',(-1.93713128791754,2.98827634729431,2.90823140511572));
#22034=CARTESIAN_POINT('Ctrl Pts',(-1.97670402457155,3.56002438557403,1.73521269249398));
#22035=CARTESIAN_POINT('Ctrl Pts',(-2.01627676122557,4.13177242385376,0.562193979872254));
#22036=CARTESIAN_POINT('Ctrl Pts',(-2.05584949787958,4.06682550127261,-0.921160016348606));
#22037=CARTESIAN_POINT('Ctrl Pts',(-2.09542223453359,3.39474340602312,-2.03971907902412));
#22038=CARTESIAN_POINT('Ctrl Pts',(-2.13499497118761,2.72266131077363,-3.15827814169962));
#22039=CARTESIAN_POINT('Ctrl Pts',(-2.17456770784162,1.4434440428558,-3.91204227082979));
#22040=CARTESIAN_POINT('Ctrl Pts',(-2.21414044449563,0.139311513420746,
-3.95794504968973));
#22041=CARTESIAN_POINT('Ctrl Pts',(-2.25371318114964,-1.16482101601431,
-4.00384782854967));
#22042=CARTESIAN_POINT('Ctrl Pts',(-2.29328591780366,-2.49386880696661,
-3.34188925713937));
#22043=CARTESIAN_POINT('Ctrl Pts',(-2.33285865445767,-3.24293220231323,
-2.27335158856057));
#22044=CARTESIAN_POINT('Ctrl Pts',(-2.35718582142819,-3.70341565205352,
-1.61647272508745));
#22045=CARTESIAN_POINT('Ctrl Pts',(-2.38151298839871,-3.94471592809748,
-0.805942664183553));
#22046=CARTESIAN_POINT('Ctrl Pts',(-2.40584015536924,-3.94895503742539,
0.00226341524845186));
#22047=CARTESIAN_POINT('Ctrl Pts',(-2.51115984463076,-3.94852321086993,
0.00190807621368246));
#22048=CARTESIAN_POINT('Ctrl Pts',(-2.48764267342882,-3.9450914009381,-0.77960227610563));
#22049=CARTESIAN_POINT('Ctrl Pts',(-2.46412550222689,-3.72066944546383,
-1.56293001901423));
#22050=CARTESIAN_POINT('Ctrl Pts',(-2.44060833102495,-3.28853666992144,
-2.20686742270246));
#22051=CARTESIAN_POINT('Ctrl Pts',(-2.40103559437094,-2.56137963307938,
-3.2904316438842));
#22052=CARTESIAN_POINT('Ctrl Pts',(-2.36146285771693,-1.24608203895624,
-3.979307173539));
#22053=CARTESIAN_POINT('Ctrl Pts',(-2.32189012106291,0.058714687369509,
-3.95996083783634));
#22054=CARTESIAN_POINT('Ctrl Pts',(-2.2823173844089,1.36351141369524,-3.94061450213368));
#22055=CARTESIAN_POINT('Ctrl Pts',(-2.24274464775489,2.6578072722236,-3.21304630107356));
#22056=CARTESIAN_POINT('Ctrl Pts',(-2.20317191110087,3.3525195178114,-2.10839989898019));
#22057=CARTESIAN_POINT('Ctrl Pts',(-2.16359917444686,4.04723176339921,-1.0037534968868));
#22058=CARTESIAN_POINT('Ctrl Pts',(-2.12402643779285,4.14236039604643,0.477971106239855));
#22059=CARTESIAN_POINT('Ctrl Pts',(-2.08445370113883,3.59460879570253,1.6623852914272));
#22060=CARTESIAN_POINT('Ctrl Pts',(-2.04488096448482,3.04685719535864,2.84679947661452));
#22061=CARTESIAN_POINT('Ctrl Pts',(-2.00530822783081,1.85622536202364,3.73390324386254));
#22062=CARTESIAN_POINT('Ctrl Pts',(-1.9657354911768,0.564614642387913,3.91994229001148));
#22063=CARTESIAN_POINT('Ctrl Pts',(-1.92616275452278,-0.72699607724783,
4.10598133616041));
#22064=CARTESIAN_POINT('Ctrl Pts',(-1.88659001786877,-2.1195856831843,3.59095566121024));
#22065=CARTESIAN_POINT('Ctrl Pts',(-1.84701728121476,-2.97933424742549,
2.60927282848582));
#22066=CARTESIAN_POINT('Ctrl Pts',(-1.81839813568676,-3.60110750239726,
1.89931627183638));
#22067=CARTESIAN_POINT('Ctrl Pts',(-1.78977899015876,-3.94419240060798,
0.94528708133517));
#22068=CARTESIAN_POINT('Ctrl Pts',(-1.76115984463076,-3.95230955109532,
-0.00347299664959956));
#22069=CARTESIAN_POINT('Origin',(4.7,0.,0.));
#22070=CARTESIAN_POINT('',(-0.905840155369234,-3.960321004907,0.000484847720224144));
#22071=CARTESIAN_POINT('',(-1.01115984463075,-3.9601030984513,0.000964724550051354));
#22072=CARTESIAN_POINT('',(4.7,-3.954,-4.84225344382863E-16));
#22073=CARTESIAN_POINT('Ctrl Pts',(-0.905840155369234,-3.960321004907,0.000484847720224144));
#22074=CARTESIAN_POINT('Ctrl Pts',(-0.906640148550558,-3.96036688714869,
0.0268665595925369));
#22075=CARTESIAN_POINT('Ctrl Pts',(-0.907440141731881,-3.96012592613957,
0.0532474112658711));
#22076=CARTESIAN_POINT('Ctrl Pts',(-0.908240134913205,-3.95959555770559,
0.0796224433230482));
#22077=CARTESIAN_POINT('Ctrl Pts',(-0.947812871567218,-3.93336017113319,
1.38429881083044));
#22078=CARTESIAN_POINT('Ctrl Pts',(-0.987385608221231,-3.19896824808949,
2.67473504879244));
#22079=CARTESIAN_POINT('Ctrl Pts',(-1.02695834487524,-2.09066918537765,
3.36360507066375));
#22080=CARTESIAN_POINT('Ctrl Pts',(-1.06653108152926,-0.982370122665806,
4.05247509253507));
#22081=CARTESIAN_POINT('Ctrl Pts',(-1.10610381818327,0.499836079714179,
4.13977889831569));
#22082=CARTESIAN_POINT('Ctrl Pts',(-1.14567655483728,1.68134160877037,3.58578124105477));
#22083=CARTESIAN_POINT('Ctrl Pts',(-1.1852492914913,2.86284713782654,3.03178358379385));
#22084=CARTESIAN_POINT('Ctrl Pts',(-1.22482202814531,3.74365199355893,1.83648446349142));
#22085=CARTESIAN_POINT('Ctrl Pts',(-1.26439476479932,3.92286874448592,0.543909484765631));
#22086=CARTESIAN_POINT('Ctrl Pts',(-1.30396750145333,4.1020854954129,-0.748665493960175));
#22087=CARTESIAN_POINT('Ctrl Pts',(-1.34354023810735,3.57971414153446,-2.13851633110934));
#22088=CARTESIAN_POINT('Ctrl Pts',(-1.38311297476136,2.5935055410265,-2.99306961541944));
#22089=CARTESIAN_POINT('Ctrl Pts',(-1.42268571141537,1.60729694051856,-3.84762289972953));
#22090=CARTESIAN_POINT('Ctrl Pts',(-1.46225844806939,0.157251093381126,
-4.16687863120059));
#22091=CARTESIAN_POINT('Ctrl Pts',(-1.5018311847234,-1.09666157514756,-3.80553151395158));
#22092=CARTESIAN_POINT('Ctrl Pts',(-1.54140392137741,-2.35057424367627,
-3.44418439670257));
#22093=CARTESIAN_POINT('Ctrl Pts',(-1.58097665803143,-3.40835373359622,
-2.40223443073346));
#22094=CARTESIAN_POINT('Ctrl Pts',(-1.62054939468544,-3.78856479846426,
-1.15391225052825));
#22095=CARTESIAN_POINT('Ctrl Pts',(-1.63231298158004,-3.90158821503936,
-0.782829841755529));
#22096=CARTESIAN_POINT('Ctrl Pts',(-1.64407656847464,-3.95473732192856,
-0.393511055063059));
#22097=CARTESIAN_POINT('Ctrl Pts',(-1.65584015536924,-3.95156722446408,
-0.00334773101343277));
#22098=CARTESIAN_POINT('Ctrl Pts',(-1.76115984463076,-3.95230955109532,
-0.00347299664959956));
#22099=CARTESIAN_POINT('Ctrl Pts',(-1.75020625350475,-3.95541628073054,
-0.366598092776724));
#22100=CARTESIAN_POINT('Ctrl Pts',(-1.73925266237873,-3.90945451756587,
-0.728951331280733));
#22101=CARTESIAN_POINT('Ctrl Pts',(-1.72829907125272,-3.81126890115824,
-1.07655311732514));
#22102=CARTESIAN_POINT('Ctrl Pts',(-1.68872633459871,-3.45654746810388,
-2.33235623991302));
#22103=CARTESIAN_POINT('Ctrl Pts',(-1.64915359794469,-2.42019707944922,
-3.39562249459013));
#22104=CARTESIAN_POINT('Ctrl Pts',(-1.60958086129068,-1.17389979134669,
-3.78241940181823));
#22105=CARTESIAN_POINT('Ctrl Pts',(-1.57000812463667,0.0723974967558526,
-4.16921630904633));
#22106=CARTESIAN_POINT('Ctrl Pts',(-1.53043538798265,1.52864168430628,-3.87954386882542));
#22107=CARTESIAN_POINT('Ctrl Pts',(-1.49086265132864,2.53204124812124,-3.04524290807442));
#22108=CARTESIAN_POINT('Ctrl Pts',(-1.45128991467463,3.5354408119362,-2.21094194732342));
#22109=CARTESIAN_POINT('Ctrl Pts',(-1.41171717802061,4.08599575201568,-0.832012466042327));
#22110=CARTESIAN_POINT('Ctrl Pts',(-1.3721444413666,3.93312779965345,0.463942844496236));
#22111=CARTESIAN_POINT('Ctrl Pts',(-1.33257170471259,3.78025984729122,1.75989815503479));
#22112=CARTESIAN_POINT('Ctrl Pts',(-1.29299896805858,2.92396900248728,2.97287929483081));
#22113=CARTESIAN_POINT('Ctrl Pts',(-1.25342623140456,1.75398544797205,3.55081290688068));
#22114=CARTESIAN_POINT('Ctrl Pts',(-1.21385349475055,0.584001893456819,
4.12874651893055));
#22115=CARTESIAN_POINT('Ctrl Pts',(-1.17428075809654,-0.899674370769732,
4.07163260323425));
#22116=CARTESIAN_POINT('Ctrl Pts',(-1.13470802144252,-2.02176645125577,
3.40546585182457));
#22117=CARTESIAN_POINT('Ctrl Pts',(-1.09513528478851,-3.14385853174181,
2.73929910041489));
#22118=CARTESIAN_POINT('Ctrl Pts',(-1.0555625481345,-3.90436642848736,1.46407951329185));
#22119=CARTESIAN_POINT('Ctrl Pts',(-1.01598981148048,-3.95715438240394,
0.160207506653819));
#22120=CARTESIAN_POINT('Ctrl Pts',(-1.01437982253057,-3.95930202317079,
0.107160391385077));
#22121=CARTESIAN_POINT('Ctrl Pts',(-1.01276983358066,-3.96027823741067,
0.0540658502883357));
#22122=CARTESIAN_POINT('Ctrl Pts',(-1.01115984463075,-3.9601030984513,0.000964724550051354));
#22123=CARTESIAN_POINT('Origin',(4.7,0.,0.));
#22124=CARTESIAN_POINT('',(-0.155840155369234,-3.95023180461977,0.00295067076493905));
#22125=CARTESIAN_POINT('',(-0.26115984463076,-3.94963863249541,0.00268116949869843));
#22126=CARTESIAN_POINT('',(4.7,-3.954,-4.84225344382863E-16));
#22127=CARTESIAN_POINT('Ctrl Pts',(-0.155840155369234,-3.95023180461977,
0.00295067076493905));
#22128=CARTESIAN_POINT('Ctrl Pts',(-0.16920372862648,-3.95333112739324,
0.446559495418593));
#22129=CARTESIAN_POINT('Ctrl Pts',(-0.182567301883726,-3.88435259221191,
0.889232777547541));
#22130=CARTESIAN_POINT('Ctrl Pts',(-0.195930875140972,-3.73911347548015,
1.30528431062562));
#22131=CARTESIAN_POINT('Ctrl Pts',(-0.235503611794985,-3.30902571319913,
2.53731240940301));
#22132=CARTESIAN_POINT('Ctrl Pts',(-0.275076348448997,-2.21021368105769,
3.53589605582361));
#22133=CARTESIAN_POINT('Ctrl Pts',(-0.314649085103011,-0.94278807937667,
3.84654225915534));
#22134=CARTESIAN_POINT('Ctrl Pts',(-0.354221821757024,0.324637522304346,
4.15718846248707));
#22135=CARTESIAN_POINT('Ctrl Pts',(-0.393794558411038,1.76067669352494,
3.77989722272996));
#22136=CARTESIAN_POINT('Ctrl Pts',(-0.433367295065051,2.71173397427943,
2.88638797926082));
#22137=CARTESIAN_POINT('Ctrl Pts',(-0.472940031719063,3.6627912550339,1.99287873579169));
#22138=CARTESIAN_POINT('Ctrl Pts',(-0.512512768373075,4.12886664532228,
0.583151488610541));
#22139=CARTESIAN_POINT('Ctrl Pts',(-0.552085505027088,3.89783169822067,
-0.701173848933898));
#22140=CARTESIAN_POINT('Ctrl Pts',(-0.5916582416811,3.66679675111907,-1.98549918647834));
#22141=CARTESIAN_POINT('Ctrl Pts',(-0.631230978335113,2.7386514666275,-3.14442261438607));
#22142=CARTESIAN_POINT('Ctrl Pts',(-0.670803714989126,1.53582968661237,
-3.6504744743393));
#22143=CARTESIAN_POINT('Ctrl Pts',(-0.710376451643139,0.333007906597224,
-4.15652633429253));
#22144=CARTESIAN_POINT('Ctrl Pts',(-0.749949188297152,-1.14449036894149,
-4.00970662629123));
#22145=CARTESIAN_POINT('Ctrl Pts',(-0.789521924951166,-2.22420008166029,
-3.27683852376418));
#22146=CARTESIAN_POINT('Ctrl Pts',(-0.828294668423855,-3.2820826355567,
-2.55878591125383));
#22147=CARTESIAN_POINT('Ctrl Pts',(-0.867067411896545,-3.95809726046985,
-1.27814023393776));
#22148=CARTESIAN_POINT('Ctrl Pts',(-0.905840155369234,-3.960321004907,0.000484847720224144));
#22149=CARTESIAN_POINT('Ctrl Pts',(-1.01115984463075,-3.9601030984513,0.000964724550051354));
#22150=CARTESIAN_POINT('Ctrl Pts',(-0.97319709692665,-3.95597340791621,
-1.25113370713065));
#22151=CARTESIAN_POINT('Ctrl Pts',(-0.935234349222548,-3.31169915783721,
-2.50689315478987));
#22152=CARTESIAN_POINT('Ctrl Pts',(-0.897271601518446,-2.29044260664442,
-3.23088376718121));
#22153=CARTESIAN_POINT('Ctrl Pts',(-0.857698864864433,-1.22587486588073,
-3.9855786082252));
#22154=CARTESIAN_POINT('Ctrl Pts',(-0.81812612821042,0.248328626734209,
-4.16244386416014));
#22155=CARTESIAN_POINT('Ctrl Pts',(-0.778553391556407,1.46120239253684,
-3.68098150218274));
#22156=CARTESIAN_POINT('Ctrl Pts',(-0.738980654902394,2.67407615833947,
-3.19951914020535));
#22157=CARTESIAN_POINT('Ctrl Pts',(-0.699407918248381,3.62562019732977,
-2.05972916031563));
#22158=CARTESIAN_POINT('Ctrl Pts',(-0.659835181594368,3.88275101405482,
-0.780372868712951));
#22159=CARTESIAN_POINT('Ctrl Pts',(-0.620262444940355,4.13988183077987,
0.498983422889739));
#22160=CARTESIAN_POINT('Ctrl Pts',(-0.580689708286341,3.70259942523967,
1.9179060262054));
#22161=CARTESIAN_POINT('Ctrl Pts',(-0.541116971632328,2.76992747361883,
2.83058987531903));
#22162=CARTESIAN_POINT('Ctrl Pts',(-0.501544234978315,1.83725552199801,
3.74327372443265));
#22163=CARTESIAN_POINT('Ctrl Pts',(-0.461971498324304,0.409194024296591,
4.14971881934427));
#22164=CARTESIAN_POINT('Ctrl Pts',(-0.422398761670291,-0.864292498870581,
3.8649367042376));
#22165=CARTESIAN_POINT('Ctrl Pts',(-0.382826025016278,-2.13777902203777,
3.58015458913094));
#22166=CARTESIAN_POINT('Ctrl Pts',(-0.343253288362265,-3.25669057067071,
2.60414526400595));
#22167=CARTESIAN_POINT('Ctrl Pts',(-0.303680551708251,-3.71176839821802,
1.3811272965795));
#22168=CARTESIAN_POINT('Ctrl Pts',(-0.289506982682421,-3.87476134604623,
0.943085072391007));
#22169=CARTESIAN_POINT('Ctrl Pts',(-0.27533341365659,-3.95259626783404,
0.473356045129417));
#22170=CARTESIAN_POINT('Ctrl Pts',(-0.26115984463076,-3.94963863249541,
0.00268116949869843));
#22171=CARTESIAN_POINT('Origin',(4.7,0.,0.));
#22172=CARTESIAN_POINT('',(0.594159844630767,-3.95001826622686,-0.00286169934786473));
#22173=CARTESIAN_POINT('',(0.488840155369245,-3.95065042271477,-0.00310251149715996));
#22174=CARTESIAN_POINT('',(4.7,-3.954,-4.84225344382863E-16));
#22175=CARTESIAN_POINT('Ctrl Pts',(0.594159844630767,-3.95001826622686,
-0.00286169934786473));
#22176=CARTESIAN_POINT('Ctrl Pts',(0.568232691297599,-3.94420741043142,
0.857917096057318));
#22177=CARTESIAN_POINT('Ctrl Pts',(0.54230553796443,-3.6674357688023,1.72209758997099));
#22178=CARTESIAN_POINT('Ctrl Pts',(0.516378384631261,-3.14891915370461,
2.40188361031813));
#22179=CARTESIAN_POINT('Ctrl Pts',(0.476805647977248,-2.35750479377407,
3.43944422557712));
#22180=CARTESIAN_POINT('Ctrl Pts',(0.437232911323236,-1.00291986527977,
4.04743834756636));
#22181=CARTESIAN_POINT('Ctrl Pts',(0.397660174669223,0.29831306247853,3.9491449746543));
#22182=CARTESIAN_POINT('Ctrl Pts',(0.35808743801521,1.59954599023685,3.85085160174224));
#22183=CARTESIAN_POINT('Ctrl Pts',(0.318514701361196,2.84742691725918,3.04627073392885));
#22184=CARTESIAN_POINT('Ctrl Pts',(0.278941964707183,3.47399828021787,1.90159739774904));
#22185=CARTESIAN_POINT('Ctrl Pts',(0.23936922805317,4.10056964317655,0.756924061569239));
#22186=CARTESIAN_POINT('Ctrl Pts',(0.199796491399158,4.1058314420716,-0.727841742976961));
#22187=CARTESIAN_POINT('Ctrl Pts',(0.160223754745145,3.48738883424261,-1.87692723164287));
#22188=CARTESIAN_POINT('Ctrl Pts',(0.120651018091132,2.86894622641362,-3.02601272030878));
#22189=CARTESIAN_POINT('Ctrl Pts',(0.0810782814371191,1.62679921186058,
-3.83941789309439));
#22190=CARTESIAN_POINT('Ctrl Pts',(0.0415055447831063,0.326295634599078,
-3.94693145024388));
#22191=CARTESIAN_POINT('Ctrl Pts',(0.00193280812909338,-0.974207942662425,
-4.05444500739337));
#22192=CARTESIAN_POINT('Ctrl Pts',(-0.0376399285249198,-2.33306808263239,
-3.45606694890674));
#22193=CARTESIAN_POINT('Ctrl Pts',(-0.0772126651789329,-3.13181640640708,
-2.42414164409634));
#22194=CARTESIAN_POINT('Ctrl Pts',(-0.1034218285757,-3.66083024524608,-1.7406938663119));
#22195=CARTESIAN_POINT('Ctrl Pts',(-0.129630991972467,-3.94415329137893,
-0.867072334743039));
#22196=CARTESIAN_POINT('Ctrl Pts',(-0.155840155369234,-3.95023180461977,
0.00295067076493905));
#22197=CARTESIAN_POINT('Ctrl Pts',(-0.26115984463076,-3.94963863249541,
0.00268116949869843));
#22198=CARTESIAN_POINT('Ctrl Pts',(-0.235760677002577,-3.94433852243758,
-0.840772588882956));
#22199=CARTESIAN_POINT('Ctrl Pts',(-0.210361509374395,-3.67958948684631,
-1.68726374763685));
#22200=CARTESIAN_POINT('Ctrl Pts',(-0.184962341746213,-3.18051337951411,
-2.35988811050413));
#22201=CARTESIAN_POINT('Ctrl Pts',(-0.1453896050922,-2.40293642680116,-3.40785894043344));
#22202=CARTESIAN_POINT('Ctrl Pts',(-0.105816868438186,-1.05653841491356,
-4.03377399056417));
#22203=CARTESIAN_POINT('Ctrl Pts',(-0.0662441317841735,0.245884260641977,
-3.95275577056508));
#22204=CARTESIAN_POINT('Ctrl Pts',(-0.0266713951301605,1.54830693619751,
-3.87173755056599));
#22205=CARTESIAN_POINT('Ctrl Pts',(0.0129013415238527,2.806754275421,-3.08378606043707));
#22206=CARTESIAN_POINT('Ctrl Pts',(0.0524740781778653,3.44845954321452,
-1.94752767122311));
#22207=CARTESIAN_POINT('Ctrl Pts',(0.0920468148318783,4.09016481100804,
-0.811269282009136));
#22208=CARTESIAN_POINT('Ctrl Pts',(0.131619551485891,4.1151280073716,0.673296006289876));
#22209=CARTESIAN_POINT('Ctrl Pts',(0.171192288139904,3.51198744236147,1.83048667191605));
#22210=CARTESIAN_POINT('Ctrl Pts',(0.210765024793917,2.90884687735135,2.98767733754223));
#22211=CARTESIAN_POINT('Ctrl Pts',(0.250337761447931,1.67760255096752,3.81749338049556));
#22212=CARTESIAN_POINT('Ctrl Pts',(0.289910498101944,0.378640083609367,
3.94225429652265));
#22213=CARTESIAN_POINT('Ctrl Pts',(0.329483234755957,-0.920322383748772,
4.06701521254974));
#22214=CARTESIAN_POINT('Ctrl Pts',(0.369055971409969,-2.28700299208125,
3.48672100165062));
#22215=CARTESIAN_POINT('Ctrl Pts',(0.408628708063982,-3.09937397307536,
2.46548539366795));
#22216=CARTESIAN_POINT('Ctrl Pts',(0.435365857165736,-3.6482489279384,1.77549195304792));
#22217=CARTESIAN_POINT('Ctrl Pts',(0.462103006267491,-3.94408314364839,
0.884210041980504));
#22218=CARTESIAN_POINT('Ctrl Pts',(0.488840155369245,-3.95065042271477,
-0.00310251149715996));
#22219=CARTESIAN_POINT('Origin',(4.7,0.,0.));
#22220=CARTESIAN_POINT('',(1.34415984463077,-3.96026049768271,-0.00065371468560671));
#22221=CARTESIAN_POINT('',(1.23884015536925,-3.9603872214563,-0.000165414599889812));
#22222=CARTESIAN_POINT('',(4.7,-3.954,-4.84225344382863E-16));
#22223=CARTESIAN_POINT('Ctrl Pts',(1.34415984463077,-3.96026049768271,-0.00065371468560671));
#22224=CARTESIAN_POINT('Ctrl Pts',(1.30566911122168,-3.95733483282496,1.26872354929189));
#22225=CARTESIAN_POINT('Ctrl Pts',(1.26717837781259,-3.29247871293452,2.54073655968515));
#22226=CARTESIAN_POINT('Ctrl Pts',(1.2286876444035,-2.24736922314309,3.26099191795255));
#22227=CARTESIAN_POINT('Ctrl Pts',(1.18911490774948,-1.17288092554265,4.00149419192653));
#22228=CARTESIAN_POINT('Ctrl Pts',(1.14954217109547,0.303539635603274,4.15878216827251));
#22229=CARTESIAN_POINT('Ctrl Pts',(1.10996943444146,1.50991791032203,3.66126817075332));
#22230=CARTESIAN_POINT('Ctrl Pts',(1.07039669778744,2.71629618504079,3.16375417323414));
#22231=CARTESIAN_POINT('Ctrl Pts',(1.03082396113343,3.65263217333238,2.01143820184979));
#22232=CARTESIAN_POINT('Ctrl Pts',(0.991251224479416,3.89276413584316,0.7287826128386));
#22233=CARTESIAN_POINT('Ctrl Pts',(0.951678487825403,4.13289609835394,-0.553872976172574));
#22234=CARTESIAN_POINT('Ctrl Pts',(0.912105751171391,3.67682403508393,-1.96686818281059));
#22235=CARTESIAN_POINT('Ctrl Pts',(0.872533014517378,2.73212350244037,-2.86709572241591));
#22236=CARTESIAN_POINT('Ctrl Pts',(0.832960277863366,1.7874229697968,-3.76732326202123));
#22237=CARTESIAN_POINT('Ctrl Pts',(0.793387541209353,0.354093967779691,
-4.15478313459385));
#22238=CARTESIAN_POINT('Ctrl Pts',(0.75381480455534,-0.915501543584075,
-3.85312777335216));
#22239=CARTESIAN_POINT('Ctrl Pts',(0.714242067901327,-2.18509705494786,
-3.55147241211047));
#22240=CARTESIAN_POINT('Ctrl Pts',(0.674669331247314,-3.29095907565829,
-2.56070181705443));
#22241=CARTESIAN_POINT('Ctrl Pts',(0.635096594593301,-3.72976819033012,
-1.33175296526204));
#22242=CARTESIAN_POINT('Ctrl Pts',(0.621451011272456,-3.8810795941522,-0.907983335660524));
#22243=CARTESIAN_POINT('Ctrl Pts',(0.607805427951612,-3.95307654709183,
-0.455893647073924));
#22244=CARTESIAN_POINT('Ctrl Pts',(0.594159844630767,-3.95001826622686,
-0.00286169934786473));
#22245=CARTESIAN_POINT('Ctrl Pts',(0.488840155369245,-3.95065042271477,
-0.00310251149715996));
#22246=CARTESIAN_POINT('Ctrl Pts',(0.501675742921504,-3.95380314797787,
-0.429070812120259));
#22247=CARTESIAN_POINT('Ctrl Pts',(0.514511330473762,-3.89029053186911,
-0.854124322474488));
#22248=CARTESIAN_POINT('Ctrl Pts',(0.527346918026021,-3.75610460203848,
-1.2555538498656));
#22249=CARTESIAN_POINT('Ctrl Pts',(0.566919654680034,-3.34240289635171,
-2.49318048035031));
#22250=CARTESIAN_POINT('Ctrl Pts',(0.606492391334046,-2.25693813132239,
-3.5062567362535));
#22251=CARTESIAN_POINT('Ctrl Pts',(0.646065127988059,-0.993746163797144,
-3.83369349496089));
#22252=CARTESIAN_POINT('Ctrl Pts',(0.685637864642072,0.26944580372809,-4.16113025366827));
#22253=CARTESIAN_POINT('Ctrl Pts',(0.725210601296086,1.71036497374923,-3.80292751517983));
#22254=CARTESIAN_POINT('Ctrl Pts',(0.764783337950099,2.67319481518899,-2.9221168237108));
#22255=CARTESIAN_POINT('Ctrl Pts',(0.804356074604112,3.63602465662875,-2.04130613224176));
#22256=CARTESIAN_POINT('Ctrl Pts',(0.843928811258124,4.12076516948713,-0.637887487792129));
#22257=CARTESIAN_POINT('Ctrl Pts',(0.883501547912137,3.9067927072547,0.649390478763368));
#22258=CARTESIAN_POINT('Ctrl Pts',(0.92307428456615,3.69282024502226,1.93666844531887));
#22259=CARTESIAN_POINT('Ctrl Pts',(0.962647021220164,2.78013480769901,3.10780573398024));
#22260=CARTESIAN_POINT('Ctrl Pts',(1.00221975787418,1.58413387900453,3.62977369883537));
#22261=CARTESIAN_POINT('Ctrl Pts',(1.04179249452819,0.388132950310035,4.15174166369052));
#22262=CARTESIAN_POINT('Ctrl Pts',(1.0813652311822,-1.09118346975568,4.02454030473942));
#22263=CARTESIAN_POINT('Ctrl Pts',(1.12093796783622,-2.18052281686445,3.30606374658756));
#22264=CARTESIAN_POINT('Ctrl Pts',(1.16023869701389,-3.26237447240231,2.59252571460078));
#22265=CARTESIAN_POINT('Ctrl Pts',(1.19953942619157,-3.95959172893657,1.29581293552976));
#22266=CARTESIAN_POINT('Ctrl Pts',(1.23884015536925,-3.9603872214563,-0.000165414599889812));
#22267=CARTESIAN_POINT('Origin',(4.7,0.,0.));
#22268=CARTESIAN_POINT('',(2.09415984463077,-3.95182140471939,0.00339740089000562));
#22269=CARTESIAN_POINT('',(1.98884015536925,-3.95110529642541,0.00323787354723457));
#22270=CARTESIAN_POINT('',(4.7,-3.954,-4.84225344382863E-16));
#22271=CARTESIAN_POINT('Ctrl Pts',(2.09415984463077,-3.95182140471939,0.00339740089000562));
#22272=CARTESIAN_POINT('Ctrl Pts',(2.08267826779977,-3.95497662709706,0.384145209727677));
#22273=CARTESIAN_POINT('Ctrl Pts',(2.07119669096877,-3.90439221631175,0.764072168098434));
#22274=CARTESIAN_POINT('Ctrl Pts',(2.05971511413777,-3.79664813820596,1.12703133440906));
#22275=CARTESIAN_POINT('Ctrl Pts',(2.02014237748376,-3.42529426480786,2.37801695389204));
#22276=CARTESIAN_POINT('Ctrl Pts',(1.98056964082974,-2.37492629601307,3.42743789470054));
#22277=CARTESIAN_POINT('Ctrl Pts',(1.94099690417573,-1.12360621613093,3.79766320059515));
#22278=CARTESIAN_POINT('Ctrl Pts',(1.90142416752171,0.127713863751167,4.16788850648974));
#22279=CARTESIAN_POINT('Ctrl Pts',(1.8618514308677,1.57998605472057,3.85891817747047));
#22280=CARTESIAN_POINT('Ctrl Pts',(1.82227869421369,2.57222663869159,3.011376235758));
#22281=CARTESIAN_POINT('Ctrl Pts',(1.78270595755968,3.56446722266259,2.16383429404553));
#22282=CARTESIAN_POINT('Ctrl Pts',(1.74313322090566,4.0966761996352,0.777720739639841));
#22283=CARTESIAN_POINT('Ctrl Pts',(1.70356048425165,3.9266252390076,-0.516091994193958));
#22284=CARTESIAN_POINT('Ctrl Pts',(1.66398774759764,3.75657427838,-1.80990472802779));
#22285=CARTESIAN_POINT('Ctrl Pts',(1.62441501094363,2.88426338015217,-3.01141664128973));
#22286=CARTESIAN_POINT('Ctrl Pts',(1.58484227428961,1.70671405614722,-3.57377445352));
#22287=CARTESIAN_POINT('Ctrl Pts',(1.5452695376356,0.52916473214227,-4.13613226575025));
#22288=CARTESIAN_POINT('Ctrl Pts',(1.50569680098158,-0.953623017639813,
-4.05933597694883));
#22289=CARTESIAN_POINT('Ctrl Pts',(1.46612406432757,-2.06677669610277,-3.37833846772776));
#22290=CARTESIAN_POINT('Ctrl Pts',(1.42655132767356,-3.17993037456572,-2.6973409585067));
#22291=CARTESIAN_POINT('Ctrl Pts',(1.38697859101955,-3.92344998170957,-1.41214222886602));
#22292=CARTESIAN_POINT('Ctrl Pts',(1.34740585436553,-3.95893176825402,-0.107684578244696));
#22293=CARTESIAN_POINT('Ctrl Pts',(1.34632385112061,-3.9599019161746,-0.0720179165433403));
#22294=CARTESIAN_POINT('Ctrl Pts',(1.34524184787569,-3.96034274030552,-0.036336857016415));
#22295=CARTESIAN_POINT('Ctrl Pts',(1.34415984463077,-3.96026049768271,-0.00065371468560671));
#22296=CARTESIAN_POINT('Ctrl Pts',(1.23884015536925,-3.9603872214563,-0.000165414599889812));
#22297=CARTESIAN_POINT('Ctrl Pts',(1.23911216284558,-3.96039272720434,-0.00913511586959148));
#22298=CARTESIAN_POINT('Ctrl Pts',(1.23938417032192,-3.96036487243322,-0.0181047819581257));
#22299=CARTESIAN_POINT('Ctrl Pts',(1.23965617779825,-3.96030355377182,-0.0270742192741198));
#22300=CARTESIAN_POINT('Ctrl Pts',(1.27922891445227,-3.95138266941864,-1.33198386963134));
#22301=CARTESIAN_POINT('Ctrl Pts',(1.31880165110628,-3.23417862656048,-2.63205141299318));
#22302=CARTESIAN_POINT('Ctrl Pts',(1.35837438776029,-2.13511797100763,-3.33556719333418));
#22303=CARTESIAN_POINT('Ctrl Pts',(1.3979471244143,-1.03605731545477,-4.03908297367518));
#22304=CARTESIAN_POINT('Ctrl Pts',(1.43751986106832,0.444859952792789,-4.14604699099532));
#22305=CARTESIAN_POINT('Ctrl Pts',(1.47709259772233,1.63361266316492,-3.60777589632646));
#22306=CARTESIAN_POINT('Ctrl Pts',(1.51666533437635,2.82236537353706,-3.06950480165761));
#22307=CARTESIAN_POINT('Ctrl Pts',(1.55623807103036,3.71895352603377,-1.88599859499978));
#22308=CARTESIAN_POINT('Ctrl Pts',(1.59581080768437,3.91530611694513,-0.595915482244824));
#22309=CARTESIAN_POINT('Ctrl Pts',(1.63538354433838,4.11165870785648,0.694167630510099));
#22310=CARTESIAN_POINT('Ctrl Pts',(1.6749562809924,3.60777573718251,2.09082764936215));
#22311=CARTESIAN_POINT('Ctrl Pts',(1.71452901764641,2.63299330424895,2.95839204824972));
#22312=CARTESIAN_POINT('Ctrl Pts',(1.75410175430042,1.65821087131538,3.82595644713731));
#22313=CARTESIAN_POINT('Ctrl Pts',(1.79367449095443,0.212528976122227,4.16442522606043));
#22314=CARTESIAN_POINT('Ctrl Pts',(1.83324722760845,-1.0460681548226,3.81974850832264));
#22315=CARTESIAN_POINT('Ctrl Pts',(1.87281996426246,-2.30466528576745,3.47507179058484));
#22316=CARTESIAN_POINT('Ctrl Pts',(1.91239270091647,-3.37617765246396,2.44724957618611));
#22317=CARTESIAN_POINT('Ctrl Pts',(1.95196543757049,-3.77291965952719,1.20408242829145));
#22318=CARTESIAN_POINT('Ctrl Pts',(1.96425701017007,-3.89615054006395,0.81794589734172));
#22319=CARTESIAN_POINT('Ctrl Pts',(1.97654858276966,-3.95428175936265,0.41103358390573));
#22320=CARTESIAN_POINT('Ctrl Pts',(1.98884015536925,-3.95110529642541,0.00323787354723457));
#22321=CARTESIAN_POINT('Origin',(4.7,0.,0.));
#22322=CARTESIAN_POINT('',(2.84415984463077,-3.94879606319858,-0.00214324138103211));
#22323=CARTESIAN_POINT('',(2.73884015536925,-3.94927650700756,-0.0024772734444678));
#22324=CARTESIAN_POINT('',(4.7,-3.954,-4.84225344382863E-16));
#22325=CARTESIAN_POINT('Ctrl Pts',(2.84415984463077,-3.94879606319858,-0.00214324138103211));
#22326=CARTESIAN_POINT('Ctrl Pts',(2.82011468772384,-3.94483830299845,0.796774452968311));
#22327=CARTESIAN_POINT('Ctrl Pts',(2.79606953081692,-3.70949558657619,1.5978361366702));
#22328=CARTESIAN_POINT('Ctrl Pts',(2.77202437391,-3.25896341504729,2.25030979499844));
#22329=CARTESIAN_POINT('Ctrl Pts',(2.73245163725599,-2.51749223034729,3.3241297062035));
#22330=CARTESIAN_POINT('Ctrl Pts',(2.69287890060197,-1.19316953698868,3.99549144530754));
#22331=CARTESIAN_POINT('Ctrl Pts',(2.65330616394796,0.111255577602164,3.95883302382597));
#22332=CARTESIAN_POINT('Ctrl Pts',(2.61373342729395,1.41568069219301,3.9221746023444));
#22333=CARTESIAN_POINT('Ctrl Pts',(2.57416069063994,2.70020822801613,3.17749602027721));
#22334=CARTESIAN_POINT('Ctrl Pts',(2.53458795398592,3.38020137119358,2.06372852000055));
#22335=CARTESIAN_POINT('Ctrl Pts',(2.49501521733191,4.06019451437106,0.949961019723846));
#22336=CARTESIAN_POINT('Ctrl Pts',(2.4554424806779,4.13565326490285,-0.532895398762326));
#22337=CARTESIAN_POINT('Ctrl Pts',(2.41586974402388,3.57223350617034,-1.70993698465078));
#22338=CARTESIAN_POINT('Ctrl Pts',(2.37629700736987,3.00881374743785,-2.88697857053918));
#22339=CARTESIAN_POINT('Ctrl Pts',(2.33672427071586,1.80651547944111,-3.75820532382986));
#22340=CARTESIAN_POINT('Ctrl Pts',(2.29715153406185,0.512549882267534,-3.92708916785323));
#22341=CARTESIAN_POINT('Ctrl Pts',(2.25757879740783,-0.78141571490604,-4.09597301187659));
#22342=CARTESIAN_POINT('Ctrl Pts',(2.21800606075382,-2.16704864125646,-3.56251394663264));
#22343=CARTESIAN_POINT('Ctrl Pts',(2.17843332409981,-3.01369521543096,-2.56950926493196));
#22344=CARTESIAN_POINT('Ctrl Pts',(2.15034216427679,-3.6146969716825,-1.86461353172711));
#22345=CARTESIAN_POINT('Ctrl Pts',(2.12225100445378,-3.94410174587872,-0.928151262481906));
#22346=CARTESIAN_POINT('Ctrl Pts',(2.09415984463077,-3.95182140471939,0.00339740089000562));
#22347=CARTESIAN_POINT('Ctrl Pts',(1.98884015536925,-3.95110529642541,0.00323787354723457));
#22348=CARTESIAN_POINT('Ctrl Pts',(2.01612131942367,-3.94405513211149,-0.901865324993545));
#22349=CARTESIAN_POINT('Ctrl Pts',(2.0434024834781,-3.63499186103326,-1.81132030196311));
#22350=CARTESIAN_POINT('Ctrl Pts',(2.07068364753253,-3.06537576631618,-2.50763008887844));
#22351=CARTESIAN_POINT('Ctrl Pts',(2.11025638418654,-2.23911821861202,-3.51766337676301));
#22352=CARTESIAN_POINT('Ctrl Pts',(2.14982912084055,-0.86463147577378,-4.07921787114163));
#22353=CARTESIAN_POINT('Ctrl Pts',(2.18940185749456,0.432503828354505,-3.93670899227079));
#22354=CARTESIAN_POINT('Ctrl Pts',(2.22897459414858,1.72963913248281,-3.79420011339995));
#22355=CARTESIAN_POINT('Ctrl Pts',(2.26854733080259,2.94942299790115,-2.94762786127962));
#22356=CARTESIAN_POINT('Ctrl Pts',(2.3081200674566,3.53668589121304,-1.78229912143322));
#22357=CARTESIAN_POINT('Ctrl Pts',(2.34769280411062,4.12394878452495,-0.616970381586784));
#22358=CARTESIAN_POINT('Ctrl Pts',(2.38726554076463,4.07869070573037,0.867114845985733));
#22359=CARTESIAN_POINT('Ctrl Pts',(2.42683827741864,3.42151030939356,1.99449353322607));
#22360=CARTESIAN_POINT('Ctrl Pts',(2.46641101407266,2.76432991305676,3.12187222046637));
#22361=CARTESIAN_POINT('Ctrl Pts',(2.50598375072667,1.49522719917778,3.89254436737451));
#22362=CARTESIAN_POINT('Ctrl Pts',(2.54555648738068,0.191818564785084,3.95574808216736));
#22363=CARTESIAN_POINT('Ctrl Pts',(2.5851292240347,-1.11159006960763,4.01895179696022));
#22364=CARTESIAN_POINT('Ctrl Pts',(2.62470196068871,-2.44930462451406,3.37468707963778));
#22365=CARTESIAN_POINT('Ctrl Pts',(2.66427469734272,-3.21248087242804,2.31618304450469));
#22366=CARTESIAN_POINT('Ctrl Pts',(2.68912985001823,-3.69182255470969,1.65134958527496));
#22367=CARTESIAN_POINT('Ctrl Pts',(2.71398500269374,-3.94451216648441,0.823101088397621));
#22368=CARTESIAN_POINT('Ctrl Pts',(2.73884015536925,-3.94927650700756,-0.0024772734444678));
#22369=CARTESIAN_POINT('Origin',(4.7,0.,0.));
#22370=CARTESIAN_POINT('',(3.59415984463077,-3.95946408857375,-0.00171547380415804));
#22371=CARTESIAN_POINT('',(3.48884015536925,-3.95988464442629,-0.0012757644514219));
#22372=CARTESIAN_POINT('',(4.7,-3.954,-4.84225344382863E-16));
#22373=CARTESIAN_POINT('Ctrl Pts',(3.59415984463077,-3.95946408857375,-0.00171547380415804));
#22374=CARTESIAN_POINT('Ctrl Pts',(3.55755110764792,-3.95286445098715,1.20624346856487));
#22375=CARTESIAN_POINT('Ctrl Pts',(3.52094237066508,-3.35954953332255,2.41981313494161));
#22376=CARTESIAN_POINT('Ctrl Pts',(3.48433363368223,-2.39904223913318,3.15108442427959));
#22377=CARTESIAN_POINT('Ctrl Pts',(3.44476089702822,-1.36076817288979,3.94156255984524));
#22378=CARTESIAN_POINT('Ctrl Pts',(3.4051881603742,0.106564219678576,4.16848287757163));
#22379=CARTESIAN_POINT('Ctrl Pts',(3.36561542372019,1.33511675607524,3.72856540263541));
#22380=CARTESIAN_POINT('Ctrl Pts',(3.32604268706618,2.56366929247188,3.2886479276992));
#22381=CARTESIAN_POINT('Ctrl Pts',(3.28646995041217,3.55344197269683,2.1818926601004));
#22382=CARTESIAN_POINT('Ctrl Pts',(3.24689721375816,3.85395200825982,0.912025565492931));
#22383=CARTESIAN_POINT('Ctrl Pts',(3.20732447710414,4.15446204382282,-0.357841529114534));
#22384=CARTESIAN_POINT('Ctrl Pts',(3.16775174045013,3.76570943472387,-1.79082045073066));
#22385=CARTESIAN_POINT('Ctrl Pts',(3.12817900379612,2.86463012077892,-2.73470857409136));
#22386=CARTESIAN_POINT('Ctrl Pts',(3.0886062671421,1.96355080683398,-3.67859669745204));
#22387=CARTESIAN_POINT('Ctrl Pts',(3.04903353048809,0.550144788043063,-4.13339402255731));
#22388=CARTESIAN_POINT('Ctrl Pts',(3.00946079383408,-0.732293674866088,
-3.89210517430269));
#22389=CARTESIAN_POINT('Ctrl Pts',(2.96988805718007,-2.01473213777531,-3.65081632604805));
#22390=CARTESIAN_POINT('Ctrl Pts',(2.93031532052605,-3.16620304480276,-2.71344130443343));
#22391=CARTESIAN_POINT('Ctrl Pts',(2.89074258387204,-3.66262866029575,-1.50661475197305));
#22392=CARTESIAN_POINT('Ctrl Pts',(2.87521500412495,-3.85741651134733,-1.03307925459082));
#22393=CARTESIAN_POINT('Ctrl Pts',(2.85968742437786,-3.95135185592497,-0.518058286493471));
#22394=CARTESIAN_POINT('Ctrl Pts',(2.84415984463077,-3.94879606319858,-0.00214324138103211));
#22395=CARTESIAN_POINT('Ctrl Pts',(2.73884015536925,-3.94927650700756,-0.0024772734444678));
#22396=CARTESIAN_POINT('Ctrl Pts',(2.75355773934775,-3.95209763559475,-0.49133039093987));
#22397=CARTESIAN_POINT('Ctrl Pts',(2.76827532332625,-3.86799050714696,-0.979247298167196));
#22398=CARTESIAN_POINT('Ctrl Pts',(2.78299290730476,-3.69253847048653,-1.43174610016721));
#22399=CARTESIAN_POINT('Ctrl Pts',(2.82256564395877,-3.2207818797095,-2.6484278567624));
#22400=CARTESIAN_POINT('Ctrl Pts',(2.86213838061279,-2.08863075723384,-3.60904801700904));
#22401=CARTESIAN_POINT('Ctrl Pts',(2.9017111172668,-0.811369677826096,-3.87639220116739));
#22402=CARTESIAN_POINT('Ctrl Pts',(2.94128385392081,0.465891401581615,-4.14373638532573));
#22403=CARTESIAN_POINT('Ctrl Pts',(2.98085659057482,1.88826243792143,-3.71780459339582));
#22404=CARTESIAN_POINT('Ctrl Pts',(3.02042932722884,2.80836885365649,-2.79245441022394));
#22405=CARTESIAN_POINT('Ctrl Pts',(3.06000206388285,3.72847526939156,-1.86710422705205));
#22406=CARTESIAN_POINT('Ctrl Pts',(3.09957480053686,4.14631706452186,-0.442335652638224));
#22407=CARTESIAN_POINT('Ctrl Pts',(3.13914753719087,3.87171871614322,0.833385525692216));
#22408=CARTESIAN_POINT('Ctrl Pts',(3.17872027384489,3.59712036776459,2.10910670402262));
#22409=CARTESIAN_POINT('Ctrl Pts',(3.2182930104989,2.63008187587697,3.23578048626965));
#22410=CARTESIAN_POINT('Ctrl Pts',(3.25786574715291,1.41073884444955,3.70061524129814));
#22411=CARTESIAN_POINT('Ctrl Pts',(3.29743848380693,0.191395813022067,4.16544999632666));
#22412=CARTESIAN_POINT('Ctrl Pts',(3.33701122046094,-1.28025175794523,3.96844572413664));
#22413=CARTESIAN_POINT('Ctrl Pts',(3.37658395711496,-2.33440168590114,3.19926648159057));
#22414=CARTESIAN_POINT('Ctrl Pts',(3.41400268986639,-3.33117263907,2.47195482845881));
#22415=CARTESIAN_POINT('Ctrl Pts',(3.45142142261782,-3.95465904777607,1.23306166885008));
#22416=CARTESIAN_POINT('Ctrl Pts',(3.48884015536925,-3.95988464442629,-0.0012757644514219));
#22417=CARTESIAN_POINT('Origin',(4.7,0.,0.));
#22418=CARTESIAN_POINT('',(4.34415984463077,-3.95361637884632,0.00355905447742291));
#22419=CARTESIAN_POINT('',(4.23884015536925,-3.95282662999892,0.00352652566842014));
#22420=CARTESIAN_POINT('',(4.7,-3.954,-4.84225344382863E-16));
#22421=CARTESIAN_POINT('Ctrl Pts',(4.34415984463077,-3.95361637884632,0.00355905447742291));
#22422=CARTESIAN_POINT('Ctrl Pts',(4.33456026422602,-3.9564854253942,0.321529051071549));
#22423=CARTESIAN_POINT('Ctrl Pts',(4.32496068382126,-3.92132433711414,0.638872526236415));
#22424=CARTESIAN_POINT('Ctrl Pts',(4.3153611034165,-3.84569027880081,0.946257361197047));
#22425=CARTESIAN_POINT('Ctrl Pts',(4.27578836676249,-3.53390095619407,2.21340223758226));
#22426=CARTESIAN_POINT('Ctrl Pts',(4.23621563010848,-2.53432656349926,3.31131307838228));
#22427=CARTESIAN_POINT('Ctrl Pts',(4.19664289345447,-1.3019110173562,3.74028934936446));
#22428=CARTESIAN_POINT('Ctrl Pts',(4.15707015680045,-0.0694954712131363,
4.16926562034663));
#22429=CARTESIAN_POINT('Ctrl Pts',(4.11749742014644,1.39576122837819,3.92930732151097));
#22430=CARTESIAN_POINT('Ctrl Pts',(4.07792468349243,2.42696562489611,3.12962850345776));
#22431=CARTESIAN_POINT('Ctrl Pts',(4.03835194683841,3.45817002141404,2.32994968540454));
#22432=CARTESIAN_POINT('Ctrl Pts',(3.99877921018441,4.05532211485856,0.970550348133779));
#22433=CARTESIAN_POINT('Ctrl Pts',(3.95920647353039,3.94663551873683,-0.329855720471081));
#22434=CARTESIAN_POINT('Ctrl Pts',(3.91963373687638,3.8379489226151,-1.63026178907598));
#22435=CARTESIAN_POINT('Ctrl Pts',(3.88006100022236,3.02342363692707,-2.87167458901497));
#22436=CARTESIAN_POINT('Ctrl Pts',(3.84048826356835,1.87378076695643,-3.48908044496925));
#22437=CARTESIAN_POINT('Ctrl Pts',(3.80091552691433,0.724137896985802,-4.10648630092352));
#22438=CARTESIAN_POINT('Ctrl Pts',(3.76134279026032,-0.760622557267377,
-4.09988521289311));
#22439=CARTESIAN_POINT('Ctrl Pts',(3.72177005360631,-1.90473024667613,-3.47228158441675));
#22440=CARTESIAN_POINT('Ctrl Pts',(3.6821973169523,-3.04883793608485,-2.84467795594042));
#22441=CARTESIAN_POINT('Ctrl Pts',(3.64262458029828,-3.85229286064914,-1.5960717870181));
#22442=CARTESIAN_POINT('Ctrl Pts',(3.60305184364427,-3.94941245297207,-0.294750725854538));
#22443=CARTESIAN_POINT('Ctrl Pts',(3.6000878439731,-3.95668671459885,-0.197281722608817));
#22444=CARTESIAN_POINT('Ctrl Pts',(3.59712384430194,-3.95999842341425,-0.0995169879520828));
#22445=CARTESIAN_POINT('Ctrl Pts',(3.59415984463077,-3.95946408857375,-0.00171547380415804));
#22446=CARTESIAN_POINT('Ctrl Pts',(3.48884015536925,-3.95988464442629,-0.0012757644514219));
#22447=CARTESIAN_POINT('Ctrl Pts',(3.49099415927183,-3.9601854551366,-0.0723302190770247));
#22448=CARTESIAN_POINT('Ctrl Pts',(3.49314816317441,-3.95843752728934,-0.143369577335591));
#22449=CARTESIAN_POINT('Ctrl Pts',(3.49530216707699,-3.95459413083459,-0.214295384307806));
#22450=CARTESIAN_POINT('Ctrl Pts',(3.534874903731,-3.8839843628677,-1.51732379475814));
#22451=CARTESIAN_POINT('Ctrl Pts',(3.57444764038502,-3.10611254198946,-2.78202640275678));
#22452=CARTESIAN_POINT('Ctrl Pts',(3.61402037703903,-1.97501740250559,-3.43278946502215));
#22453=CARTESIAN_POINT('Ctrl Pts',(3.65359311369304,-0.843922263021716,
-4.08355252728753));
#22454=CARTESIAN_POINT('Ctrl Pts',(3.69316585034705,0.640396195067791,-4.12037604381963));
#22455=CARTESIAN_POINT('Ctrl Pts',(3.73273858700107,1.80236879172075,-3.52650024670325));
#22456=CARTESIAN_POINT('Ctrl Pts',(3.77231132365508,2.96434138837375,-2.93262444958684));
#22457=CARTESIAN_POINT('Ctrl Pts',(3.8118840603091,3.80396812359018,-1.70804933882191));
#22458=CARTESIAN_POINT('Ctrl Pts',(3.85145679696311,3.93910327792533,-0.410125123840174));
#22459=CARTESIAN_POINT('Ctrl Pts',(3.89102953361713,4.07423843226048,0.887799091141527));
#22460=CARTESIAN_POINT('Ctrl Pts',(3.93060227027114,3.50488200571439,2.25907241034003));
#22461=CARTESIAN_POINT('Ctrl Pts',(3.97017500692515,2.49016953091971,3.07957674991972));
#22462=CARTESIAN_POINT('Ctrl Pts',(4.00974774357916,1.47545705612503,3.90008108949941));
#22463=CARTESIAN_POINT('Ctrl Pts',(4.04932048023317,0.0153885330817553,
4.16981644946029));
#22464=CARTESIAN_POINT('Ctrl Pts',(4.08889321688719,-1.22550391604859,3.76601611827626));
#22465=CARTESIAN_POINT('Ctrl Pts',(4.1284659535412,-2.46639636517894,3.36221578709222));
#22466=CARTESIAN_POINT('Ctrl Pts',(4.16803869019521,-3.48811274039636,2.28487976476326));
#22467=CARTESIAN_POINT('Ctrl Pts',(4.20761142684922,-3.82563147568885,1.02434421147664));
#22468=CARTESIAN_POINT('Ctrl Pts',(4.21802100302256,-3.91441550434159,0.69276135998306));
#22469=CARTESIAN_POINT('Ctrl Pts',(4.22843057919591,-3.95585656325474,0.348502039960021));
#22470=CARTESIAN_POINT('Ctrl Pts',(4.23884015536925,-3.95282662999892,0.00352652566842014));
#22471=CARTESIAN_POINT('Origin',(4.7,0.,0.));
#22472=CARTESIAN_POINT('',(5.09415984463078,-3.94797828517504,-0.00125412662908497));
#22473=CARTESIAN_POINT('',(4.98884015536925,-3.94827688052699,-0.00165327621010028));
#22474=CARTESIAN_POINT('',(4.7,-3.954,-4.84225344382863E-16));
#22475=CARTESIAN_POINT('Ctrl Pts',(5.09415984463078,-3.94797828517504,-0.00125412662908497));
#22476=CARTESIAN_POINT('Ctrl Pts',(5.0719966841501,-3.94586967481992,0.735514823501616));
#22477=CARTESIAN_POINT('Ctrl Pts',(5.04983352366942,-3.74808709220802,1.47333516746832));
#22478=CARTESIAN_POINT('Ctrl Pts',(5.02767036318874,-3.36171787287947,2.09370238029319));
#22479=CARTESIAN_POINT('Ctrl Pts',(4.98809762653473,-2.67184842122634,3.20137961627701));
#22480=CARTESIAN_POINT('Ctrl Pts',(4.94852488988071,-1.38075027064227,3.93460723880349));
#22481=CARTESIAN_POINT('Ctrl Pts',(4.9089521532267,-0.0760507690123915,
3.95966576804347));
#22482=CARTESIAN_POINT('Ctrl Pts',(4.86937941657269,1.22864873261751,3.98472429728344));
#22483=CARTESIAN_POINT('Ctrl Pts',(4.82980667991868,2.54694958529321,3.30161373323687));
#22484=CARTESIAN_POINT('Ctrl Pts',(4.79023394326466,3.27884346786418,2.22124339668733));
#22485=CARTESIAN_POINT('Ctrl Pts',(4.75066120661065,4.01073735043511,1.14087306013782));
#22486=CARTESIAN_POINT('Ctrl Pts',(4.71108846995663,4.15622426290134,-0.336757048914672));
#22487=CARTESIAN_POINT('Ctrl Pts',(4.67151573330262,3.64908763723056,-1.53912186973409));
#22488=CARTESIAN_POINT('Ctrl Pts',(4.63194299664861,3.14195101155977,-2.74148669055352));
#22489=CARTESIAN_POINT('Ctrl Pts',(4.5923702599946,1.98219084775198,-3.66858622313989));
#22490=CARTESIAN_POINT('Ctrl Pts',(4.55279752334059,0.697657634116575,-3.89846258666689));
#22491=CARTESIAN_POINT('Ctrl Pts',(4.51322478668657,-0.586875579518827,
-4.12833895019389));
#22492=CARTESIAN_POINT('Ctrl Pts',(4.47365205003256,-1.99618184298182,-3.6609921446615));
#22493=CARTESIAN_POINT('Ctrl Pts',(4.43407931337854,-2.888832848454,-2.7091292859101));
#22494=CARTESIAN_POINT('Ctrl Pts',(4.40410615712929,-3.56494398772144,-1.9881699435562));
#22495=CARTESIAN_POINT('Ctrl Pts',(4.37413300088003,-3.94465823934023,-0.989251463133344));
#22496=CARTESIAN_POINT('Ctrl Pts',(4.34415984463077,-3.95361637884632,0.00355905447742291));
#22497=CARTESIAN_POINT('Ctrl Pts',(4.23884015536925,-3.95282662999892,0.00352652566842014));
#22498=CARTESIAN_POINT('Ctrl Pts',(4.26800331584992,-3.94433805867635,-0.962946663792761));
#22499=CARTESIAN_POINT('Ctrl Pts',(4.29716647633059,-3.58680571057285,-1.93504111646879));
#22500=CARTESIAN_POINT('Ctrl Pts',(4.32632963681127,-2.94338137561686,-2.64976288166296));
#22501=CARTESIAN_POINT('Ctrl Pts',(4.36590237346528,-2.07029144488486,-3.61959933727155));
#22502=CARTESIAN_POINT('Ctrl Pts',(4.40547511011929,-0.67079048805332,-4.11553716424445));
#22503=CARTESIAN_POINT('Ctrl Pts',(4.4450478467733,0.618155951047059,-3.91185639710254));
#22504=CARTESIAN_POINT('Ctrl Pts',(4.48462058342732,1.90710239014744,-3.70817562996064));
#22505=CARTESIAN_POINT('Ctrl Pts',(4.52419332008133,3.08549431151664,-2.80487626870394));
#22506=CARTESIAN_POINT('Ctrl Pts',(4.56376605673534,3.61700121293053,-1.61308384066856));
#22507=CARTESIAN_POINT('Ctrl Pts',(4.60333879338935,4.14850811434442,-0.421291412633197));
#22508=CARTESIAN_POINT('Ctrl Pts',(4.64291153004337,4.033129995803,1.05899408218087));
#22509=CARTESIAN_POINT('Ctrl Pts',(4.68248426669738,3.32337978033369,2.15403901706449));
#22510=CARTESIAN_POINT('Ctrl Pts',(4.7220570033514,2.61362956486436,3.24908395194817));
#22511=CARTESIAN_POINT('Ctrl Pts',(4.76162974000541,1.3095072524671,3.95888832690141));
#22512=CARTESIAN_POINT('Ctrl Pts',(4.80120247665942,0.00456797712235453,
3.96039346340133));
#22513=CARTESIAN_POINT('Ctrl Pts',(4.84077521331344,-1.30037129822235,3.96189859990126));
#22514=CARTESIAN_POINT('Ctrl Pts',(4.88034794996745,-2.60612753651453,3.25510449794791));
#22515=CARTESIAN_POINT('Ctrl Pts',(4.91992068662146,-3.31840194262003,2.16169974755576));
#22516=CARTESIAN_POINT('Ctrl Pts',(4.94289384287072,-3.73189852151165,1.52694561381809));
#22517=CARTESIAN_POINT('Ctrl Pts',(4.96586699911999,-3.9453828521266,0.761897912850191));
#22518=CARTESIAN_POINT('Ctrl Pts',(4.98884015536925,-3.94827688052699,-0.00165327621010028));
#22519=CARTESIAN_POINT('Origin',(4.7,0.,0.));
#22520=CARTESIAN_POINT('',(5.84415984463077,-3.95812868148667,-0.00259109635525723));
#22521=CARTESIAN_POINT('',(5.73884015536925,-3.95875693366943,-0.00224257783873754));
#22522=CARTESIAN_POINT('',(4.7,-3.954,-4.84225344382863E-16));
#22523=CARTESIAN_POINT('Ctrl Pts',(5.84415984463077,-3.95812868148667,-0.00259109635525723));
#22524=CARTESIAN_POINT('Ctrl Pts',(5.80943310407417,-3.94941271527673,1.14428747213603));
#22525=CARTESIAN_POINT('Ctrl Pts',(5.77470636351757,-3.4226605516743,2.29814636133711));
#22526=CARTESIAN_POINT('Ctrl Pts',(5.73997962296097,-2.54534896397193,3.03412843592516));
#22527=CARTESIAN_POINT('Ctrl Pts',(5.70040688630696,-1.54561158962567,3.87281425420047));
#22528=CARTESIAN_POINT('Ctrl Pts',(5.66083414965294,-0.0906495641330535,
4.16885932720762));
#22529=CARTESIAN_POINT('Ctrl Pts',(5.62126141299893,1.15732914951951,3.78752240306972));
#22530=CARTESIAN_POINT('Ctrl Pts',(5.58168867634492,2.40530786317208,3.40618547893183));
#22531=CARTESIAN_POINT('Ctrl Pts',(5.54211593969091,3.44630326498462,2.34746655764887));
#22532=CARTESIAN_POINT('Ctrl Pts',(5.5025432030369,3.80651917853864,1.09322845622502));
#22533=CARTESIAN_POINT('Ctrl Pts',(5.46297046638288,4.16673509209267,-0.161009645198846));
#22534=CARTESIAN_POINT('Ctrl Pts',(5.42339772972887,3.84617151738819,-1.61076692676359));
#22535=CARTESIAN_POINT('Ctrl Pts',(5.38382499307485,2.99072899897088,-2.59620430028094));
#22536=CARTESIAN_POINT('Ctrl Pts',(5.34425225642084,2.13528648055357,-3.58164167379831));
#22537=CARTESIAN_POINT('Ctrl Pts',(5.30467951976683,0.744965018423408,-4.10275913926823));
#22538=CARTESIAN_POINT('Ctrl Pts',(5.26510678311281,-0.547447777020062,
-3.92237653030894));
#22539=CARTESIAN_POINT('Ctrl Pts',(5.2255340464588,-1.8398605724635,-3.74199392134966));
#22540=CARTESIAN_POINT('Ctrl Pts',(5.18596130980479,-3.03436470122026,-2.8601112379612));
#22541=CARTESIAN_POINT('Ctrl Pts',(5.14638857315078,-3.58729638923753,-1.67810647154643));
#22542=CARTESIAN_POINT('Ctrl Pts',(5.12897899697745,-3.83055240727213,-1.15809689530562));
#22543=CARTESIAN_POINT('Ctrl Pts',(5.11156942080411,-3.94963463796052,-0.579999886766972));
#22544=CARTESIAN_POINT('Ctrl Pts',(5.09415984463078,-3.94797828517504,-0.00125412662908497));
#22545=CARTESIAN_POINT('Ctrl Pts',(4.98884015536925,-3.94827688052699,-0.00165327621010028));
#22546=CARTESIAN_POINT('Ctrl Pts',(5.005439735774,-3.95036800186029,-0.553368034879958));
#22547=CARTESIAN_POINT('Ctrl Pts',(5.02203931617875,-3.84251013030004,-1.10430146613177));
#22548=CARTESIAN_POINT('Ctrl Pts',(5.0386388965835,-3.62071269423261,-1.60473575307272));
#22549=CARTESIAN_POINT('Ctrl Pts',(5.07821163323751,-3.0919564658209,-2.79775110447809));
#22550=CARTESIAN_POINT('Ctrl Pts',(5.11778436989152,-1.9156514350787,-3.70376640845788));
#22551=CARTESIAN_POINT('Ctrl Pts',(5.15735710654554,-0.627178281783331,
-3.91042000995114));
#22552=CARTESIAN_POINT('Ctrl Pts',(5.19692984319955,0.661294871512074,-4.11707361144442));
#22553=CARTESIAN_POINT('Ctrl Pts',(5.23650257985356,2.06193614736065,-3.62436551045113));
#22554=CARTESIAN_POINT('Ctrl Pts',(5.27607531650758,2.93726099984076,-2.65654570263367));
#22555=CARTESIAN_POINT('Ctrl Pts',(5.31564805316159,3.81258585232085,-1.68872589481625));
#22556=CARTESIAN_POINT('Ctrl Pts',(5.3552207898156,4.16259428143251,-0.24579438017468));
#22557=CARTESIAN_POINT('Ctrl Pts',(5.39479352646961,3.82798428148137,1.01551641645942));
#22558=CARTESIAN_POINT('Ctrl Pts',(5.43436626312363,3.49337428153023,2.27682721309352));
#22559=CARTESIAN_POINT('Ctrl Pts',(5.47393899977764,2.4741458525163,3.35651729172016));
#22560=CARTESIAN_POINT('Ctrl Pts',(5.51351173643165,1.23418820252157,3.76317907255602));
#22561=CARTESIAN_POINT('Ctrl Pts',(5.55308447308566,-0.00576944747316441,
4.16984085339188));
#22562=CARTESIAN_POINT('Ctrl Pts',(5.59265720973968,-1.4664563184487,3.90347433643695));
#22563=CARTESIAN_POINT('Ctrl Pts',(5.63222994639369,-2.48305885483325,3.08531294600745));
#22564=CARTESIAN_POINT('Ctrl Pts',(5.66776668271888,-3.39597869150952,2.35059535855969));
#22565=CARTESIAN_POINT('Ctrl Pts',(5.70330341904407,-3.95077870340937,1.17089768960724));
#22566=CARTESIAN_POINT('Ctrl Pts',(5.73884015536925,-3.95875693366943,-0.00224257783873754));
#22567=CARTESIAN_POINT('Origin',(4.7,0.,0.));
#22568=CARTESIAN_POINT('',(6.59415984463077,-3.95548544114442,0.00341059480280986));
#22569=CARTESIAN_POINT('',(6.48884015536925,-3.95468133138785,0.0035131856141757));
#22570=CARTESIAN_POINT('',(4.7,-3.954,-4.84225344382863E-16));
#22571=CARTESIAN_POINT('Ctrl Pts',(6.59415984463077,-3.95548544114442,0.00341059480280986));
#22572=CARTESIAN_POINT('Ctrl Pts',(6.58644226065226,-3.95780309731958,0.258732729269525));
#22573=CARTESIAN_POINT('Ctrl Pts',(6.57872467667375,-3.93518375266648,0.51364602629909));
#22574=CARTESIAN_POINT('Ctrl Pts',(6.57100709269525,-3.88613019748507,0.763366754762944));
#22575=CARTESIAN_POINT('Ctrl Pts',(6.53143435604123,-3.63460285077364,2.04383647845702));
#22576=CARTESIAN_POINT('Ctrl Pts',(6.49186161938722,-2.68805792945867,3.18778136035047));
#22577=CARTESIAN_POINT('Ctrl Pts',(6.4522888827332,-1.47730364243954,3.6745490420074));
#22578=CARTESIAN_POINT('Ctrl Pts',(6.41271614607919,-0.266549355420404,
4.16131672366433));
#22579=CARTESIAN_POINT('Ctrl Pts',(6.37314340942518,1.20841429730289,3.99090720508476));
#22580=CARTESIAN_POINT('Ctrl Pts',(6.33357067277117,2.27627585959928,3.24088027009456));
#22581=CARTESIAN_POINT('Ctrl Pts',(6.29399793611716,3.3441374218957,2.49085333510434));
#22582=CARTESIAN_POINT('Ctrl Pts',(6.25442519946314,4.00489689376518,1.16120898370345));
#22583=CARTESIAN_POINT('Ctrl Pts',(6.21485246280913,3.95781777746819,-0.142881609871119));
#22584=CARTESIAN_POINT('Ctrl Pts',(6.17527972615511,3.91073866117121,-1.44697220344565));
#22585=CARTESIAN_POINT('Ctrl Pts',(6.1357069895011,3.15582095670779,-2.72550903919386));
#22586=CARTESIAN_POINT('Ctrl Pts',(6.09613425284709,2.03665611631933,-3.39658189625124));
#22587=CARTESIAN_POINT('Ctrl Pts',(6.05656151619308,0.917491275930869,-4.06765475330863));
#22588=CARTESIAN_POINT('Ctrl Pts',(6.01698877953907,-0.565920700382629,
-4.13126363167517));
#22589=CARTESIAN_POINT('Ctrl Pts',(5.97741604288505,-1.73842320654302,-3.55845773742436));
#22590=CARTESIAN_POINT('Ctrl Pts',(5.93784330623104,-2.91092571270342,-2.98565184317355));
#22591=CARTESIAN_POINT('Ctrl Pts',(5.89827056957702,-3.77251874871071,-1.77643117630538));
#22592=CARTESIAN_POINT('Ctrl Pts',(5.85869783292301,-3.93105890511442,-0.481157561099551));
#22593=CARTESIAN_POINT('Ctrl Pts',(5.8538518368256,-3.9504734072231,-0.32254101306424));
#22594=CARTESIAN_POINT('Ctrl Pts',(5.84900584072818,-3.95934496431545,-0.162634019417884));
#22595=CARTESIAN_POINT('Ctrl Pts',(5.84415984463077,-3.95812868148667,-0.00259109635525723));
#22596=CARTESIAN_POINT('Ctrl Pts',(5.73884015536925,-3.95875693366943,-0.00224257783873754));
#22597=CARTESIAN_POINT('Ctrl Pts',(5.74287615569808,-3.95966304220056,-0.135479194219172));
#22598=CARTESIAN_POINT('Ctrl Pts',(5.74691215602691,-3.95351583846345,-0.268631228379135));
#22599=CARTESIAN_POINT('Ctrl Pts',(5.75094815635573,-3.94003888469953,-0.401037203290042));
#22600=CARTESIAN_POINT('Ctrl Pts',(5.79052089300975,-3.80789817638765,-1.69926969825382));
#22601=CARTESIAN_POINT('Ctrl Pts',(5.83009362966376,-2.97109855797036,-2.92577842427728));
#22602=CARTESIAN_POINT('Ctrl Pts',(5.86966636631777,-1.81049902166246,-3.52233311086931));
#22603=CARTESIAN_POINT('Ctrl Pts',(5.90923910297178,-0.649899485354549,
-4.11888779746134));
#22604=CARTESIAN_POINT('Ctrl Pts',(5.9488118396258,0.834499968843993,-4.08548844462194));
#22605=CARTESIAN_POINT('Ctrl Pts',(5.98838457627981,1.96709329651415,-3.43733635453036));
#22606=CARTESIAN_POINT('Ctrl Pts',(6.02795731293382,3.09968662418432,-2.78918426443878));
#22607=CARTESIAN_POINT('Ctrl Pts',(6.06753004958783,3.88047382532609,-1.52627943709504));
#22608=CARTESIAN_POINT('Ctrl Pts',(6.10710278624184,3.95408926638018,-0.223417378160364));
#22609=CARTESIAN_POINT('Ctrl Pts',(6.14667552289586,4.02770470743426,1.07944468077433));
#22610=CARTESIAN_POINT('Ctrl Pts',(6.18624825954988,3.3941483884006,2.42226397129993));
#22611=CARTESIAN_POINT('Ctrl Pts',(6.22582099620389,2.34177562860268,3.19387290865644));
#22612=CARTESIAN_POINT('Ctrl Pts',(6.2653937328579,1.28940286880478,3.96548184601292));
#22613=CARTESIAN_POINT('Ctrl Pts',(6.30496646951191,-0.181786331757368,
4.16588043020035));
#22614=CARTESIAN_POINT('Ctrl Pts',(6.34453920616592,-1.40219841215079,3.70385972524997));
#22615=CARTESIAN_POINT('Ctrl Pts',(6.38411194281993,-2.62261049254421,3.2418390202996));
#22616=CARTESIAN_POINT('Ctrl Pts',(6.42368467947395,-3.59224545276892,2.11739902621141));
#22617=CARTESIAN_POINT('Ctrl Pts',(6.46325741612797,-3.86978593841946,0.842314693079716));
#22618=CARTESIAN_POINT('Ctrl Pts',(6.47178499587506,-3.92959349343203,0.567545135691775));
#22619=CARTESIAN_POINT('Ctrl Pts',(6.48031257562216,-3.95726260853577,0.285780183576929));
#22620=CARTESIAN_POINT('Ctrl Pts',(6.48884015536925,-3.95468133138785,0.0035131856141757));
#22621=CARTESIAN_POINT('Origin',(4.7,0.,0.));
#22622=CARTESIAN_POINT('',(7.34415984463077,-3.94761516686083,-0.000266384231551453));
#22623=CARTESIAN_POINT('',(7.23884015536925,-3.94771372514716,-0.000698679637915435));
#22624=CARTESIAN_POINT('',(4.7,-3.954,-4.84225344382863E-16));
#22625=CARTESIAN_POINT('Ctrl Pts',(7.34415984463077,-3.94761516686083,-0.000266384231551453));
#22626=CARTESIAN_POINT('Ctrl Pts',(7.32387868057634,-3.94720746447042,0.674094403609092));
#22627=CARTESIAN_POINT('Ctrl Pts',(7.30359751652191,-3.78327622808021,1.34864110485744));
#22628=CARTESIAN_POINT('Ctrl Pts',(7.28331635246748,-3.45695268116967,1.93241167307498));
#22629=CARTESIAN_POINT('Ctrl Pts',(7.24374361581347,-2.82022809518258,3.07146852900473));
#22630=CARTESIAN_POINT('Ctrl Pts',(7.20417087915945,-1.56524247678311,3.8649219167271));
#22631=CARTESIAN_POINT('Ctrl Pts',(7.16459814250544,-0.26318700166963,3.95164134458515));
#22632=CARTESIAN_POINT('Ctrl Pts',(7.12502540585142,1.0388684734438,4.0383607724432));
#22633=CARTESIAN_POINT('Ctrl Pts',(7.08545266919741,2.38799380527123,3.41834624043699));
#22634=CARTESIAN_POINT('Ctrl Pts',(7.0458799325434,3.17015129238174,2.37378969108322));
#22635=CARTESIAN_POINT('Ctrl Pts',(7.00630719588939,3.95230877949225,1.32923314172946));
#22636=CARTESIAN_POINT('Ctrl Pts',(6.96673445923537,4.16749842188584,-0.139865424971873));
#22637=CARTESIAN_POINT('Ctrl Pts',(6.92716172258136,3.71777931646781,-1.36486397422117));
#22638=CARTESIAN_POINT('Ctrl Pts',(6.88758898592735,3.26806021104977,-2.58986252347049));
#22639=CARTESIAN_POINT('Ctrl Pts',(6.84801624927334,2.15343235782014,-3.57076105526773));
#22640=CARTESIAN_POINT('Ctrl Pts',(6.80844351261932,0.881204832371534,-3.86111573997565));
#22641=CARTESIAN_POINT('Ctrl Pts',(6.76887077596531,-0.391022693077072,
-4.15147042468356));
#22642=CARTESIAN_POINT('Ctrl Pts',(6.72929803931129,-1.82084989074469,-3.75128126230207));
#22643=CARTESIAN_POINT('Ctrl Pts',(6.68972530265728,-2.75750860352453,-2.84268939836396));
#22644=CARTESIAN_POINT('Ctrl Pts',(6.65787014998178,-3.51149755711427,-2.11129361953467));
#22645=CARTESIAN_POINT('Ctrl Pts',(6.62601499730628,-3.94591906758573,-1.05045880234535));
#22646=CARTESIAN_POINT('Ctrl Pts',(6.59415984463077,-3.95548544114442,0.00341059480280986));
#22647=CARTESIAN_POINT('Ctrl Pts',(6.48884015536925,-3.95468133138785,0.0035131856141757));
#22648=CARTESIAN_POINT('Ctrl Pts',(6.51988531227617,-3.94528403972316,-1.02409646463657));
#22649=CARTESIAN_POINT('Ctrl Pts',(6.55093046918308,-3.5349580443317,-2.05836006467214));
#22650=CARTESIAN_POINT('Ctrl Pts',(6.58197562609,-2.81480309023937,-2.78596855950419));
#22651=CARTESIAN_POINT('Ctrl Pts',(6.62154836274401,-1.89683374533234,-3.71343880678121));
#22652=CARTESIAN_POINT('Ctrl Pts',(6.66112109939803,-0.475449044441877,
-4.14265062915996));
#22653=CARTESIAN_POINT('Ctrl Pts',(6.70069383605204,0.802425353270519,-3.87825357652071));
#22654=CARTESIAN_POINT('Ctrl Pts',(6.74026657270606,2.08029975098288,-3.61385652388146));
#22655=CARTESIAN_POINT('Ctrl Pts',(6.77983930936007,3.21466384551719,-2.65585059622425));
#22656=CARTESIAN_POINT('Ctrl Pts',(6.81941204601408,3.68922585525657,-1.4402603376728));
#22657=CARTESIAN_POINT('Ctrl Pts',(6.85898478266809,4.16378786499596,-0.224670079121361));
#22658=CARTESIAN_POINT('Ctrl Pts',(6.89855751932211,3.97854778994043,1.24850451032431));
#22659=CARTESIAN_POINT('Ctrl Pts',(6.93813025597612,3.21781535819058,2.30876624454704));
#22660=CARTESIAN_POINT('Ctrl Pts',(6.97770299263014,2.45708292644072,3.36902797876977));
#22661=CARTESIAN_POINT('Ctrl Pts',(7.01727572928414,1.12085813799653,4.01637685776957));
#22662=CARTESIAN_POINT('Ctrl Pts',(7.05684846593816,-0.182692828407551,
3.95618004921609));
#22663=CARTESIAN_POINT('Ctrl Pts',(7.09642120259217,-1.48624379481167,3.89598324066261));
#22664=CARTESIAN_POINT('Ctrl Pts',(7.13599393924619,-2.7571209391757,3.12824074455581));
#22665=CARTESIAN_POINT('Ctrl Pts',(7.1755666759002,-3.41690025439169,2.00238105836652));
#22666=CARTESIAN_POINT('Ctrl Pts',(7.19665783572322,-3.76854414262731,1.40232939180324));
#22667=CARTESIAN_POINT('Ctrl Pts',(7.21774899554623,-3.94660011203609,0.700551267122433));
#22668=CARTESIAN_POINT('Ctrl Pts',(7.23884015536925,-3.94771372514716,-0.000698679637915435));
#22669=CARTESIAN_POINT('Origin',(4.7,0.,0.));
#22670=CARTESIAN_POINT('',(8.09415984463078,-3.95644716314161,-0.00320656848566359));
#22671=CARTESIAN_POINT('',(7.98884015536925,-3.95720150084823,-0.00297693462621818));
#22672=CARTESIAN_POINT('',(4.7,-3.954,-4.84225344382863E-16));
#22673=CARTESIAN_POINT('Ctrl Pts',(8.09415984463078,-3.95644716314161,-0.00320656848566359));
#22674=CARTESIAN_POINT('Ctrl Pts',(8.06131510050042,-3.94689655284687,1.08271904018544));
#22675=CARTESIAN_POINT('Ctrl Pts',(8.02847035637007,-3.48188740146714,2.17583507877882));
#22676=CARTESIAN_POINT('Ctrl Pts',(7.99562561223971,-2.68596213185717,2.91038556557579));
#22677=CARTESIAN_POINT('Ctrl Pts',(7.9560528755857,-1.72699770925295,3.79540305445398));
#22678=CARTESIAN_POINT('Ctrl Pts',(7.91648013893168,-0.287660578712081,
4.15991067512015));
#22679=CARTESIAN_POINT('Ctrl Pts',(7.87690740227767,0.976952774382327,3.8380072942491));
#22680=CARTESIAN_POINT('Ctrl Pts',(7.83733466562366,2.24156612747672,3.51610391337806));
#22681=CARTESIAN_POINT('Ctrl Pts',(7.79776192896965,3.33145570312463,2.50778953096983));
#22682=CARTESIAN_POINT('Ctrl Pts',(7.75818919231564,3.75057174667662,1.27198596183832));
#22683=CARTESIAN_POINT('Ctrl Pts',(7.71861645566162,4.16968779022862,0.0361823927067614));
#22684=CARTESIAN_POINT('Ctrl Pts',(7.6790437190076,3.91803030168461,-1.42711036314813));
#22685=CARTESIAN_POINT('Ctrl Pts',(7.63947098235359,3.11013807308118,-2.45189271389543));
#22686=CARTESIAN_POINT('Ctrl Pts',(7.59989824569957,2.30224584447777,-3.4766750646427));
#22687=CARTESIAN_POINT('Ctrl Pts',(7.56032550904557,0.938118875814986,-4.06294701028245));
#22688=CARTESIAN_POINT('Ctrl Pts',(7.52075277239156,-0.361377322092827,
-3.9438741289701));
#22689=CARTESIAN_POINT('Ctrl Pts',(7.48118003573754,-1.66087352000064,-3.82480124765774));
#22690=CARTESIAN_POINT('Ctrl Pts',(7.44160729908353,-2.89573894715346,-3.00038353939327));
#22691=CARTESIAN_POINT('Ctrl Pts',(7.40203456242951,-3.50393988394249,-1.8458445231925));
#22692=CARTESIAN_POINT('Ctrl Pts',(7.38274298982993,-3.80043574243673,-1.28301073575904));
#22693=CARTESIAN_POINT('Ctrl Pts',(7.36345141723035,-3.94800297597488,-0.641722666623542));
#22694=CARTESIAN_POINT('Ctrl Pts',(7.34415984463077,-3.94761516686083,-0.000266384231551453));
#22695=CARTESIAN_POINT('Ctrl Pts',(7.23884015536925,-3.94771372514716,-0.000698679637915435));
#22696=CARTESIAN_POINT('Ctrl Pts',(7.25732173220024,-3.94868955229203,-0.615183842025179));
#22697=CARTESIAN_POINT('Ctrl Pts',(7.27580330903124,-3.81379996271696,-1.22926344231433));
#22698=CARTESIAN_POINT('Ctrl Pts',(7.29428488586223,-3.5407879365703,-1.77413585714432));
#22699=CARTESIAN_POINT('Ctrl Pts',(7.33385762251625,-2.95621481746495,-2.94081621019416));
#22700=CARTESIAN_POINT('Ctrl Pts',(7.37343035917026,-1.73838709318626,-3.79020004002209));
#22701=CARTESIAN_POINT('Ctrl Pts',(7.41300309582428,-0.441583983695238,
-3.93570080630005));
#22702=CARTESIAN_POINT('Ctrl Pts',(7.45257583247829,0.855219125795781,-4.081201572578));
#22703=CARTESIAN_POINT('Ctrl Pts',(7.4921485691323,2.23099762049913,-3.52281927530597));
#22704=CARTESIAN_POINT('Ctrl Pts',(7.53172130578631,3.05958294169278,-2.51469470796547));
#22705=CARTESIAN_POINT('Ctrl Pts',(7.57129404244033,3.88816826288645,-1.50657014062495));
#22706=CARTESIAN_POINT('Ctrl Pts',(7.61086677909435,4.1695604105704,-0.0487033032159304));
#22707=CARTESIAN_POINT('Ctrl Pts',(7.65043951574836,3.77568723052116,1.19537575207398));
#22708=CARTESIAN_POINT('Ctrl Pts',(7.69001225240237,3.38181405047194,2.43945480736386));
#22709=CARTESIAN_POINT('Ctrl Pts',(7.72958498905637,2.31267554268956,3.46974608053465));
#22710=CARTESIAN_POINT('Ctrl Pts',(7.76915772571039,1.05487687004705,3.81732524687205));
#22711=CARTESIAN_POINT('Ctrl Pts',(7.8087304623644,-0.202921802595454,4.16490441320944));
#22712=CARTESIAN_POINT('Ctrl Pts',(7.84830319901842,-1.64938064009809,3.82977147271344));
#22713=CARTESIAN_POINT('Ctrl Pts',(7.88787593567243,-2.62616180027425,2.96445803649627));
#22714=CARTESIAN_POINT('Ctrl Pts',(7.92153067557138,-3.45686795464837,2.22854990657432));
#22715=CARTESIAN_POINT('Ctrl Pts',(7.95518541547031,-3.94787044850959,1.10917825725707));
#22716=CARTESIAN_POINT('Ctrl Pts',(7.98884015536925,-3.95720150084823,-0.00297693462621818));
#22717=CARTESIAN_POINT('Origin',(4.7,0.,0.));
#22718=CARTESIAN_POINT('',(8.84415984463078,-3.95727591145965,0.00295051159254288));
#22719=CARTESIAN_POINT('',(8.73884015536925,-3.95652560052937,0.00318574057616234));
#22720=CARTESIAN_POINT('',(4.7,-3.954,-4.84225344382863E-16));
#22721=CARTESIAN_POINT('Ctrl Pts',(8.84415984463078,-3.95727591145965,0.00295051159254288));
#22722=CARTESIAN_POINT('Ctrl Pts',(8.83832425707851,-3.95888409829544,0.195783997048772));
#22723=CARTESIAN_POINT('Ctrl Pts',(8.83248866952625,-3.94599938707022,0.3884017661895));
#22724=CARTESIAN_POINT('Ctrl Pts',(8.82665308197398,-3.91787743633585,0.578768613465758));
#22725=CARTESIAN_POINT('Ctrl Pts',(8.78708034531997,-3.72717469378571,1.86969896922656));
#22726=CARTESIAN_POINT('Ctrl Pts',(8.74750760866596,-2.83577652030062,3.05711906219486));
#22727=CARTESIAN_POINT('Ctrl Pts',(8.70793487201194,-1.64939176486137,3.60058932955289));
#22728=CARTESIAN_POINT('Ctrl Pts',(8.66836213535793,-0.463007009422064,
4.14405959691094));
#22729=CARTESIAN_POINT('Ctrl Pts',(8.62878939870392,1.0183643279714,4.04358003865869));
#22730=CARTESIAN_POINT('Ctrl Pts',(8.58921666204991,2.12049441279558,3.3448826824547));
#22731=CARTESIAN_POINT('Ctrl Pts',(8.54964392539589,3.22262449761972,2.64618532625074));
#22732=CARTESIAN_POINT('Ctrl Pts',(8.51007118874188,3.94551332987458,1.34927017209508));
#22733=CARTESIAN_POINT('Ctrl Pts',(8.47049845208787,3.96014700219647,0.0444121050719863));
#22734=CARTESIAN_POINT('Ctrl Pts',(8.43092571543385,3.97478067451836,-1.26044596195111));
#22735=CARTESIAN_POINT('Ctrl Pts',(8.39135297877984,3.28115918690728,-2.57324694184166));
#22736=CARTESIAN_POINT('Ctrl Pts',(8.35178024212583,2.19497577695067,-3.29648571249481));
#22737=CARTESIAN_POINT('Ctrl Pts',(8.31220750547182,1.10879236699404,-4.01972448314798));
#22738=CARTESIAN_POINT('Ctrl Pts',(8.2726347688178,-0.3699529653081,-4.15340104456376));
#22739=CARTESIAN_POINT('Ctrl Pts',(8.23306203216379,-1.56822757915689,-3.63667416385554));
#22740=CARTESIAN_POINT('Ctrl Pts',(8.19348929550978,-2.76650219300569,-3.11994728314731));
#22741=CARTESIAN_POINT('Ctrl Pts',(8.15391655885576,-3.68430608840111,-1.95281696031504));
#22742=CARTESIAN_POINT('Ctrl Pts',(8.11434382220175,-3.90391217876503,-0.666488120353801));
#22743=CARTESIAN_POINT('Ctrl Pts',(8.10761582967809,-3.94124869524191,-0.447791827148448));
#22744=CARTESIAN_POINT('Ctrl Pts',(8.10088783715443,-3.95840353200246,-0.225650054341145));
#22745=CARTESIAN_POINT('Ctrl Pts',(8.09415984463078,-3.95644716314161,-0.00320656848566359));
#22746=CARTESIAN_POINT('Ctrl Pts',(7.98884015536925,-3.95720150084823,-0.00297693462621818));
#22747=CARTESIAN_POINT('Ctrl Pts',(7.99475815212432,-3.95884231392916,-0.198543170956203));
#22748=CARTESIAN_POINT('Ctrl Pts',(8.00067614887939,-3.94558924647289,-0.393886265439571));
#22749=CARTESIAN_POINT('Ctrl Pts',(8.00659414563446,-3.91667037322966,-0.586881963287379));
#22750=CARTESIAN_POINT('Ctrl Pts',(8.04616688228848,-3.72329430315924,-1.87741459491562));
#22751=CARTESIAN_POINT('Ctrl Pts',(8.0857396189425,-2.82943868016865,-3.0629859262337));
#22752=CARTESIAN_POINT('Ctrl Pts',(8.12531235559651,-1.64193083097396,-3.60399783541336));
#22753=CARTESIAN_POINT('Ctrl Pts',(8.16488509225053,-0.454422981779327,
-4.14500974459299));
#22754=CARTESIAN_POINT('Ctrl Pts',(8.20445782890453,1.02673709361936,-4.04146223163425));
#22755=CARTESIAN_POINT('Ctrl Pts',(8.24403056555854,2.12741771398153,-3.34048366581915));
#22756=CARTESIAN_POINT('Ctrl Pts',(8.28360330221256,3.22809833434371,-2.63950510000405));
#22757=CARTESIAN_POINT('Ctrl Pts',(8.32317603886657,3.94829949966936,-1.3410954813326));
#22758=CARTESIAN_POINT('Ctrl Pts',(8.36274877552059,3.9602305609419,-0.0362098819216899));
#22759=CARTESIAN_POINT('Ctrl Pts',(8.4023215121746,3.97216162221444,1.2686757174892));
#22760=CARTESIAN_POINT('Ctrl Pts',(8.44189424882861,3.27582257943385,2.58003729763958));
#22761=CARTESIAN_POINT('Ctrl Pts',(8.48146698548262,2.18814353179743,3.30102486140593));
#22762=CARTESIAN_POINT('Ctrl Pts',(8.52103972213664,1.10046448416096,4.02201242517232));
#22763=CARTESIAN_POINT('Ctrl Pts',(8.56061245879065,-0.37855456833137,4.15262597255467));
#22764=CARTESIAN_POINT('Ctrl Pts',(8.60018519544467,-1.57575640452294,3.63341836360361));
#22765=CARTESIAN_POINT('Ctrl Pts',(8.63975793209868,-2.77295824071448,3.11421075465256));
#22766=CARTESIAN_POINT('Ctrl Pts',(8.67933066875269,-3.68834286060526,1.94518198936815));
#22767=CARTESIAN_POINT('Ctrl Pts',(8.7189034054067,-3.90528428092833,0.658401045337166));
#22768=CARTESIAN_POINT('Ctrl Pts',(8.72554898872755,-3.9417159863498,0.442307575380675));
#22769=CARTESIAN_POINT('Ctrl Pts',(8.7321945720484,-3.95845046258346,0.22289330331233));
#22770=CARTESIAN_POINT('Ctrl Pts',(8.73884015536925,-3.95652560052937,0.00318574057616234));
#22771=CARTESIAN_POINT('Origin',(4.7,0.,0.));
#22772=CARTESIAN_POINT('',(9.59415984463078,-3.94772861144879,0.000742196070642187));
#22773=CARTESIAN_POINT('',(9.48884015536925,-3.9476212151691,0.00031064949736361));
#22774=CARTESIAN_POINT('',(4.7,-3.954,-4.84225344382863E-16));
#22775=CARTESIAN_POINT('Ctrl Pts',(9.59415984463078,-3.94772861144879,0.000742196070642187));
#22776=CARTESIAN_POINT('Ctrl Pts',(9.57576067700259,-3.9487608168787,0.612481575277166));
#22777=CARTESIAN_POINT('Ctrl Pts',(9.5573615093744,-3.81512540423781,1.22379386335884));
#22778=CARTESIAN_POINT('Ctrl Pts',(9.53896234174621,-3.54445481419423,1.7667984560266));
#22779=CARTESIAN_POINT('Ctrl Pts',(9.4993896050922,-2.96229934954316,2.93468703565128));
#22780=CARTESIAN_POINT('Ctrl Pts',(9.45981686843819,-1.74623347451844,3.78659135450272));
#22781=CARTESIAN_POINT('Ctrl Pts',(9.42024413178417,-0.449734525193319,
3.93477770286096));
#22782=CARTESIAN_POINT('Ctrl Pts',(9.38067139513016,0.846764424131798,4.08296405121919));
#22783=CARTESIAN_POINT('Ctrl Pts',(9.34109865847615,2.22369644775731,3.52743242908423));
#22784=CARTESIAN_POINT('Ctrl Pts',(9.30152592182214,3.05436797254543,2.52102618042165));
#22785=CARTESIAN_POINT('Ctrl Pts',(9.26195318516812,3.88503949733354,1.51461993175908));
#22786=CARTESIAN_POINT('Ctrl Pts',(9.22238044851411,4.16945052328425,0.0573390565689048));
#22787=CARTESIAN_POINT('Ctrl Pts',(9.1828077118601,3.77815489108496,-1.18755308641483));
#22788=CARTESIAN_POINT('Ctrl Pts',(9.14323497520609,3.38685925888568,-2.43244522939857));
#22789=CARTESIAN_POINT('Ctrl Pts',(9.10366223855208,2.3198569685364,-3.46494864017587));
#22790=CARTESIAN_POINT('Ctrl Pts',(9.06408950189806,1.06278090997786,-3.81513216697263));
#22791=CARTESIAN_POINT('Ctrl Pts',(9.02451676524405,-0.194295148580706,
-4.1653156937694));
#22792=CARTESIAN_POINT('Ctrl Pts',(8.98494402859004,-1.64144497534855,-3.83317933658557));
#22793=CARTESIAN_POINT('Ctrl Pts',(8.94537129193602,-2.62001623292487,-2.96989084871697));
#22794=CARTESIAN_POINT('Ctrl Pts',(8.91163414283427,-3.45428262981783,-2.23390706554609));
#22795=CARTESIAN_POINT('Ctrl Pts',(8.87789699373252,-3.94797853761737,-1.11187331589373));
#22796=CARTESIAN_POINT('Ctrl Pts',(8.84415984463078,-3.95727591145965,0.00295051159254288));
#22797=CARTESIAN_POINT('Ctrl Pts',(8.73884015536925,-3.95652560052937,0.00318574057616234));
#22798=CARTESIAN_POINT('Ctrl Pts',(8.77176730870242,-3.9469884049304,-1.0854086321664));
#22799=CARTESIAN_POINT('Ctrl Pts',(8.80469446203558,-3.47937430514818,-2.18120313596773));
#22800=CARTESIAN_POINT('Ctrl Pts',(8.83762161536874,-2.67992852017388,-2.91594245109975));
#22801=CARTESIAN_POINT('Ctrl Pts',(8.87719435202275,-1.71913311834099,-3.79897188072816));
#22802=CARTESIAN_POINT('Ctrl Pts',(8.91676708867676,-0.279044093919909,
-4.16049761720741));
#22803=CARTESIAN_POINT('Ctrl Pts',(8.95633982533078,0.984899852510242,-3.83597569490375));
#22804=CARTESIAN_POINT('Ctrl Pts',(8.99591256198479,2.24884379894041,-3.51145377260009));
#22805=CARTESIAN_POINT('Ctrl Pts',(9.03548529863881,3.33664266737961,-2.50088419151347));
#22806=CARTESIAN_POINT('Ctrl Pts',(9.07505803529282,3.75319826269509,-1.26421519223174));
#22807=CARTESIAN_POINT('Ctrl Pts',(9.11463077194684,4.16975385801057,-0.0275461929500335));
#22808=CARTESIAN_POINT('Ctrl Pts',(9.15420350860084,3.91506618020236,1.43522222452681));
#22809=CARTESIAN_POINT('Ctrl Pts',(9.19377624525486,3.10505317445673,2.45832911449284));
#22810=CARTESIAN_POINT('Ctrl Pts',(9.23334898190887,2.29504016871111,3.48143600445886));
#22811=CARTESIAN_POINT('Ctrl Pts',(9.27292171856288,0.92970183502812,4.06488136691408));
#22812=CARTESIAN_POINT('Ctrl Pts',(9.3124944552169,-0.369544977977794,3.94311726437579));
#22813=CARTESIAN_POINT('Ctrl Pts',(9.35206719187091,-1.66879179098376,3.82135316183748));
#22814=CARTESIAN_POINT('Ctrl Pts',(9.39163992852492,-2.90194708331263,2.99437959430555));
#22815=CARTESIAN_POINT('Ctrl Pts',(9.43121266517893,-3.50775548206036,1.83858334851659));
#22816=CARTESIAN_POINT('Ctrl Pts',(9.45042182857571,-3.80182340615735,1.27754358184973));
#22817=CARTESIAN_POINT('Ctrl Pts',(9.46963099197248,-3.94807157344821,0.639024371465793));
#22818=CARTESIAN_POINT('Ctrl Pts',(9.48884015536925,-3.9476212151691,0.00031064949736361));
#22819=CARTESIAN_POINT('Origin',(4.7,0.,0.));
#22820=CARTESIAN_POINT('',(10.3441598446308,-3.95459914581543,-0.00352034347287922));
#22821=CARTESIAN_POINT('',(10.2388401553693,-3.95540412882742,-0.0034237005329492));
#22822=CARTESIAN_POINT('',(4.7,-3.954,-4.84225344382863E-16));
#22823=CARTESIAN_POINT('Ctrl Pts',(10.3441598446308,-3.95459914581543,-0.00352034347287922));
#22824=CARTESIAN_POINT('Ctrl Pts',(10.3131970969267,-3.94522735882427,1.02141614396006));
#22825=CARTESIAN_POINT('Ctrl Pts',(10.2822343492226,-3.53730596752864,2.05296951176746));
#22826=CARTESIAN_POINT('Ctrl Pts',(10.2512716015185,-2.82056721260417,2.78013260713677));
#22827=CARTESIAN_POINT('Ctrl Pts',(10.2116988648644,-1.90452079871997,3.70950211763882));
#22828=CARTESIAN_POINT('Ctrl Pts',(10.1721261282104,-0.484028140502754,
4.14165693807744));
#22829=CARTESIAN_POINT('Ctrl Pts',(10.1325533915564,0.794391105071104,3.87990714918108));
#22830=CARTESIAN_POINT('Ctrl Pts',(10.0929806549024,2.07281035064496,3.61815736028473));
#22831=CARTESIAN_POINT('Ctrl Pts',(10.0534079182484,3.20915618357542,2.66250296205341));
#22832=CARTESIAN_POINT('Ctrl Pts',(10.0138351815944,3.68623485853561,1.44789822908918));
#22833=CARTESIAN_POINT('Ctrl Pts',(9.97426244494036,4.1633135334958,0.233293496124942));
#22834=CARTESIAN_POINT('Ctrl Pts',(9.93468970828635,3.98112505048568,-1.24026157157228));
#22835=CARTESIAN_POINT('Ctrl Pts',(9.89511697163234,3.22259024324513,-2.30209661791679));
#22836=CARTESIAN_POINT('Ctrl Pts',(9.85554423497832,2.46405543600457,-3.36393166426134));
#22837=CARTESIAN_POINT('Ctrl Pts',(9.8159714983243,1.12917430453357,-4.01404668925322));
#22838=CARTESIAN_POINT('Ctrl Pts',(9.77639876167029,-0.174498521279079,
-3.95654988344063));
#22839=CARTESIAN_POINT('Ctrl Pts',(9.73682602501627,-1.47817134709166,-3.89905307762803));
#22840=CARTESIAN_POINT('Ctrl Pts',(9.69725328836227,-2.75063586724586,-3.13394444101105));
#22841=CARTESIAN_POINT('Ctrl Pts',(9.65768055170826,-3.41274560018428,-2.00945370250361));
#22842=CARTESIAN_POINT('Ctrl Pts',(9.63650698268243,-3.76701036219998,-1.40778992375466));
#22843=CARTESIAN_POINT('Ctrl Pts',(9.61533341365661,-3.94654076027199,-0.703241061932939));
#22844=CARTESIAN_POINT('Ctrl Pts',(9.59415984463078,-3.94772861144879,0.000742196070642187));
#22845=CARTESIAN_POINT('Ctrl Pts',(9.48884015536925,-3.9476212151691,0.00031064949736361));
#22846=CARTESIAN_POINT('Ctrl Pts',(9.5092037286265,-3.94714379178427,-0.676787743548417));
#22847=CARTESIAN_POINT('Ctrl Pts',(9.52956730188374,-3.78180578893861,-1.35410472974234));
#22848=CARTESIAN_POINT('Ctrl Pts',(9.54993087514098,-3.45294297697788,-1.93956749021687));
#22849=CARTESIAN_POINT('Ctrl Pts',(9.58950361179499,-2.81386056798107,-3.07730315911534));
#22850=CARTESIAN_POINT('Ctrl Pts',(9.629076348449,-1.55723424482083,-3.86815557286639));
#22851=CARTESIAN_POINT('Ctrl Pts',(9.66864908510301,-0.255001929666197,
-3.95217804093306));
#22852=CARTESIAN_POINT('Ctrl Pts',(9.70822182175703,1.04723038548845,-4.03620050899974));
#22853=CARTESIAN_POINT('Ctrl Pts',(9.74779455841104,2.39506869263753,-3.41339303138206));
#22854=CARTESIAN_POINT('Ctrl Pts',(9.78736729506505,3.17506106370751,-2.36721872523338));
#22855=CARTESIAN_POINT('Ctrl Pts',(9.82694003171907,3.95505343477749,-1.32104441908469));
#22856=CARTESIAN_POINT('Ctrl Pts',(9.86651276837308,4.16719986976838,0.148496715594994));
#22857=CARTESIAN_POINT('Ctrl Pts',(9.90608550502709,3.7149445437798,1.37256121466685));
#22858=CARTESIAN_POINT('Ctrl Pts',(9.94565824168111,3.2626892177912,2.59662571373873));
#22859=CARTESIAN_POINT('Ctrl Pts',(9.98523097833512,2.14603213082312,3.57521357720275));
#22860=CARTESIAN_POINT('Ctrl Pts',(10.0248037149891,0.873205939095632,3.86293264752249));
#22861=CARTESIAN_POINT('Ctrl Pts',(10.0643764516431,-0.399620252631823,
4.15065171784221));
#22862=CARTESIAN_POINT('Ctrl Pts',(10.1039491882972,-1.82861554911865,3.74750199501769));
#22863=CARTESIAN_POINT('Ctrl Pts',(10.1435219249512,-2.76339042278715,2.83697208703492));
#22864=CARTESIAN_POINT('Ctrl Pts',(10.1752946684239,-3.51391628420185,2.10591238187753));
#22865=CARTESIAN_POINT('Ctrl Pts',(10.2070674118966,-3.94584788289007,1.04777510454963));
#22866=CARTESIAN_POINT('Ctrl Pts',(10.2388401553693,-3.95540412882742,-0.0034237005329492));
#22867=CARTESIAN_POINT('Origin',(4.7,0.,0.));
#22868=CARTESIAN_POINT('',(11.0941598446308,-3.95881660301891,0.00220458637196837));
#22869=CARTESIAN_POINT('',(10.9888401553692,-3.95819583346249,0.00255778193754717));
#22870=CARTESIAN_POINT('',(4.7,-3.954,-4.84225344382863E-16));
#22871=CARTESIAN_POINT('Ctrl Pts',(11.0941598446308,-3.95881660301891,0.00220458637196837));
#22872=CARTESIAN_POINT('Ctrl Pts',(11.0902062535048,-3.95969225385185,0.132715516968071));
#22873=CARTESIAN_POINT('Ctrl Pts',(11.0862526623788,-3.95379409173705,0.263146353242184));
#22874=CARTESIAN_POINT('Ctrl Pts',(11.0822990712527,-3.94086098162676,0.392875855157525));
#22875=CARTESIAN_POINT('Ctrl Pts',(11.0427263345987,-3.81140941615156,1.69137922890495));
#22876=CARTESIAN_POINT('Ctrl Pts',(11.0031535979447,-2.97715191209434,2.9196184555242));
#22877=CARTESIAN_POINT('Ctrl Pts',(10.9635808612907,-1.81779044977045,3.51857564858477));
#22878=CARTESIAN_POINT('Ctrl Pts',(10.9240081246367,-0.658428987446535,
4.11753284164536));
#22879=CARTESIAN_POINT('Ctrl Pts',(10.8844353879827,0.826036433144062,4.08720800114722));
#22880=CARTESIAN_POINT('Ctrl Pts',(10.8448626513286,1.95996974379351,3.44140310302274));
#22881=CARTESIAN_POINT('Ctrl Pts',(10.8052899146746,3.09390305444297,2.79559820489827));
#22882=CARTESIAN_POINT('Ctrl Pts',(10.7657171780206,3.87730425515128,1.53431324914745));
#22883=CARTESIAN_POINT('Ctrl Pts',(10.7261444413666,3.95361798280149,0.231606476917969));
#22884=CARTESIAN_POINT('Ctrl Pts',(10.6865717047126,4.0299317104517,-1.07110029531144));
#22885=CARTESIAN_POINT('Ctrl Pts',(10.6469989680586,3.39915796504391,-2.41522888401951));
#22886=CARTESIAN_POINT('Ctrl Pts',(10.6074262314046,2.34838561194535,-3.1890157935783));
#22887=CARTESIAN_POINT('Ctrl Pts',(10.5678534947506,1.29761325884674,-3.96280270313713));
#22888=CARTESIAN_POINT('Ctrl Pts',(10.5282807580965,-0.17315770194269,-4.16624793354662));
#22889=CARTESIAN_POINT('Ctrl Pts',(10.4887080214425,-1.39452406614718,-3.70675590550802));
#22890=CARTESIAN_POINT('Ctrl Pts',(10.4491352847885,-2.61589043035163,-3.24726387746944));
#22891=CARTESIAN_POINT('Ctrl Pts',(10.4095625481345,-3.58785219797115,-2.12483459098281));
#22892=CARTESIAN_POINT('Ctrl Pts',(10.3699898114805,-3.86803299700534,-0.850327847456766));
#22893=CARTESIAN_POINT('Ctrl Pts',(10.3613798225306,-3.92899298581659,-0.573028628191791));
#22894=CARTESIAN_POINT('Ctrl Pts',(10.3527698335807,-3.95720521240893,-0.288530314664122));
#22895=CARTESIAN_POINT('Ctrl Pts',(10.3441598446308,-3.95459914581543,-0.00352034347287922));
#22896=CARTESIAN_POINT('Ctrl Pts',(10.2388401553693,-3.95540412882742,-0.0034237005329492));
#22897=CARTESIAN_POINT('Ctrl Pts',(10.2466401485506,-3.95775012243715,-0.261485882632503));
#22898=CARTESIAN_POINT('Ctrl Pts',(10.2544401417319,-3.9346408534935,-0.519129904364567));
#22899=CARTESIAN_POINT('Ctrl Pts',(10.2622401349132,-3.88454086821667,-0.77141395795088));
#22900=CARTESIAN_POINT('Ctrl Pts',(10.3018128715672,-3.63036198912756,-2.0513600018129));
#22901=CARTESIAN_POINT('Ctrl Pts',(10.3413856082212,-2.68144978009919,-3.19334199639593));
#22902=CARTESIAN_POINT('Ctrl Pts',(10.3809583448752,-1.46968989174215,-3.67760096713576));
#22903=CARTESIAN_POINT('Ctrl Pts',(10.4205310815293,-0.257930003385074,
-4.1618599378756));
#22904=CARTESIAN_POINT('Ctrl Pts',(10.4601038181833,1.21667756430069,-3.9883958847722));
#22905=CARTESIAN_POINT('Ctrl Pts',(10.4996765548373,2.28298342288284,-3.23615882524473));
#22906=CARTESIAN_POINT('Ctrl Pts',(10.5392492914913,3.34928928146496,-2.48392176571727));
#22907=CARTESIAN_POINT('Ctrl Pts',(10.5788220281453,4.00729343094349,-1.15291169976578));
#22908=CARTESIAN_POINT('Ctrl Pts',(10.6183947647993,3.95751342447232,0.151078610293575));
#22909=CARTESIAN_POINT('Ctrl Pts',(10.6579675014533,3.90773341800116,1.45506892035293));
#22910=CARTESIAN_POINT('Ctrl Pts',(10.6975402381073,3.15016925558029,2.73203947452015));
#22911=CARTESIAN_POINT('Ctrl Pts',(10.7371129747614,2.02961689204451,3.40079292561223));
#22912=CARTESIAN_POINT('Ctrl Pts',(10.7766857114154,0.909064528508733,4.06954637670431));
#22913=CARTESIAN_POINT('Ctrl Pts',(10.8162584480694,-0.574476036141954,
4.13008272472125));
#22914=CARTESIAN_POINT('Ctrl Pts',(10.8558311847234,-1.74578967043865,3.55484959990684));
#22915=CARTESIAN_POINT('Ctrl Pts',(10.8954039213774,-2.91710330473538,2.97961647509242));
#22916=CARTESIAN_POINT('Ctrl Pts',(10.9349766580314,-3.77619000867811,1.76861387744662));
#22917=CARTESIAN_POINT('Ctrl Pts',(10.9745493946854,-3.93204709884383,0.473014654994837));
#22918=CARTESIAN_POINT('Ctrl Pts',(10.97931298158,-3.9508084698007,0.317056285709203));
#22919=CARTESIAN_POINT('Ctrl Pts',(10.9840765684746,-3.95937986467358,0.159872089799277));
#22920=CARTESIAN_POINT('Ctrl Pts',(10.9888401553692,-3.95819583346249,0.00255778193754717));
#22921=CARTESIAN_POINT('Origin',(4.7,0.,0.));
#22922=CARTESIAN_POINT('',(11.8441598446308,-3.9483118015039,0.00169262224176542));
#22923=CARTESIAN_POINT('',(11.7388401553692,-3.94800490926472,0.00129567598274352));
#22924=CARTESIAN_POINT('',(4.7,-3.954,-4.84225344382863E-16));
#22925=CARTESIAN_POINT('Ctrl Pts',(11.8441598446308,-3.9483118015039,0.00169262224176542));
#22926=CARTESIAN_POINT('Ctrl Pts',(11.8276426734288,-3.95044317207578,0.550656188455528));
#22927=CARTESIAN_POINT('Ctrl Pts',(11.8111255022269,-3.84369304308854,1.09882729481394));
#22928=CARTESIAN_POINT('Ctrl Pts',(11.794608331025,-3.62402854299927,1.59723318054838));
#22929=CARTESIAN_POINT('Ctrl Pts',(11.7550355943709,-3.09774439252394,2.79134109538696));
#22930=CARTESIAN_POINT('Ctrl Pts',(11.7154628577169,-1.92331841462687,3.6997907656419));
#22931=CARTESIAN_POINT('Ctrl Pts',(11.6758901210629,-0.635276061282561,
3.90911256430254));
#22932=CARTESIAN_POINT('Ctrl Pts',(11.6363173844089,0.652766292061783,4.11843436296318));
#22933=CARTESIAN_POINT('Ctrl Pts',(11.5967446477549,2.05442502085337,3.62862829002949));
#22934=CARTESIAN_POINT('Ctrl Pts',(11.5571719111009,2.93175249797369,2.66262351913797));
#22935=CARTESIAN_POINT('Ctrl Pts',(11.5175991744469,3.80907997509398,1.69661874824647));
#22936=CARTESIAN_POINT('Ctrl Pts',(11.4780264377928,4.16207620054304,0.254415279397177));
#22937=CARTESIAN_POINT('Ctrl Pts',(11.4384537011388,3.83007931013461,-1.00758582368442));
#22938=CARTESIAN_POINT('Ctrl Pts',(11.3988809644848,3.49808241972618,-2.26958692676602));
#22939=CARTESIAN_POINT('Ctrl Pts',(11.3593082278308,2.48109241346025,-3.35138566407993));
#22940=CARTESIAN_POINT('Ctrl Pts',(11.3197354911768,1.24197970898019,-3.76061472589476));
#22941=CARTESIAN_POINT('Ctrl Pts',(11.2801627545228,0.00286700450012237,
-4.16984378770958));
#22942=CARTESIAN_POINT('Ctrl Pts',(11.2405900178688,-1.45836839819409,-3.90650317402533));
#22943=CARTESIAN_POINT('Ctrl Pts',(11.2010172812148,-2.47666328609461,-3.09044910674541));
#22944=CARTESIAN_POINT('Ctrl Pts',(11.1653981356868,-3.39322344516725,-2.35592450625361));
#22945=CARTESIAN_POINT('Ctrl Pts',(11.1297789901588,-3.950927589346,-1.17360942213905));
#22946=CARTESIAN_POINT('Ctrl Pts',(11.0941598446308,-3.95881660301891,0.00220458637196837));
#22947=CARTESIAN_POINT('Ctrl Pts',(10.9888401553692,-3.95819583346249,0.00255778193754717));
#22948=CARTESIAN_POINT('Ctrl Pts',(11.0236493051287,-3.9495437146582,-1.14699137562275));
#22949=CARTESIAN_POINT('Ctrl Pts',(11.0584584548881,-3.41997896279796,-2.30348814970156));
#22950=CARTESIAN_POINT('Ctrl Pts',(11.0932676046475,-2.5390593592383,-3.0393938247008));
#22951=CARTESIAN_POINT('Ctrl Pts',(11.1328403413015,-1.53758705307831,-3.87600723468695));
#22952=CARTESIAN_POINT('Ctrl Pts',(11.1724130779555,-0.0820149643695929,
-4.16903820740154));
#22953=CARTESIAN_POINT('Ctrl Pts',(11.2119858146095,1.16517128117612,-3.78511732141781));
#22954=CARTESIAN_POINT('Ctrl Pts',(11.2515585512635,2.4123575267218,-3.4011964354341));
#22955=CARTESIAN_POINT('Ctrl Pts',(11.2911312879175,3.45115792910449,-2.34032369075211));
#22956=CARTESIAN_POINT('Ctrl Pts',(11.3307040245716,3.80877533873865,-1.08534219045179));
#22957=CARTESIAN_POINT('Ctrl Pts',(11.3702767612256,4.16639274837284,0.169639309848643));
#22958=CARTESIAN_POINT('Ctrl Pts',(11.4098494978796,3.84282716525836,1.61872956576745));
#22959=CARTESIAN_POINT('Ctrl Pts',(11.4494222345336,2.98534546091942,2.60239307759696));
#22960=CARTESIAN_POINT('Ctrl Pts',(11.4889949711876,2.12786375658053,3.58605658942642));
#22961=CARTESIAN_POINT('Ctrl Pts',(11.5285677078416,0.736465931017243,4.10429335716664));
#22962=CARTESIAN_POINT('Ctrl Pts',(11.5681404444956,-0.555570511864919,
3.9212343283417));
#22963=CARTESIAN_POINT('Ctrl Pts',(11.6077131811497,-1.84760695474708,3.73817529951676));
#22964=CARTESIAN_POINT('Ctrl Pts',(11.6472859178037,-3.04028201494811,2.85382047412666));
#22965=CARTESIAN_POINT('Ctrl Pts',(11.6868586544577,-3.59076439635125,1.6706730084585));
#22966=CARTESIAN_POINT('Ctrl Pts',(11.7041858214282,-3.83179650439823,1.1526245887188));
#22967=CARTESIAN_POINT('Ctrl Pts',(11.7215129883987,-3.94970869911457,0.577292233503969));
#22968=CARTESIAN_POINT('Ctrl Pts',(11.7388401553692,-3.94800490926472,0.00129567598274352));
#22969=CARTESIAN_POINT('Origin',(4.7,0.,0.));
#22970=CARTESIAN_POINT('',(12.5941598446308,-3.95274743352102,-0.003520024949899));
#22971=CARTESIAN_POINT('',(12.4888401553692,-3.95353526093205,-0.00355836282268518));
#22972=CARTESIAN_POINT('',(4.7,-3.954,-4.84225344382863E-16));
#22973=CARTESIAN_POINT('Ctrl Pts',(12.5941598446308,-3.95274743352102,-0.003520024949899));
#22974=CARTESIAN_POINT('Ctrl Pts',(12.5650790933529,-3.94431242632764,0.960271211073185));
#22975=CARTESIAN_POINT('Ctrl Pts',(12.5359983420751,-3.58899174946445,1.92963147645128));
#22976=CARTESIAN_POINT('Ctrl Pts',(12.5069175907972,-2.94886311311229,2.64366091296727));
#22977=CARTESIAN_POINT('Ctrl Pts',(12.4673448541432,-2.07778376206595,3.61530358424772));
#22978=CARTESIAN_POINT('Ctrl Pts',(12.4277721174892,-0.679313005392218,
4.11413894713976));
#22979=CARTESIAN_POINT('Ctrl Pts',(12.3881993808351,0.610052503064052,3.91312824619137));
#22980=CARTESIAN_POINT('Ctrl Pts',(12.3486266441811,1.89941801152032,3.71211754524298));
#22981=CARTESIAN_POINT('Ctrl Pts',(12.3090539075271,3.07967827175917,2.81126078045414));
#22982=CARTESIAN_POINT('Ctrl Pts',(12.2694811708731,3.61365242648782,1.62057176809711));
#22983=CARTESIAN_POINT('Ctrl Pts',(12.2299084342191,4.14762658121646,0.429882755740119));
#22984=CARTESIAN_POINT('Ctrl Pts',(12.1903356975651,4.03531463043501,-1.05063850418497));
#22985=CARTESIAN_POINT('Ctrl Pts',(12.1507629609111,3.32783397082584,-2.14715108281151));
#22986=CARTESIAN_POINT('Ctrl Pts',(12.111190224257,2.62035331121666,-3.24366366143806));
#22987=CARTESIAN_POINT('Ctrl Pts',(12.071617487603,1.31770394277974,-3.95616755876599));
#22988=CARTESIAN_POINT('Ctrl Pts',(12.032044750949,0.0127706062405369,-3.96037544027009));
#22989=CARTESIAN_POINT('Ctrl Pts',(11.992472014295,-1.29216273029871,-3.9645833217742));
#22990=CARTESIAN_POINT('Ctrl Pts',(11.952899277641,-2.59938003494028,-3.26049518745443));
#22991=CARTESIAN_POINT('Ctrl Pts',(11.913326540987,-3.31391752573424,-2.16856804058342));
#22992=CARTESIAN_POINT('Ctrl Pts',(11.8902709755349,-3.73021589880342,-1.53239778974413));
#22993=CARTESIAN_POINT('Ctrl Pts',(11.8672154100828,-3.94533671859644,-0.764580565636778));
#22994=CARTESIAN_POINT('Ctrl Pts',(11.8441598446308,-3.9483118015039,0.00169262224176542));
#22995=CARTESIAN_POINT('Ctrl Pts',(11.7388401553692,-3.94800490926472,0.00129567598274352));
#22996=CARTESIAN_POINT('Ctrl Pts',(11.7610857250527,-3.94581749017334,-0.738200375482764));
#22997=CARTESIAN_POINT('Ctrl Pts',(11.7833312947362,-3.74646900286499,-1.47879122073117));
#22998=CARTESIAN_POINT('Ctrl Pts',(11.8055768644197,-3.35737431122418,-2.10066060696583));
#22999=CARTESIAN_POINT('Ctrl Pts',(11.8451496010737,-2.6652121420887,-3.20690665077582));
#23000=CARTESIAN_POINT('Ctrl Pts',(11.8847223377277,-1.37259810121253,-3.93745863244953));
#23001=CARTESIAN_POINT('Ctrl Pts',(11.9242950743818,-0.0678494752439936,
-3.95981485683605));
#23002=CARTESIAN_POINT('Ctrl Pts',(11.9638678110358,1.23689915072447,-3.98217108122257));
#23003=CARTESIAN_POINT('Ctrl Pts',(12.0034405476898,2.55378236178524,-3.29633154832198));
#23004=CARTESIAN_POINT('Ctrl Pts',(12.0430132843438,3.2834370589297,-2.21444763560813));
#23005=CARTESIAN_POINT('Ctrl Pts',(12.0825860209978,4.01309175607421,-1.13256372289422));
#23006=CARTESIAN_POINT('Ctrl Pts',(12.1221587576518,4.1555179393023,0.345364569633074));
#23007=CARTESIAN_POINT('Ctrl Pts',(12.1617314943058,3.64589209342869,1.54667646725719));
#23008=CARTESIAN_POINT('Ctrl Pts',(12.2013042309598,3.1362662475551,2.74798836488128));
#23009=CARTESIAN_POINT('Ctrl Pts',(12.2408769676139,1.97458837257992,3.67268386760227));
#23010=CARTESIAN_POINT('Ctrl Pts',(12.2804497042679,0.689581779690363,3.89989925801654));
#23011=CARTESIAN_POINT('Ctrl Pts',(12.3200224409219,-0.595424813199232,
4.12711464843081));
#23012=CARTESIAN_POINT('Ctrl Pts',(12.3595951775759,-2.00376012400316,3.65684992653832));
#23013=CARTESIAN_POINT('Ctrl Pts',(12.3991679142299,-2.89443776269302,2.70314026365419));
#23014=CARTESIAN_POINT('Ctrl Pts',(12.4290586612764,-3.56719942258961,1.98276819188519));
#23015=CARTESIAN_POINT('Ctrl Pts',(12.4589494083228,-3.94461989025521,0.986574446948708));
#23016=CARTESIAN_POINT('Ctrl Pts',(12.4888401553692,-3.95353526093205,-0.00355836282268518));
#23017=CARTESIAN_POINT('Origin',(4.7,0.,0.));
#23018=CARTESIAN_POINT('',(13.3441598446308,-3.95992130118435,0.00122964282165419));
#23019=CARTESIAN_POINT('',(13.2388401553692,-3.95951177378463,0.0016722506470103));
#23020=CARTESIAN_POINT('',(4.7,-3.954,-4.84225344382863E-16));
#23021=CARTESIAN_POINT('Ctrl Pts',(13.3441598446308,-3.95992130118435,0.00122964282165419));
#23022=CARTESIAN_POINT('Ctrl Pts',(13.342088249931,-3.96020131501855,0.0695639880146641));
#23023=CARTESIAN_POINT('Ctrl Pts',(13.3400166552312,-3.9585846683956,0.137884811974986));
#23024=CARTESIAN_POINT('Ctrl Pts',(13.3379450605315,-3.95502961063748,0.206104619115586));
#23025=CARTESIAN_POINT('Ctrl Pts',(13.2983723238774,-3.88711895008823,1.50927674195507));
#23026=CARTESIAN_POINT('Ctrl Pts',(13.2587995872234,-3.11186785732278,2.77558708680145));
#23027=CARTESIAN_POINT('Ctrl Pts',(13.2192268505694,-1.9821229161865,3.42869127999069));
#23028=CARTESIAN_POINT('Ctrl Pts',(13.1796541139154,-0.852377975050223,
4.08179547317992));
#23029=CARTESIAN_POINT('Ctrl Pts',(13.1400813772614,0.63186081445685,4.12169351471201));
#23030=CARTESIAN_POINT('Ctrl Pts',(13.1005086406074,1.7950608697933,3.53022572037632));
#23031=CARTESIAN_POINT('Ctrl Pts',(13.0609359039534,2.95826092512974,2.93875792604063));
#23032=CARTESIAN_POINT('Ctrl Pts',(13.0213631672994,3.80042224629552,1.71592429583719));
#23033=CARTESIAN_POINT('Ctrl Pts',(12.9817904306453,3.93824535103146,0.418282733106529));
#23034=CARTESIAN_POINT('Ctrl Pts',(12.9422176939913,4.07606845576739,-0.879358829624127));
#23035=CARTESIAN_POINT('Ctrl Pts',(12.9026449573373,3.50955334407346,-2.25180832488194));
#23036=CARTESIAN_POINT('Ctrl Pts',(12.8630722206833,2.49654245255791,-3.07441250840861));
#23037=CARTESIAN_POINT('Ctrl Pts',(12.8234994840293,1.48353156104236,-3.89701669193528));
#23038=CARTESIAN_POINT('Ctrl Pts',(12.7839267473753,0.024024889705067,-4.1697755637308));
#23039=CARTESIAN_POINT('Ctrl Pts',(12.7443540107213,-1.21770120819094,-3.76854621331596));
#23040=CARTESIAN_POINT('Ctrl Pts',(12.7047812740673,-2.45942730608694,-3.36731686290113));
#23041=CARTESIAN_POINT('Ctrl Pts',(12.6652085374132,-3.48337283054174,-2.29209929027598));
#23042=CARTESIAN_POINT('Ctrl Pts',(12.6256358007592,-3.82350162005966,-1.03226551412899));
#23043=CARTESIAN_POINT('Ctrl Pts',(12.6151438153831,-3.91368053077872,-0.698243693215093));
#23044=CARTESIAN_POINT('Ctrl Pts',(12.6046518300069,-3.95579068268866,-0.351244313686516));
#23045=CARTESIAN_POINT('Ctrl Pts',(12.5941598446308,-3.95274743352102,-0.003520024949899));
#23046=CARTESIAN_POINT('Ctrl Pts',(12.4888401553692,-3.95353526093205,-0.00355836282268518));
#23047=CARTESIAN_POINT('Ctrl Pts',(12.4985221449768,-3.95642306183267,-0.324274856104691));
#23048=CARTESIAN_POINT('Ctrl Pts',(12.5082041345844,-3.92064753909048,-0.64435543987071));
#23049=CARTESIAN_POINT('Ctrl Pts',(12.5178861241919,-3.84372223884785,-0.954220416301001));
#23050=CARTESIAN_POINT('Ctrl Pts',(12.557458860846,-3.52930910973709,-2.22071682949655));
#23051=CARTESIAN_POINT('Ctrl Pts',(12.5970315975,-2.52746288493975,-3.316555052012));
#23052=CARTESIAN_POINT('Ctrl Pts',(12.636604334154,-1.29416147990325,-3.7429778691348));
#23053=CARTESIAN_POINT('Ctrl Pts',(12.676177070808,-0.0608600748667443,
-4.1694006862576));
#23054=CARTESIAN_POINT('Ctrl Pts',(12.715749807462,1.40389651040895,-3.92640809798775));
#23055=CARTESIAN_POINT('Ctrl Pts',(12.755322544116,2.43344244506891,-3.12459518761852));
#23056=CARTESIAN_POINT('Ctrl Pts',(12.79489528077,3.46298837972893,-2.32278227724925));
#23057=CARTESIAN_POINT('Ctrl Pts',(12.834468017424,4.05732366377315,-0.962149044780607));
#23058=CARTESIAN_POINT('Ctrl Pts',(12.8740407540781,3.94594393747885,0.338029155260154));
#23059=CARTESIAN_POINT('Ctrl Pts',(12.9136134907321,3.83456421118455,1.63820735530084));
#23060=CARTESIAN_POINT('Ctrl Pts',(12.9531862273861,3.01746947455173,2.87793052291361));
#23061=CARTESIAN_POINT('Ctrl Pts',(12.9927589640401,1.86655030411764,3.4929539495523));
#23062=CARTESIAN_POINT('Ctrl Pts',(13.0323317006941,0.715631133683578,4.10797737619097));
#23063=CARTESIAN_POINT('Ctrl Pts',(13.0719044373481,-0.769112470551771,
4.09830106185561));
#23064=CARTESIAN_POINT('Ctrl Pts',(13.1114771740021,-1.91191786172387,3.46832915347659));
#23065=CARTESIAN_POINT('Ctrl Pts',(13.1510499106561,-3.05472325289603,2.83835724509754));
#23066=CARTESIAN_POINT('Ctrl Pts',(13.1906226473102,-3.85559043100492,1.58808974267472));
#23067=CARTESIAN_POINT('Ctrl Pts',(13.2301953839642,-3.95001454631996,0.286570254467792));
#23068=CARTESIAN_POINT('Ctrl Pts',(13.2330769744325,-3.95689028082004,0.191796769773386));
#23069=CARTESIAN_POINT('Ctrl Pts',(13.2359585649009,-3.96002017282103,0.0967515266364028));
#23070=CARTESIAN_POINT('Ctrl Pts',(13.2388401553692,-3.95951177378463,0.0016722506470103));
#23071=CARTESIAN_POINT('Origin',(4.7,0.,0.));
#23072=CARTESIAN_POINT('',(14.0941598446308,-3.94932298134531,0.002498291375507));
#23073=CARTESIAN_POINT('',(13.9888401553692,-3.94884092925267,0.00217675990483683));
#23074=CARTESIAN_POINT('',(4.7,-3.954,-4.84225344382863E-16));
#23075=CARTESIAN_POINT('Ctrl Pts',(14.0941598446308,-3.94932298134531,0.002498291375507));
#23076=CARTESIAN_POINT('Ctrl Pts',(14.0795246698551,-3.95217299008822,0.488608263067992));
#23077=CARTESIAN_POINT('Ctrl Pts',(14.0648894950794,-3.86903917261975,0.973780078148339));
#23078=CARTESIAN_POINT('Ctrl Pts',(14.0502543203037,-3.69550476445004,1.4241105383856));
#23079=CARTESIAN_POINT('Ctrl Pts',(14.0106815836497,-3.22627692534584,2.64178022688495));
#23080=CARTESIAN_POINT('Ctrl Pts',(13.9711088469957,-2.09610060077861,3.60471329766544));
#23081=CARTESIAN_POINT('Ctrl Pts',(13.9315361103417,-0.819391906539967,
3.87469523990012));
#23082=CARTESIAN_POINT('Ctrl Pts',(13.8919633736876,0.457316787698675,4.14467718213481));
#23083=CARTESIAN_POINT('Ctrl Pts',(13.8523906370336,1.88055785160873,3.72170799582369));
#23084=CARTESIAN_POINT('Ctrl Pts',(13.8128179003796,2.80257668230365,2.7982692338459));
#23085=CARTESIAN_POINT('Ctrl Pts',(13.7732451637256,3.72459551299857,1.87483047186812));
#23086=CARTESIAN_POINT('Ctrl Pts',(13.7336724270716,4.14539211047836,0.450922134223676));
#23087=CARTESIAN_POINT('Ctrl Pts',(13.6940996904176,3.87343771936786,-0.825366984455388));
#23088=CARTESIAN_POINT('Ctrl Pts',(13.6545269537636,3.60148332825735,-2.10165610313449));
#23089=CARTESIAN_POINT('Ctrl Pts',(13.6149542171096,2.63677794855649,-3.2303260028482));
#23090=CARTESIAN_POINT('Ctrl Pts',(13.5753814804555,1.41839970925465,-3.69768418650959));
#23091=CARTESIAN_POINT('Ctrl Pts',(13.5358087438015,0.200021469952839,-4.16504237017096));
#23092=CARTESIAN_POINT('Ctrl Pts',(13.4962360071475,-1.27202962894994,-3.97108883778006));
#23093=CARTESIAN_POINT('Ctrl Pts',(13.4566632704935,-2.32777006423482,-3.20409512116832));
#23094=CARTESIAN_POINT('Ctrl Pts',(13.4191621285393,-3.328243503224,-2.4772527878683));
#23095=CARTESIAN_POINT('Ctrl Pts',(13.381660986585,-3.95485233738253,-1.23579610343927));
#23096=CARTESIAN_POINT('Ctrl Pts',(13.3441598446308,-3.95992130118435,0.00122964282165419));
#23097=CARTESIAN_POINT('Ctrl Pts',(13.2388401553692,-3.95951177378463,0.0016722506470103));
#23098=CARTESIAN_POINT('Ctrl Pts',(13.2755313015549,-3.95303835448019,-1.20896737801102));
#23099=CARTESIAN_POINT('Ctrl Pts',(13.3122224477405,-3.35669606630255,-2.42512468514771));
#23100=CARTESIAN_POINT('Ctrl Pts',(13.3489135939262,-2.39251067506772,-3.15604663613086));
#23101=CARTESIAN_POINT('Ctrl Pts',(13.3884863305802,-1.35260163597929,-3.9443725645315));
#23102=CARTESIAN_POINT('Ctrl Pts',(13.4280590672342,0.115197494718774,-4.16825294734179));
#23103=CARTESIAN_POINT('Ctrl Pts',(13.4676318038883,1.3428363327277,-3.72579203267733));
#23104=CARTESIAN_POINT('Ctrl Pts',(13.5072045405423,2.57047517073663,-3.28333111801288));
#23105=CARTESIAN_POINT('Ctrl Pts',(13.5467772771963,3.55795371605642,-2.17452890587367));
#23106=CARTESIAN_POINT('Ctrl Pts',(13.5863500138503,3.85583289315453,-0.90404179728785));
#23107=CARTESIAN_POINT('Ctrl Pts',(13.6259227505043,4.15371207025265,0.366445311297973));
#23108=CARTESIAN_POINT('Ctrl Pts',(13.6654954871583,3.7619918791291,1.79861731633042));
#23109=CARTESIAN_POINT('Ctrl Pts',(13.7050682238123,2.85895974354046,2.74063655681762));
#23110=CARTESIAN_POINT('Ctrl Pts',(13.7446409604664,1.9559276079518,3.68265579730486));
#23111=CARTESIAN_POINT('Ctrl Pts',(13.7842136971204,0.541583527898016,4.13452227324683));
#23112=CARTESIAN_POINT('Ctrl Pts',(13.8237864337744,-0.74035285927286,3.89057891177458));
#23113=CARTESIAN_POINT('Ctrl Pts',(13.8633591704284,-2.0222892464437,3.64663555030234));
#23114=CARTESIAN_POINT('Ctrl Pts',(13.9029319070824,-3.17181794073164,2.70688235141592));
#23115=CARTESIAN_POINT('Ctrl Pts',(13.9425046437364,-3.66574219400503,1.4990280587802));
#23116=CARTESIAN_POINT('Ctrl Pts',(13.9579498142807,-3.85851997418385,1.0276046213389));
#23117=CARTESIAN_POINT('Ctrl Pts',(13.973394984825,-3.95142773522678,0.515340610393162));
#23118=CARTESIAN_POINT('Ctrl Pts',(13.9888401553692,-3.94884092925267,0.00217675990483683));
#23119=CARTESIAN_POINT('Origin',(4.7,0.,0.));
#23120=CARTESIAN_POINT('',(14.8441598446308,-3.95012252210193,-0.00484157028959653));
#23121=CARTESIAN_POINT('',(14.7388401553692,-3.95165589089271,-0.00363582964324092));
#23122=CARTESIAN_POINT('',(4.7,-3.954,-4.84225344382863E-16));
#23123=CARTESIAN_POINT('Ctrl Pts',(14.8441598446308,-3.95012252210193,-0.00484157028959653));
#23124=CARTESIAN_POINT('Ctrl Pts',(14.8169610897792,-3.94332577709582,0.897842123970638));
#23125=CARTESIAN_POINT('Ctrl Pts',(14.7897623349275,-3.63714466198666,1.80607102634386));
#23126=CARTESIAN_POINT('Ctrl Pts',(14.7625635800759,-3.07096454601399,2.50195343740126));
#23127=CARTESIAN_POINT('Ctrl Pts',(14.7229908434219,-2.24720269550416,3.51442520477352));
#23128=CARTESIAN_POINT('Ctrl Pts',(14.6834181067679,-0.873056840637845,
4.07738712090295));
#23129=CARTESIAN_POINT('Ctrl Pts',(14.6438453701139,0.424568275462648,3.93721918519319));
#23130=CARTESIAN_POINT('Ctrl Pts',(14.6042726334599,1.72219339156307,3.79705124948343));
#23131=CARTESIAN_POINT('Ctrl Pts',(14.5646998968058,2.94329776889771,2.95375346193458));
#23132=CARTESIAN_POINT('Ctrl Pts',(14.5251271601518,3.53287076796465,1.78982106701354));
#23133=CARTESIAN_POINT('Ctrl Pts',(14.4855544234978,4.12244376703158,0.625888672092527));
#23134=CARTESIAN_POINT('Ctrl Pts',(14.4459816868438,4.08048538783091,-0.85867833020057));
#23135=CARTESIAN_POINT('Ctrl Pts',(14.4064089501898,3.425694963339,-1.98750853586906));
#23136=CARTESIAN_POINT('Ctrl Pts',(14.3668362135358,2.77090453884704,-3.11633874153765));
#23137=CARTESIAN_POINT('Ctrl Pts',(14.3272634768818,1.5032820690637,-3.88943215058149));
#23138=CARTESIAN_POINT('Ctrl Pts',(14.2876907402278,0.199979015819173,-3.95528655559086));
#23139=CARTESIAN_POINT('Ctrl Pts',(14.2481180035737,-1.10332403742528,-4.02114096060022));
#23140=CARTESIAN_POINT('Ctrl Pts',(14.2085452669197,-2.44230767413093,-3.37975636157519));
#23141=CARTESIAN_POINT('Ctrl Pts',(14.1689725302657,-3.20765981566317,-2.32286090895358));
#23142=CARTESIAN_POINT('Ctrl Pts',(14.1440349683874,-3.68996197623994,-1.65683682325276));
#23143=CARTESIAN_POINT('Ctrl Pts',(14.1190974065091,-3.94446671755144,-0.825807327419405));
#23144=CARTESIAN_POINT('Ctrl Pts',(14.0941598446308,-3.94932298134531,0.002498291375507));
#23145=CARTESIAN_POINT('Ctrl Pts',(13.9888401553692,-3.94884092925267,0.00217675990483683));
#23146=CARTESIAN_POINT('Ctrl Pts',(14.012967721479,-3.94479996823029,-0.799458592213253));
#23147=CARTESIAN_POINT('Ctrl Pts',(14.0370952875887,-3.70772447792752,-1.60328981463878));
#23148=CARTESIAN_POINT('Ctrl Pts',(14.0612228536984,-3.25429404769414,-2.25705948968798));
#23149=CARTESIAN_POINT('Ctrl Pts',(14.1007955903525,-2.51060183585106,-3.32933735913542));
#23150=CARTESIAN_POINT('Ctrl Pts',(14.1403683270065,-1.18489759990609,-3.99793771164533));
#23151=CARTESIAN_POINT('Ctrl Pts',(14.1799410636605,0.119451583199217,-3.95858537939921));
#23152=CARTESIAN_POINT('Ctrl Pts',(14.2195138003145,1.42380076630463,-3.91923304715309));
#23153=CARTESIAN_POINT('Ctrl Pts',(14.2590865369685,2.70679489657038,-3.1719280301508));
#23154=CARTESIAN_POINT('Ctrl Pts',(14.2986592736225,3.3844745259588,-2.05673988602559));
#23155=CARTESIAN_POINT('Ctrl Pts',(14.3382320102765,4.06215415534718,-0.941551741900444));
#23156=CARTESIAN_POINT('Ctrl Pts',(14.3778047469306,4.1345192838583,0.541519529347578));
#23157=CARTESIAN_POINT('Ctrl Pts',(14.4173774835846,3.56867289191554,1.71736384111271));
#23158=CARTESIAN_POINT('Ctrl Pts',(14.4569502202386,3.00282649997279,2.89320815287784));
#23159=CARTESIAN_POINT('Ctrl Pts',(14.4965229568926,1.79876858757616,3.76182550516009));
#23160=CARTESIAN_POINT('Ctrl Pts',(14.5360956935466,0.504436900763993,3.92808191777024));
#23161=CARTESIAN_POINT('Ctrl Pts',(14.5756684302006,-0.789894786048174,
4.09433833038039));
#23162=CARTESIAN_POINT('Ctrl Pts',(14.6152411668546,-2.17450024727588,3.55823380331844));
#23163=CARTESIAN_POINT('Ctrl Pts',(14.6548139035086,-3.01905207823151,2.56337686971723));
#23164=CARTESIAN_POINT('Ctrl Pts',(14.6828226541288,-3.61680809965312,1.85923805820075));
#23165=CARTESIAN_POINT('Ctrl Pts',(14.710831404749,-3.94402368019253,0.925286740362676));
#23166=CARTESIAN_POINT('Ctrl Pts',(14.7388401553692,-3.95165589089271,-0.00363582964324092));
#23167=CARTESIAN_POINT('Origin',(-7.03243520205041,0.,0.));
#23168=CARTESIAN_POINT('',(14.3425647979496,-3.51958190579553,0.00222644264931085));
#23169=CARTESIAN_POINT('',(14.4904352020504,-3.52166096245149,-0.00324020098756483));
#23170=CARTESIAN_POINT('',(-7.03243520205041,-3.52375,3.2169090177286E-13));
#23171=CARTESIAN_POINT('',(15.,-2.52120044613813,2.46936361140965));
#23172=CARTESIAN_POINT('Ctrl Pts',(14.3425647979496,-3.51958190579553,0.00222644264931099));
#23173=CARTESIAN_POINT('Ctrl Pts',(14.3675023598279,-3.5152540708073,-0.735948045016053));
#23174=CARTESIAN_POINT('Ctrl Pts',(14.4320126583603,-2.92852262828258,-2.65179107551659));
#23175=CARTESIAN_POINT('Ctrl Pts',(14.5360956935466,0.210016568782032,-4.155178159011));
#23176=CARTESIAN_POINT('Ctrl Pts',(14.6548139035087,3.59907929859906,-2.08826776438434));
#23177=CARTESIAN_POINT('Ctrl Pts',(14.7735321134707,3.7112574766783,1.88080884739934));
#23178=CARTESIAN_POINT('Ctrl Pts',(14.8885941456345,0.547106722347347,4.06597940294392));
#23179=CARTESIAN_POINT('Ctrl Pts',(14.9640834411443,-1.7769695191295,3.21936428498554));
#23180=CARTESIAN_POINT('Ctrl Pts',(15.,-2.52120044613813,2.46936361140965));
#23181=CARTESIAN_POINT('',(15.,1.51195443948857,3.18289299779474));
#23182=CARTESIAN_POINT('Origin',(15.,0.,0.));
#23183=CARTESIAN_POINT('Ctrl Pts',(14.4904352020504,-3.52166096245149,-0.00324020098756532));
#23184=CARTESIAN_POINT('Ctrl Pts',(14.5019991880842,-3.52446919194943,-0.345032096527443));
#23185=CARTESIAN_POINT('Ctrl Pts',(14.553135910772,-3.32220045815802,-1.85308063959033));
#23186=CARTESIAN_POINT('Ctrl Pts',(14.6438453701139,-1.17267268992146,-3.99072892597622));
#23187=CARTESIAN_POINT('Ctrl Pts',(14.7625635800759,2.70983253704952,-3.16081271422384));
#23188=CARTESIAN_POINT('Ctrl Pts',(14.881281790038,4.12213179013054,0.556374543543842));
#23189=CARTESIAN_POINT('Ctrl Pts',(14.960427263346,2.56715916810242,2.68164414176901));
#23190=CARTESIAN_POINT('Ctrl Pts',(15.,1.51195443948848,3.18289299779479));
#23191=CARTESIAN_POINT('Origin',(-7.03243520205041,0.,0.));
#23192=CARTESIAN_POINT('',(13.5925647979496,-3.52902698154992,0.00109584064080212));
#23193=CARTESIAN_POINT('',(13.7404352020504,-3.51915230765151,0.00193989825877733));
#23194=CARTESIAN_POINT('',(-7.03243520205041,-3.52375,3.2169090177286E-13));
#23195=CARTESIAN_POINT('Ctrl Pts',(13.5925647979496,-3.52902698154992,0.00109584064080225));
#23196=CARTESIAN_POINT('Ctrl Pts',(13.6300659399038,-3.52450959126252,-1.10132436001352));
#23197=CARTESIAN_POINT('Ctrl Pts',(13.7071398185121,-2.37681150026024,-3.37517909858378));
#23198=CARTESIAN_POINT('Ctrl Pts',(13.8237864337744,1.49012789947011,-3.88467673536986));
#23199=CARTESIAN_POINT('Ctrl Pts',(13.9425046437364,4.06932409197459,-0.867111819500367));
#23200=CARTESIAN_POINT('Ctrl Pts',(14.0612228536985,2.9442998048962,2.93979030855331));
#23201=CARTESIAN_POINT('Ctrl Pts',(14.1799410636605,-0.860818327845137,
4.07062313879903));
#23202=CARTESIAN_POINT('Ctrl Pts',(14.2737217117442,-3.2477048593109,2.03694757208693));
#23203=CARTESIAN_POINT('Ctrl Pts',(14.3279296231739,-3.52212179408783,0.435440912237356));
#23204=CARTESIAN_POINT('Ctrl Pts',(14.3425647979496,-3.51958190579553,0.00222644264931099));
#23205=CARTESIAN_POINT('Ctrl Pts',(13.7404352020504,-3.51915230765151,0.00193989825877757));
#23206=CARTESIAN_POINT('Ctrl Pts',(13.7645627681601,-3.51555105919362,-0.712466417377603));
#23207=CARTESIAN_POINT('Ctrl Pts',(13.8282630709239,-2.95774521056077,-2.60377013928517));
#23208=CARTESIAN_POINT('Ctrl Pts',(13.9315361103417,0.125484922544878,-4.15875404743734));
#23209=CARTESIAN_POINT('Ctrl Pts',(14.0502543203037,3.55564468470245,-2.16079042553925));
#23210=CARTESIAN_POINT('Ctrl Pts',(14.1689725302657,3.74911708348173,1.80428726191164));
#23211=CARTESIAN_POINT('Ctrl Pts',(14.2876907402278,0.529997911397081,4.12658649947203));
#23212=CARTESIAN_POINT('Ctrl Pts',(14.394844964156,-2.81124210751884,2.83289385539345));
#23213=CARTESIAN_POINT('Ctrl Pts',(14.4624264514302,-3.51485924205318,0.824602719108089));
#23214=CARTESIAN_POINT('Ctrl Pts',(14.4904352020504,-3.52166096245149,-0.00324020098756532));
#23215=CARTESIAN_POINT('Origin',(-7.03243520205041,0.,0.));
#23216=CARTESIAN_POINT('',(12.8425647979496,-3.52263373011373,-0.00313699744994253));
#23217=CARTESIAN_POINT('',(12.9904352020504,-3.52866201640708,0.00149028660038811));
#23218=CARTESIAN_POINT('',(-7.03243520205041,-3.52375,3.2169090177286E-13));
#23219=CARTESIAN_POINT('Ctrl Pts',(12.8425647979496,-3.52263373011373,-0.00313699744994185));
#23220=CARTESIAN_POINT('Ctrl Pts',(12.8530567833258,-3.52534583159438,-0.313024064327951));
#23221=CARTESIAN_POINT('Ctrl Pts',(12.9031215053559,-3.34627313867605,-1.78863292620238));
#23222=CARTESIAN_POINT('Ctrl Pts',(12.9927589640401,-1.2792814688989,-3.95912511815523));
#23223=CARTESIAN_POINT('Ctrl Pts',(13.1114771740022,2.62279488400284,-3.22988833933176));
#23224=CARTESIAN_POINT('Ctrl Pts',(13.2301953839642,4.1374061319782,0.439435567280381));
#23225=CARTESIAN_POINT('Ctrl Pts',(13.3489135939262,1.88583863921803,3.70875271783386));
#23226=CARTESIAN_POINT('Ctrl Pts',(13.4676318038883,-2.08236047650701,3.60208297288041));
#23227=CARTESIAN_POINT('Ctrl Pts',(13.5488488718961,-3.50031412078277,1.28596967099022));
#23228=CARTESIAN_POINT('Ctrl Pts',(13.5904932032498,-3.52927652599813,0.0619944620048905));
#23229=CARTESIAN_POINT('Ctrl Pts',(13.5925647979496,-3.52902698154992,0.00109584064080225));
#23230=CARTESIAN_POINT('Ctrl Pts',(12.9904352020504,-3.52866201640708,0.00149028660038825));
#23231=CARTESIAN_POINT('Ctrl Pts',(13.0271263482361,-3.5228929948406,-1.07741497174151));
#23232=CARTESIAN_POINT('Ctrl Pts',(13.1033902310757,-2.41825070574393,-3.33017956397349));
#23233=CARTESIAN_POINT('Ctrl Pts',(13.2192268505694,1.41074465321508,-3.91420835157396));
#23234=CARTESIAN_POINT('Ctrl Pts',(13.3379450605315,4.05082623445229,-0.949760859141879));
#23235=CARTESIAN_POINT('Ctrl Pts',(13.4566632704935,3.00353941846475,2.8792346664523));
#23236=CARTESIAN_POINT('Ctrl Pts',(13.5753814804555,-0.777792108158467,
4.08732608875924));
#23237=CARTESIAN_POINT('Ctrl Pts',(13.6699721243078,-3.2265189232229,2.08546317825473));
#23238=CARTESIAN_POINT('Ctrl Pts',(13.7249900315061,-3.52145763328409,0.459264409679643));
#23239=CARTESIAN_POINT('Ctrl Pts',(13.7404352020504,-3.51915230765151,0.00193989825877757));
#23240=CARTESIAN_POINT('Origin',(-7.03243520205041,0.,0.));
#23241=CARTESIAN_POINT('',(12.0925647979496,-3.5186807563352,0.00150844148329803));
#23242=CARTESIAN_POINT('',(12.2404352020504,-3.52333583098364,-0.00317116363052899));
#23243=CARTESIAN_POINT('',(-7.03243520205041,-3.52375,3.2169090177286E-13));
#23244=CARTESIAN_POINT('Ctrl Pts',(12.0925647979496,-3.5186807563352,0.00150844148329801));
#23245=CARTESIAN_POINT('Ctrl Pts',(12.1156203634017,-3.51602940368091,-0.68138360348061));
#23246=CARTESIAN_POINT('Ctrl Pts',(12.1782486655078,-2.99525967935504,-2.54013425586182));
#23247=CARTESIAN_POINT('Ctrl Pts',(12.2804497042679,0.0134164280071953,
-4.16065529676554));
#23248=CARTESIAN_POINT('Ctrl Pts',(12.3991679142299,3.49612561771096,-2.25573450146264));
#23249=CARTESIAN_POINT('Ctrl Pts',(12.5178861241919,3.79639817959729,1.70252558174023));
#23250=CARTESIAN_POINT('Ctrl Pts',(12.636604334154,0.640903420859428,4.11101877212304));
#23251=CARTESIAN_POINT('Ctrl Pts',(12.7448305587399,-2.76755685483373,2.89521893475459));
#23252=CARTESIAN_POINT('Ctrl Pts',(12.8134840466717,-3.51511656860697,0.855780394542055));
#23253=CARTESIAN_POINT('Ctrl Pts',(12.8425647979496,-3.52263373011373,-0.00313699744994185));
#23254=CARTESIAN_POINT('Ctrl Pts',(12.2404352020504,-3.52333583098364,-0.00317116363052868));
#23255=CARTESIAN_POINT('Ctrl Pts',(12.250117191658,-3.52590939912316,-0.28898925751087));
#23256=CARTESIAN_POINT('Ctrl Pts',(12.2993719179196,-3.36371430659345,-1.74013506675719));
#23257=CARTESIAN_POINT('Ctrl Pts',(12.3881993808351,-1.35960842341351,-3.93226373321093));
#23258=CARTESIAN_POINT('Ctrl Pts',(12.5069175907972,2.55650388111248,-3.28260885239469));
#23259=CARTESIAN_POINT('Ctrl Pts',(12.6256358007592,4.14549398517236,0.355123585322626));
#23260=CARTESIAN_POINT('Ctrl Pts',(12.7443540107213,1.96094347059736,3.66959590085791));
#23261=CARTESIAN_POINT('Ctrl Pts',(12.8630722206833,-2.008605296796,3.64372570917414));
#23262=CARTESIAN_POINT('Ctrl Pts',(12.9450992844597,-3.48802023705692,1.33414869944489));
#23263=CARTESIAN_POINT('Ctrl Pts',(12.987553611582,-3.52911509458222,0.0862236196220098));
#23264=CARTESIAN_POINT('Ctrl Pts',(12.9904352020504,-3.52866201640708,0.00149028660038825));
#23265=CARTESIAN_POINT('Origin',(-7.03243520205041,0.,0.));
#23266=CARTESIAN_POINT('',(11.3425647979496,-3.52804248985531,0.00196469682072595));
#23267=CARTESIAN_POINT('',(11.4904352020504,-3.51840725822498,0.00115468847878691));
#23268=CARTESIAN_POINT('',(-7.03243520205041,-3.52375,3.2169090177286E-13));
#23269=CARTESIAN_POINT('Ctrl Pts',(11.3425647979496,-3.52804248985531,0.00196469682072596));
#23270=CARTESIAN_POINT('Ctrl Pts',(11.3781839434776,-3.52101191020695,-1.04590445150779));
#23271=CARTESIAN_POINT('Ctrl Pts',(11.4533758256596,-2.4718083520435,-3.27018269306563));
#23272=CARTESIAN_POINT('Ctrl Pts',(11.5681404444956,1.30478777373567,-3.9507924973221));
#23273=CARTESIAN_POINT('Ctrl Pts',(11.6868586544577,4.02376996992659,-1.05854037242841));
#23274=CARTESIAN_POINT('Ctrl Pts',(11.8055768644197,3.0800139384955,2.79727485773682));
#23275=CARTESIAN_POINT('Ctrl Pts',(11.9242950743818,-0.66740256042652,4.10680000910255));
#23276=CARTESIAN_POINT('Ctrl Pts',(12.0199577188917,-3.19751819588237,2.14968840054265));
#23277=CARTESIAN_POINT('Ctrl Pts',(12.0760476267477,-3.52058020424936,0.490737163396706));
#23278=CARTESIAN_POINT('Ctrl Pts',(12.0925647979496,-3.5186807563352,0.00150844148329801));
#23279=CARTESIAN_POINT('Ctrl Pts',(11.4904352020504,-3.51840725822498,0.00115468847878698));
#23280=CARTESIAN_POINT('Ctrl Pts',(11.5126807717339,-3.51645786064706,-0.657873943628404));
#23281=CARTESIAN_POINT('Ctrl Pts',(11.5744990780714,-3.02276716911119,-2.4919626366133));
#23282=CARTESIAN_POINT('Ctrl Pts',(11.6758901210629,-0.071280686042087,
-4.16006636356011));
#23283=CARTESIAN_POINT('Ctrl Pts',(11.7946083310249,3.44948351348419,-2.32643430433509));
#23284=CARTESIAN_POINT('Ctrl Pts',(11.913326540987,3.83026823514579,1.62489332904317));
#23285=CARTESIAN_POINT('Ctrl Pts',(12.032044750949,0.724454569027592,4.09712077799104));
#23286=CARTESIAN_POINT('Ctrl Pts',(12.1410809713035,-2.73373818088755,2.94237727385996));
#23287=CARTESIAN_POINT('Ctrl Pts',(12.210544455004,-3.51539057619789,0.879221473807933));
#23288=CARTESIAN_POINT('Ctrl Pts',(12.2404352020504,-3.52333583098364,-0.00317116363052868));
#23289=CARTESIAN_POINT('Origin',(-7.03243520205041,0.,0.));
#23290=CARTESIAN_POINT('',(10.5925647979496,-3.52428395044692,-0.00313728131290625));
#23291=CARTESIAN_POINT('',(10.7404352020504,-3.52748926863011,0.00227945981369715));
#23292=CARTESIAN_POINT('',(-7.03243520205041,-3.52375,3.2169090177286E-13));
#23293=CARTESIAN_POINT('Ctrl Pts',(10.5925647979496,-3.52428395044692,-0.00313728131290616));
#23294=CARTESIAN_POINT('Ctrl Pts',(10.6011747868995,-3.5266064408766,-0.25713421757632));
#23295=CARTESIAN_POINT('Ctrl Pts',(10.6493575125034,-3.38590629208833,-1.6759855412164));
#23296=CARTESIAN_POINT('Ctrl Pts',(10.7371129747614,-1.46504644039007,-3.89420998646693));
#23297=CARTESIAN_POINT('Ctrl Pts',(10.8558311847234,2.46714564844276,-3.35028727732022));
#23298=CARTESIAN_POINT('Ctrl Pts',(10.9745493946854,4.1535561077605,0.243319031071492));
#23299=CARTESIAN_POINT('Ctrl Pts',(11.0932676046475,2.05908722991844,3.61543804687332));
#23300=CARTESIAN_POINT('Ctrl Pts',(11.2119858146095,-1.90971779724849,3.69651327957846));
#23301=CARTESIAN_POINT('Ctrl Pts',(11.2950848790436,-3.47095393416288,1.39797660948795));
#23302=CARTESIAN_POINT('Ctrl Pts',(11.3386112068236,-3.52882285774164,0.118274229366946));
#23303=CARTESIAN_POINT('Ctrl Pts',(11.3425647979496,-3.52804248985531,0.00196469682072596));
#23304=CARTESIAN_POINT('Ctrl Pts',(10.7404352020504,-3.52748926863011,0.00227945981369699));
#23305=CARTESIAN_POINT('Ctrl Pts',(10.7752443518098,-3.51977862026482,-1.02218281736217));
#23306=CARTESIAN_POINT('Ctrl Pts',(10.8496262382232,-2.51131260490639,-3.22453425679115));
#23307=CARTESIAN_POINT('Ctrl Pts',(10.9635808612907,1.22409507255686,-3.97653421179419));
#23308=CARTESIAN_POINT('Ctrl Pts',(11.0822990712527,4.00138863696973,-1.14022895073704));
#23309=CARTESIAN_POINT('Ctrl Pts',(11.2010172812148,3.13631714721284,2.73399850699711));
#23310=CARTESIAN_POINT('Ctrl Pts',(11.3197354911768,-0.583666227467498,
4.11953478190202));
#23311=CARTESIAN_POINT('Ctrl Pts',(11.4162081314553,-3.17485254267083,2.19819996255183));
#23312=CARTESIAN_POINT('Ctrl Pts',(11.4731080350799,-3.51992565212565,0.514474837584795));
#23313=CARTESIAN_POINT('Ctrl Pts',(11.4904352020504,-3.51840725822498,0.00115468847878698));
#23314=CARTESIAN_POINT('Origin',(-7.03243520205041,0.,0.));
#23315=CARTESIAN_POINT('',(9.84256479794961,-3.51816102544073,0.000661434852013216));
#23316=CARTESIAN_POINT('',(9.99043520205041,-3.52500134015064,-0.00305115446425308));
#23317=CARTESIAN_POINT('',(-7.03243520205041,-3.52375,3.2169090177286E-13));
#23318=CARTESIAN_POINT('Ctrl Pts',(9.84256479794961,-3.51816102544073,0.000661434852013316));
#23319=CARTESIAN_POINT('Ctrl Pts',(9.86373836697544,-3.5171024289349,-0.626718687907311));
#23320=CARTESIAN_POINT('Ctrl Pts',(9.92448467265527,-3.05808178285527,-2.42809871725697));
#23321=CARTESIAN_POINT('Ctrl Pts',(10.0248037149891,-0.183323073196887,
-4.15663627733209));
#23322=CARTESIAN_POINT('Ctrl Pts',(10.1435219249512,3.3855596180177,-2.41851577709298));
#23323=CARTESIAN_POINT('Ctrl Pts',(10.2622401349132,3.87265117113374,1.52111978421037));
#23324=CARTESIAN_POINT('Ctrl Pts',(10.3809583448753,0.834564199366861,4.07611764898101));
#23325=CARTESIAN_POINT('Ctrl Pts',(10.4910665658874,-2.68777420777237,3.00452075401946));
#23326=CARTESIAN_POINT('Ctrl Pts',(10.5616020502455,-3.51593194376749,0.910271911299991));
#23327=CARTESIAN_POINT('Ctrl Pts',(10.5925647979496,-3.52428395044692,-0.00313728131290616));
#23328=CARTESIAN_POINT('Ctrl Pts',(9.99043520205041,-3.52500134015064,-0.00305115446425291));
#23329=CARTESIAN_POINT('Ctrl Pts',(9.99823519523173,-3.52709205714162,-0.233032594568881));
#23330=CARTESIAN_POINT('Ctrl Pts',(10.0456079250671,-3.40201178448786,-1.62754596340236));
#23331=CARTESIAN_POINT('Ctrl Pts',(10.1325533915564,-1.54401347143674,-3.86358065584526));
#23332=CARTESIAN_POINT('Ctrl Pts',(10.2512716015185,2.3984360100751,-3.39981437578226));
#23333=CARTESIAN_POINT('Ctrl Pts',(10.3699898114805,4.15764854552659,0.158718795611215));
#23334=CARTESIAN_POINT('Ctrl Pts',(10.4887080214425,2.13225649899359,3.57277417516111));
#23335=CARTESIAN_POINT('Ctrl Pts',(10.6074262314046,-1.83407587178631,3.73462163822996));
#23336=CARTESIAN_POINT('Ctrl Pts',(10.6913352916072,-3.45744840424911,1.4462515066276));
#23337=CARTESIAN_POINT('Ctrl Pts',(10.7356716151558,-3.52854446083548,0.142475790700775));
#23338=CARTESIAN_POINT('Ctrl Pts',(10.7404352020504,-3.52748926863011,0.00227945981369699));
#23339=CARTESIAN_POINT('Origin',(-7.03243520205041,0.,0.));
#23340=CARTESIAN_POINT('',(9.09256479794961,-3.52666944689073,0.00262945503923755));
#23341=CARTESIAN_POINT('',(9.24043520205041,-3.51806531536473,0.000276846526976737));
#23342=CARTESIAN_POINT('',(-7.03243520205041,-3.52375,3.2169090177286E-13));
#23343=CARTESIAN_POINT('Ctrl Pts',(9.09256479794961,-3.52666944689073,0.00262945503923759));
#23344=CARTESIAN_POINT('Ctrl Pts',(9.12630194705135,-3.51838375617842,-0.990886089246301));
#23345=CARTESIAN_POINT('Ctrl Pts',(9.19961183280712,-2.56233043718894,-3.16372988524757));
#23346=CARTESIAN_POINT('Ctrl Pts',(9.31249445521691,1.11652672540754,-4.00806693589946));
#23347=CARTESIAN_POINT('Ctrl Pts',(9.43121266517893,3.96921968490559,-1.24760874642564));
#23348=CARTESIAN_POINT('Ctrl Pts',(9.54993087514098,3.20883019120772,2.64851681044191));
#23349=CARTESIAN_POINT('Ctrl Pts',(9.66864908510301,-0.472478016872994,
4.1337630574056));
#23350=CARTESIAN_POINT('Ctrl Pts',(9.76619372603923,-3.14384070009375,2.26236328063938));
#23351=CARTESIAN_POINT('Ctrl Pts',(9.82416563032143,-3.51908091261411,0.545835091270507));
#23352=CARTESIAN_POINT('Ctrl Pts',(9.84256479794961,-3.51816102544073,0.000661434852013316));
#23353=CARTESIAN_POINT('Ctrl Pts',(9.24043520205041,-3.51806531536473,0.000276846526976876));
#23354=CARTESIAN_POINT('Ctrl Pts',(9.26079877530765,-3.51763984226101,-0.60314385718963));
#23355=CARTESIAN_POINT('Ctrl Pts',(9.3207350852189,-3.08395212212633,-2.3797714594065));
#23356=CARTESIAN_POINT('Ctrl Pts',(9.42024413178417,-0.267897613543705,
-4.1520433466978));
#23357=CARTESIAN_POINT('Ctrl Pts',(9.53896234174623,3.33562684382852,-2.48693116972114));
#23358=CARTESIAN_POINT('Ctrl Pts',(9.65768055170824,3.90281273176416,1.44197290715868));
#23359=CARTESIAN_POINT('Ctrl Pts',(9.77639876167031,0.917364772580788,4.05828473104436));
#23360=CARTESIAN_POINT('Ctrl Pts',(9.88731697845101,-2.652123974148,3.05125664466314));
#23361=CARTESIAN_POINT('Ctrl Pts',(9.95866245857771,-3.51648494621486,0.933762651658492));
#23362=CARTESIAN_POINT('Ctrl Pts',(9.99043520205041,-3.52500134015064,-0.00305115446425291));
#23363=CARTESIAN_POINT('Origin',(-7.03243520205041,0.,0.));
#23364=CARTESIAN_POINT('',(8.34256479794962,-3.52593087787563,-0.00285764939352675));
#23365=CARTESIAN_POINT('',(8.49043520205041,-3.52600078018851,0.00283908784911309));
#23366=CARTESIAN_POINT('',(-7.03243520205041,-3.52375,3.2169090177286E-13));
#23367=CARTESIAN_POINT('Ctrl Pts',(8.34256479794962,-3.52593087787563,-0.00285764939352656));
#23368=CARTESIAN_POINT('Ctrl Pts',(8.34929279047327,-3.52767436669035,-0.201096201058421));
#23369=CARTESIAN_POINT('Ctrl Pts',(8.39559351965095,-3.42246428829984,-1.56348475987019));
#23370=CARTESIAN_POINT('Ctrl Pts',(8.48146698548262,-1.64753430101277,-3.82058414619887));
#23371=CARTESIAN_POINT('Ctrl Pts',(8.60018519544467,2.305977735937,-3.46319204962163));
#23372=CARTESIAN_POINT('Ctrl Pts',(8.7189034054067,4.16041530571664,0.0466580663793381));
#23373=CARTESIAN_POINT('Ctrl Pts',(8.83762161536874,2.22772978017945,3.5140364991988));
#23374=CARTESIAN_POINT('Ctrl Pts',(8.95633982533078,-1.73280303479793,3.78267446838806));
#23375=CARTESIAN_POINT('Ctrl Pts',(9.04132088619107,-3.43875275553379,1.51020068927361));
#23376=CARTESIAN_POINT('Ctrl Pts',(9.08672921039734,-3.5281026407103,0.174479984724652));
#23377=CARTESIAN_POINT('Ctrl Pts',(9.09256479794961,-3.52666944689073,0.00262945503923759));
#23378=CARTESIAN_POINT('Ctrl Pts',(8.49043520205041,-3.52600078018851,0.0028390878491133));
#23379=CARTESIAN_POINT('Ctrl Pts',(8.52336235538358,-3.51750136365036,-0.967301129892824));
#23380=CARTESIAN_POINT('Ctrl Pts',(8.59586224537075,-2.59993141150347,-3.11751026790667));
#23381=CARTESIAN_POINT('Ctrl Pts',(8.70793487201195,1.03470715069641,-4.02996454035241));
#23382=CARTESIAN_POINT('Ctrl Pts',(8.82665308197397,3.9430009766923,-1.32814772597166));
#23383=CARTESIAN_POINT('Ctrl Pts',(8.94537129193603,3.26207859074647,2.58264909579165));
#23384=CARTESIAN_POINT('Ctrl Pts',(9.06408950189805,-0.388233209948286,
4.14252435827397));
#23385=CARTESIAN_POINT('Ctrl Pts',(9.16244413860286,-3.11963096819313,2.31080554513191));
#23386=CARTESIAN_POINT('Ctrl Pts',(9.22122603865364,-3.51846666842133,0.569489663367105));
#23387=CARTESIAN_POINT('Ctrl Pts',(9.24043520205041,-3.51806531536473,0.000276846526976876));
#23388=CARTESIAN_POINT('Origin',(-7.03243520205041,0.,0.));
#23389=CARTESIAN_POINT('',(7.59256479794961,-3.51805992519622,-0.000237397935153123));
#23390=CARTESIAN_POINT('',(7.74043520205041,-3.52660313318512,-0.00265300288022408));
#23391=CARTESIAN_POINT('',(-7.03243520205041,-3.52375,3.2169090177286E-13));
#23392=CARTESIAN_POINT('Ctrl Pts',(7.59256479794961,-3.51805992519622,-0.000237397935152622));
#23393=CARTESIAN_POINT('Ctrl Pts',(7.61185637054919,-3.51840553530387,-0.571894346614677));
#23394=CARTESIAN_POINT('Ctrl Pts',(7.67072067980279,-3.11712991020214,-2.31573181407069));
#23395=CARTESIAN_POINT('Ctrl Pts',(7.76915772571038,-0.379652508136737,
-4.14331949821216));
#23396=CARTESIAN_POINT('Ctrl Pts',(7.88787593567244,3.26742063740621,-2.57588720045187));
#23397=CARTESIAN_POINT('Ctrl Pts',(8.00659414563445,3.940241635325,1.33631147059774));
#23398=CARTESIAN_POINT('Ctrl Pts',(8.12531235559652,1.02635818146356,4.03209887955918));
#23399=CARTESIAN_POINT('Ctrl Pts',(8.23730257303488,-2.60371145120387,3.11279511355487));
#23400=CARTESIAN_POINT('Ctrl Pts',(8.30972005381926,-3.51741950634657,0.964904202795411));
#23401=CARTESIAN_POINT('Ctrl Pts',(8.34256479794962,-3.52593087787563,-0.00285764939352656));
#23402=CARTESIAN_POINT('Ctrl Pts',(7.74043520205041,-3.52660313318512,-0.00265300288022373));
#23403=CARTESIAN_POINT('Ctrl Pts',(7.74635319880549,-3.52806540306219,-0.17693892227022));
#23404=CARTESIAN_POINT('Ctrl Pts',(7.79184393221457,-3.43727644157581,-1.51511944087091));
#23405=CARTESIAN_POINT('Ctrl Pts',(7.87690740227768,-1.7249647945704,-3.78625534554826));
#23406=CARTESIAN_POINT('Ctrl Pts',(7.9956256122397,2.2350031991217,-3.50941502021571));
#23407=CARTESIAN_POINT('Ctrl Pts',(8.11434382220176,4.16050309010526,-0.0380410492039316));
#23408=CARTESIAN_POINT('Ctrl Pts',(8.23306203216378,2.2987999778154,3.46796074749932));
#23409=CARTESIAN_POINT('Ctrl Pts',(8.35178024212583,-1.65544386605393,3.81716369711131));
#23410=CARTESIAN_POINT('Ctrl Pts',(8.4375712987547,-3.42399640853641,1.55856250352173));
#23411=CARTESIAN_POINT('Ctrl Pts',(8.48378961872956,-3.52771619057371,0.198639422748347));
#23412=CARTESIAN_POINT('Ctrl Pts',(8.49043520205041,-3.52600078018851,0.0028390878491133));
#23413=CARTESIAN_POINT('Origin',(-7.03243520205041,0.,0.));
#23414=CARTESIAN_POINT('',(6.84256479794961,-3.52507380456061,0.00303947481950978));
#23415=CARTESIAN_POINT('',(6.99043520205041,-3.51814775897504,-0.000622653609956558));
#23416=CARTESIAN_POINT('',(-7.03243520205041,-3.52375,3.2169090177286E-13));
#23417=CARTESIAN_POINT('Ctrl Pts',(6.84256479794961,-3.52507380456061,0.00303947481950992));
#23418=CARTESIAN_POINT('Ctrl Pts',(6.87441995062511,-3.51654838502914,-0.936154325939411));
#23419=CARTESIAN_POINT('Ctrl Pts',(6.94584783995463,-2.6484521526581,-3.05600034132353));
#23420=CARTESIAN_POINT('Ctrl Pts',(7.05684846593816,0.925768177301577,-4.05637594079931));
#23421=CARTESIAN_POINT('Ctrl Pts',(7.1755666759002,3.90579086153378,-1.43388641013115));
#23422=CARTESIAN_POINT('Ctrl Pts',(7.29428488586224,3.33046878081729,2.49383443540284));
#23423=CARTESIAN_POINT('Ctrl Pts',(7.41300309582428,-0.276496612222895,
4.15147950911829));
#23424=CARTESIAN_POINT('Ctrl Pts',(7.51242973318673,-3.08654526745354,2.37485148050317));
#23425=CARTESIAN_POINT('Ctrl Pts',(7.57228363389518,-3.51769658647637,0.600743589964055));
#23426=CARTESIAN_POINT('Ctrl Pts',(7.59256479794961,-3.51805992519622,-0.000237397935152622));
#23427=CARTESIAN_POINT('Ctrl Pts',(6.99043520205041,-3.51814775897504,-0.000622653609956524));
#23428=CARTESIAN_POINT('Ctrl Pts',(7.00891677888141,-3.5190174026022,-0.548243313944348));
#23429=CARTESIAN_POINT('Ctrl Pts',(7.06697109236642,-3.1414084095468,-2.26729354051509));
#23430=CARTESIAN_POINT('Ctrl Pts',(7.16459814250543,-0.463915294938845,
-4.13473284304098));
#23431=CARTESIAN_POINT('Ctrl Pts',(7.28331635246748,3.21430888617722,-2.64186514955669));
#23432=CARTESIAN_POINT('Ctrl Pts',(7.40203456242951,3.96662723246049,1.25582701153581));
#23433=CARTESIAN_POINT('Ctrl Pts',(7.52075277239156,1.1082229708534,4.01037092188151));
#23434=CARTESIAN_POINT('Ctrl Pts',(7.63355298559851,-2.5661931577787,3.15903810143261));
#23435=CARTESIAN_POINT('Ctrl Pts',(7.70678046215147,-3.51828742866349,0.988484290341461));
#23436=CARTESIAN_POINT('Ctrl Pts',(7.74043520205041,-3.52660313318512,-0.00265300288022373));
#23437=CARTESIAN_POINT('Origin',(-7.03243520205041,0.,0.));
#23438=CARTESIAN_POINT('',(6.09256479794961,-3.52742942371994,-0.00230914916092352));
#23439=CARTESIAN_POINT('',(6.24043520205041,-3.52435719309002,0.00313090232885352));
#23440=CARTESIAN_POINT('',(-7.03243520205041,-3.52375,3.2169090177286E-13));
#23441=CARTESIAN_POINT('Ctrl Pts',(6.09256479794962,-3.52742942371994,-0.00230914916092399));
#23442=CARTESIAN_POINT('Ctrl Pts',(6.09741079404703,-3.52851335812002,-0.144937184098135));
#23443=CARTESIAN_POINT('Ctrl Pts',(6.14182952679845,-3.45604450642565,-1.45116517618719));
#23444=CARTESIAN_POINT('Ctrl Pts',(6.22582099620389,-1.82633687898537,-3.73841224260482));
#23445=CARTESIAN_POINT('Ctrl Pts',(6.34453920616593,2.13965170336266,-3.56835019014346));
#23446=CARTESIAN_POINT('Ctrl Pts',(6.46325741612797,4.15796828993553,-0.15010726528171));
#23447=CARTESIAN_POINT('Ctrl Pts',(6.58197562609,2.39138923910093,3.40477458847308));
#23448=CARTESIAN_POINT('Ctrl Pts',(6.70069383605204,-1.55201225656202,3.86037439203516));
#23449=CARTESIAN_POINT('Ctrl Pts',(6.78755689333858,-3.40361868355192,1.62261932332329));
#23450=CARTESIAN_POINT('Ctrl Pts',(6.8348472139711,-3.52713926762263,0.230579022449037));
#23451=CARTESIAN_POINT('Ctrl Pts',(6.84256479794961,-3.52507380456061,0.00303947481950992));
#23452=CARTESIAN_POINT('Ctrl Pts',(6.24043520205041,-3.52435719309002,0.00313090232885352));
#23453=CARTESIAN_POINT('Ctrl Pts',(6.27148035895733,-3.51598245699914,-0.912660575939013));
#23454=CARTESIAN_POINT('Ctrl Pts',(6.34209825251826,-2.68418353073412,-3.00928463009835));
#23455=CARTESIAN_POINT('Ctrl Pts',(6.45228888273322,0.843004746942437,-4.07438045361901));
#23456=CARTESIAN_POINT('Ctrl Pts',(6.57100709269524,3.87579342533039,-1.51309563754761));
#23457=CARTESIAN_POINT('Ctrl Pts',(6.68972530265728,3.38054326260136,2.42552269292219));
#23458=CARTESIAN_POINT('Ctrl Pts',(6.80844351261932,-0.191931774030066,
4.15624774024814));
#23459=CARTESIAN_POINT('Ctrl Pts',(6.90868014575036,-3.06074569025441,2.42318458251062));
#23460=CARTESIAN_POINT('Ctrl Pts',(6.9693440422274,-3.51715532240443,0.624321580051326));
#23461=CARTESIAN_POINT('Ctrl Pts',(6.99043520205041,-3.51814775897504,-0.000622653609956524));
#23462=CARTESIAN_POINT('Origin',(-7.03243520205041,0.,0.));
#23463=CARTESIAN_POINT('',(5.34256479794961,-3.51838353120525,-0.0011176602703349));
#23464=CARTESIAN_POINT('',(5.49043520205041,-3.52798931335802,-0.00199855428895335));
#23465=CARTESIAN_POINT('',(-7.03243520205041,-3.52375,3.2169090177286E-13));
#23466=CARTESIAN_POINT('Ctrl Pts',(5.34256479794961,-3.51838353120525,-0.00111766027033496));
#23467=CARTESIAN_POINT('Ctrl Pts',(5.35997437412294,-3.51985964985165,-0.516887860646145));
#23468=CARTESIAN_POINT('Ctrl Pts',(5.41695668695029,-3.17250968493244,-2.20313420046544));
#23469=CARTESIAN_POINT('Ctrl Pts',(5.51351173643166,-0.575132718389392,
-4.12073474606626));
#23470=CARTESIAN_POINT('Ctrl Pts',(5.63222994639369,3.14197293576922,-2.72749675748542));
#23471=CARTESIAN_POINT('Ctrl Pts',(5.75094815635573,3.99901838065921,1.14851403228232));
#23472=CARTESIAN_POINT('Ctrl Pts',(5.86966636631777,1.21585635703487,3.97906092065169));
#23473=CARTESIAN_POINT('Ctrl Pts',(5.9835385801824,-2.51528550301645,3.21987535772615));
#23474=CARTESIAN_POINT('Ctrl Pts',(6.05783805739301,-3.51966187543159,1.01977313604934));
#23475=CARTESIAN_POINT('Ctrl Pts',(6.09256479794962,-3.52742942371994,-0.00230914916092399));
#23476=CARTESIAN_POINT('Ctrl Pts',(5.49043520205041,-3.52798931335802,-0.00199855428895362));
#23477=CARTESIAN_POINT('Ctrl Pts',(5.49447120237924,-3.52879682472288,-0.120737180229964));
#23478=CARTESIAN_POINT('Ctrl Pts',(5.53807993936208,-3.46960409793346,-1.40288631934378));
#23479=CARTESIAN_POINT('Ctrl Pts',(5.62126141299893,-1.90205763486351,-3.70046076021046));
#23480=CARTESIAN_POINT('Ctrl Pts',(5.73997962296098,2.06657102730044,-3.61116563914235));
#23481=CARTESIAN_POINT('Ctrl Pts',(5.85869783292301,4.15405122458681,-0.23471580200077));
#23482=CARTESIAN_POINT('Ctrl Pts',(5.97741604288506,2.46020139211735,3.35539002120827));
#23483=CARTESIAN_POINT('Ctrl Pts',(6.09613425284709,-1.47310888518228,3.89116734368968));
#23484=CARTESIAN_POINT('Ctrl Pts',(6.18380730590221,-3.38757081640289,1.67105601217906));
#23485=CARTESIAN_POINT('Ctrl Pts',(6.23190762230332,-3.52665759150933,0.254683338866837));
#23486=CARTESIAN_POINT('Ctrl Pts',(6.24043520205041,-3.52435719309002,0.00313090232885352));
#23487=CARTESIAN_POINT('Origin',(-7.03243520205041,0.,0.));
#23488=CARTESIAN_POINT('',(4.59256479794961,-3.5234081221446,0.00317178002406706));
#23489=CARTESIAN_POINT('',(4.74043520205041,-3.51864963524456,-0.00147337684491794));
#23490=CARTESIAN_POINT('',(-7.03243520205041,-3.52375,3.2169090177286E-13));
#23491=CARTESIAN_POINT('Ctrl Pts',(4.59256479794961,-3.5234081221446,0.00317178002406677));
#23492=CARTESIAN_POINT('Ctrl Pts',(4.62253795419887,-3.51542475237107,-0.88160719352955));
#23493=CARTESIAN_POINT('Ctrl Pts',(4.69208384710213,-2.73025360675707,-2.94716560832423));
#23494=CARTESIAN_POINT('Ctrl Pts',(4.80120247665942,0.732938827149255,-4.09561145213467));
#23495=CARTESIAN_POINT('Ctrl Pts',(4.91992068662146,3.83362538042524,-1.61695668889399));
#23496=CARTESIAN_POINT('Ctrl Pts',(5.0386388965835,3.44465762033206,2.33357373354433));
#23497=CARTESIAN_POINT('Ctrl Pts',(5.15735710654553,-0.0798967268727354,
4.15990973510661));
#23498=CARTESIAN_POINT('Ctrl Pts',(5.25866574033425,-3.02552579319884,2.4870573681738));
#23499=CARTESIAN_POINT('Ctrl Pts',(5.32040163746893,-3.51650436688079,0.655480616923154));
#23500=CARTESIAN_POINT('Ctrl Pts',(5.34256479794961,-3.51838353120525,-0.00111766027033496));
#23501=CARTESIAN_POINT('Ctrl Pts',(4.74043520205041,-3.51864963524456,-0.00147337684491766));
#23502=CARTESIAN_POINT('Ctrl Pts',(4.75703478245516,-3.52051321359516,-0.493153923345435));
#23503=CARTESIAN_POINT('Ctrl Pts',(4.81320709951392,-3.19524209899379,-2.15462497466647));
#23504=CARTESIAN_POINT('Ctrl Pts',(4.90895215322669,-0.658895268659781,
-4.10817357339461));
#23505=CARTESIAN_POINT('Ctrl Pts',(5.02767036318875,3.08580101037766,-2.79088968046971));
#23506=CARTESIAN_POINT('Ctrl Pts',(5.14638857315077,4.02156899374811,1.06687202265491));
#23507=CARTESIAN_POINT('Ctrl Pts',(5.26510678311282,1.29660224356769,3.95348652535647));
#23508=CARTESIAN_POINT('Ctrl Pts',(5.37978899274602,-2.47586534144427,3.2655505474875));
#23509=CARTESIAN_POINT('Ctrl Pts',(5.45489846572523,-3.52087922512356,1.04348779305868));
#23510=CARTESIAN_POINT('Ctrl Pts',(5.49043520205041,-3.52798931335802,-0.00199855428895362));
#23511=CARTESIAN_POINT('Origin',(-7.03243520205041,0.,0.));
#23512=CARTESIAN_POINT('',(3.84256479794961,-3.52861952000803,-0.00152880647882163));
#23513=CARTESIAN_POINT('',(3.99043520205041,-3.52270430891722,0.00314279080041127));
#23514=CARTESIAN_POINT('',(-7.03243520205041,-3.52375,3.2169090177286E-13));
#23515=CARTESIAN_POINT('Ctrl Pts',(3.84256479794961,-3.52861952000803,-0.00152880647882115));
#23516=CARTESIAN_POINT('Ctrl Pts',(3.84552879762077,-3.52909571181233,-0.0886881604188186));
#23517=CARTESIAN_POINT('Ctrl Pts',(3.88806553394595,-3.48674052690646,-1.33905274392585));
#23518=CARTESIAN_POINT('Ctrl Pts',(3.97017500692515,-2.00105422024427,-3.6478780816856));
#23519=CARTESIAN_POINT('Ctrl Pts',(4.08889321688719,1.96853959665618,-3.66552647618271));
#23520=CARTESIAN_POINT('Ctrl Pts',(4.20761142684923,4.14622053401822,-0.346536829911929));
#23521=CARTESIAN_POINT('Ctrl Pts',(4.32632963681127,2.54969952546351,3.28789671690745));
#23522=CARTESIAN_POINT('Ctrl Pts',(4.4450478467733,-1.3677498639029,3.92943924765267));
#23523=CARTESIAN_POINT('Ctrl Pts',(4.53379290048609,-3.36545606309109,1.73520207145909));
#23524=CARTESIAN_POINT('Ctrl Pts',(4.58296521754485,-3.52596497666484,0.286542234120801));
#23525=CARTESIAN_POINT('Ctrl Pts',(4.59256479794961,-3.5234081221446,0.00317178002406677));
#23526=CARTESIAN_POINT('Ctrl Pts',(3.99043520205041,-3.52270430891722,0.0031427908004112));
#23527=CARTESIAN_POINT('Ctrl Pts',(4.01959836253108,-3.51513941180095,-0.858164720925442));
#23528=CARTESIAN_POINT('Ctrl Pts',(4.08833425966577,-2.76415178313285,-2.90002446236997));
#23529=CARTESIAN_POINT('Ctrl Pts',(4.19664289345446,0.649416670297701,-4.10968259997526));
#23530=CARTESIAN_POINT('Ctrl Pts',(4.3153611034165,3.79991631591589,-1.69465898523452));
#23531=CARTESIAN_POINT('Ctrl Pts',(4.43407931337854,3.49144617539216,2.26297076616989));
#23532=CARTESIAN_POINT('Ctrl Pts',(4.55279752334059,0.00479898395836184,
4.16067423069304));
#23533=CARTESIAN_POINT('Ctrl Pts',(4.65491615289787,-2.99809103350652,2.53523688571456));
#23534=CARTESIAN_POINT('Ctrl Pts',(4.71746204580115,-3.51607051724355,0.678992860497283));
#23535=CARTESIAN_POINT('Ctrl Pts',(4.74043520205041,-3.51864963524456,-0.00147337684491766));
#23536=CARTESIAN_POINT('Origin',(-7.03243520205041,0.,0.));
#23537=CARTESIAN_POINT('',(3.09256479794961,-3.51911232364593,-0.00191002701478894));
#23538=CARTESIAN_POINT('',(3.24043520205041,-3.52899431355517,-0.00113694359771377));
#23539=CARTESIAN_POINT('',(-7.03243520205041,-3.52375,3.2169090177286E-13));
#23540=CARTESIAN_POINT('Ctrl Pts',(3.09256479794961,-3.51911232364593,-0.00191002701478871));
#23541=CARTESIAN_POINT('Ctrl Pts',(3.1080923776967,-3.52139001070197,-0.461686364954821));
#23542=CARTESIAN_POINT('Ctrl Pts',(3.1631926940978,-3.22432754532709,-2.09039597570537));
#23543=CARTESIAN_POINT('Ctrl Pts',(3.25786574715292,-0.769326444574681,
-4.08893253953619));
#23544=CARTESIAN_POINT('Ctrl Pts',(3.37658395711495,3.0094971204592,-2.87300532076558));
#23545=CARTESIAN_POINT('Ctrl Pts',(3.495302167077,4.04884993253241,0.958147543456581));
#23546=CARTESIAN_POINT('Ctrl Pts',(3.61402037703903,1.40263484759868,3.9171224100737));
#23547=CARTESIAN_POINT('Ctrl Pts',(3.72977458732991,-2.42241976690523,3.32558458753253));
#23548=CARTESIAN_POINT('Ctrl Pts',(3.80595606096676,-3.52273801445775,1.07498746139492));
#23549=CARTESIAN_POINT('Ctrl Pts',(3.84256479794961,-3.52861952000803,-0.00152880647882115));
#23550=CARTESIAN_POINT('Ctrl Pts',(3.24043520205041,-3.52899431355517,-0.00113694359771367));
#23551=CARTESIAN_POINT('Ctrl Pts',(3.24258920595299,-3.52926239189115,-0.0644596887891739));
#23552=CARTESIAN_POINT('Ctrl Pts',(3.28431594650959,-3.49908651487518,-1.29086897191188));
#23553=CARTESIAN_POINT('Ctrl Pts',(3.3656154237202,-2.07489586267471,-3.60638880921834));
#23554=CARTESIAN_POINT('Ctrl Pts',(3.48433363368223,1.89351625165984,-3.70483863196498));
#23555=CARTESIAN_POINT('Ctrl Pts',(3.60305184364428,4.13830738080923,-0.430865531390001));
#23556=CARTESIAN_POINT('Ctrl Pts',(3.72177005360631,2.6160997115818,3.23531379981317));
#23557=CARTESIAN_POINT('Ctrl Pts',(3.84048826356835,-1.28747878468051,3.95646704310772));
#23558=CARTESIAN_POINT('Ctrl Pts',(3.93004331304971,-3.34807439860695,1.78369783221634));
#23559=CARTESIAN_POINT('Ctrl Pts',(3.98002562587707,-3.52540454344179,0.310580187989291));
#23560=CARTESIAN_POINT('Ctrl Pts',(3.99043520205041,-3.52270430891722,0.0031427908004112));
#23561=CARTESIAN_POINT('Origin',(-7.03243520205041,0.,0.));
#23562=CARTESIAN_POINT('',(2.34256479794961,-3.52180846607991,0.00302771658732861));
#23563=CARTESIAN_POINT('',(2.49043520205041,-3.51954048850984,-0.00220771176014323));
#23564=CARTESIAN_POINT('',(-7.03243520205041,-3.52375,3.2169090177286E-13));
#23565=CARTESIAN_POINT('Ctrl Pts',(2.34256479794961,-3.52180846607991,0.00302771658732888));
#23566=CARTESIAN_POINT('Ctrl Pts',(2.37065595777262,-3.51492881311082,-0.827155541520102));
#23567=CARTESIAN_POINT('Ctrl Pts',(2.43831985424964,-2.80782098383424,-2.83738688689506));
#23568=CARTESIAN_POINT('Ctrl Pts',(2.54555648738068,0.538470004761492,-4.12568570605805));
#23569=CARTESIAN_POINT('Ctrl Pts',(2.66427469734272,3.75288466474145,-1.79641008245562));
#23570=CARTESIAN_POINT('Ctrl Pts',(2.78299290730476,3.55114128675486,2.16809318358432));
#23571=CARTESIAN_POINT('Ctrl Pts',(2.9017111172668,0.116881875255089,4.15903487824236));
#23572=CARTESIAN_POINT('Ctrl Pts',(3.00490174748175,-2.96067738920047,2.59887469195073));
#23573=CARTESIAN_POINT('Ctrl Pts',(3.06851964104268,-3.51558522260769,0.71007434968313));
#23574=CARTESIAN_POINT('Ctrl Pts',(3.09256479794961,-3.51911232364593,-0.00191002701478871));
#23575=CARTESIAN_POINT('Ctrl Pts',(2.49043520205041,-3.51954048850984,-0.00220771176014333));
#23576=CARTESIAN_POINT('Ctrl Pts',(2.50515278602891,-3.52205463920765,-0.437866834869524));
#23577=CARTESIAN_POINT('Ctrl Pts',(2.55944310666143,-3.24555974650898,-2.04185136506832));
#23578=CARTESIAN_POINT('Ctrl Pts',(2.65330616394796,-0.852401394279078,
-4.07242494678922));
#23579=CARTESIAN_POINT('Ctrl Pts',(2.77202437391,2.95039066892461,-2.93367141734082));
#23580=CARTESIAN_POINT('Ctrl Pts',(2.89074258387204,4.06751511929676,0.875530603972367));
#23581=CARTESIAN_POINT('Ctrl Pts',(3.00946079383408,1.48208121505632,3.88775878317795));
#23582=CARTESIAN_POINT('Ctrl Pts',(3.12602499989353,-2.38106696512148,3.37061275541135));
#23583=CARTESIAN_POINT('Ctrl Pts',(3.20301646929898,-3.52433733424402,1.09888746980545));
#23584=CARTESIAN_POINT('Ctrl Pts',(3.24043520205041,-3.52899431355517,-0.00113694359771367));
#23585=CARTESIAN_POINT('Origin',(-7.03243520205041,0.,0.));
#23586=CARTESIAN_POINT('',(1.59256479794961,-3.5293292687682,-0.000582581467793654));
#23587=CARTESIAN_POINT('',(1.74043520205041,-3.52117028029313,0.00288554803045085));
#23588=CARTESIAN_POINT('',(-7.03243520205041,-3.52375,3.2169090177286E-13));
#23589=CARTESIAN_POINT('Ctrl Pts',(1.59256479794961,-3.5293292687682,-0.000582581467793819));
#23590=CARTESIAN_POINT('Ctrl Pts',(1.59364680119453,-3.52940256225382,-0.032382903366644));
#23591=CARTESIAN_POINT('Ctrl Pts',(1.63430154109346,-3.51464154093268,-1.22716522922806));
#23592=CARTESIAN_POINT('Ctrl Pts',(1.71452901764641,-2.17129550877666,-3.54918417453448));
#23593=CARTESIAN_POINT('Ctrl Pts',(1.83324722760845,1.7930241674711,-3.7545035392265));
#23594=CARTESIAN_POINT('Ctrl Pts',(1.95196543757049,4.12519831590081,-0.54219124457039));
#23595=CARTESIAN_POINT('Ctrl Pts',(2.07068364753253,2.70230652333086,3.16366432245317));
#23596=CARTESIAN_POINT('Ctrl Pts',(2.18940185749457,-1.18042802365586,3.98971454770484));
#23597=CARTESIAN_POINT('Ctrl Pts',(2.28002890763359,-3.32416575786672,1.84790964055073));
#23598=CARTESIAN_POINT('Ctrl Pts',(2.33108322111861,-3.52462035653345,0.342344886893788));
#23599=CARTESIAN_POINT('Ctrl Pts',(2.34256479794961,-3.52180846607991,0.00302771658732888));
#23600=CARTESIAN_POINT('Ctrl Pts',(1.74043520205041,-3.52117028029313,0.00288554803045071));
#23601=CARTESIAN_POINT('Ctrl Pts',(1.76771636610483,-3.51488727156751,-0.803729878337304));
#23602=CARTESIAN_POINT('Ctrl Pts',(1.83457026681328,-2.83992472367244,-2.78988645498181));
#23603=CARTESIAN_POINT('Ctrl Pts',(1.94099690417573,0.454375947728439,-4.13579201391049));
#23604=CARTESIAN_POINT('Ctrl Pts',(2.05971511413777,3.71553937395602,-1.87243163954858));
#23605=CARTESIAN_POINT('Ctrl Pts',(2.17843332409981,3.594539256238,2.09535691937294));
#23606=CARTESIAN_POINT('Ctrl Pts',(2.29715153406184,0.201519007352503,4.15579392822546));
#23607=CARTESIAN_POINT('Ctrl Pts',(2.40115216004538,-2.93156287124292,2.64685160308012));
#23608=CARTESIAN_POINT('Ctrl Pts',(2.4655800493749,-3.51529457426641,0.733536282306892));
#23609=CARTESIAN_POINT('Ctrl Pts',(2.49043520205041,-3.51954048850984,-0.00220771176014333));
#23610=CARTESIAN_POINT('Origin',(-7.03243520205041,0.,0.));
#23611=CARTESIAN_POINT('',(0.842564797949603,-3.52020153404575,-0.00255030679734297));
#23612=CARTESIAN_POINT('',(0.990435202050402,-3.5294422032389,-0.000147415198692435));
#23613=CARTESIAN_POINT('',(-7.03243520205041,-3.52375,3.2169090177286E-13));
#23614=CARTESIAN_POINT('Ctrl Pts',(0.842564797949603,-3.52020153404575,
-0.00255030679734352));
#23615=CARTESIAN_POINT('Ctrl Pts',(0.856210381270448,-3.52292703156673,
-0.406286099867594));
#23616=CARTESIAN_POINT('Ctrl Pts',(0.909428701245306,-3.2726899909767,-1.97759684475512));
#23617=CARTESIAN_POINT('Ctrl Pts',(1.00221975787418,-0.961799304980866,
-4.04798401530169));
#23618=CARTESIAN_POINT('Ctrl Pts',(1.12093796783622,2.87028951964572,-3.01208740985575));
#23619=CARTESIAN_POINT('Ctrl Pts',(1.23965617779825,4.0896248253724,0.765637824886821));
#23620=CARTESIAN_POINT('Ctrl Pts',(1.35837438776029,1.586275858193,3.84642189481521));
#23621=CARTESIAN_POINT('Ctrl Pts',(1.47601059447741,-2.32504492362501,3.42973592687219));
#23622=CARTESIAN_POINT('Ctrl Pts',(1.55407406454052,-3.5267219567949,1.13066884340344));
#23623=CARTESIAN_POINT('Ctrl Pts',(1.59256479794961,-3.5293292687682,-0.000582581467793819));
#23624=CARTESIAN_POINT('Ctrl Pts',(0.990435202050402,-3.5294422032389,-0.000147415198692102));
#23625=CARTESIAN_POINT('Ctrl Pts',(0.99070720952674,-3.52944710988525,-0.00814108865577569));
#23626=CARTESIAN_POINT('Ctrl Pts',(1.03055195365709,-3.52581082233263,-1.17908178703684));
#23627=CARTESIAN_POINT('Ctrl Pts',(1.10996943444146,-2.24309286528101,-3.50424991716136));
#23628=CARTESIAN_POINT('Ctrl Pts',(1.22868764440349,1.71622596930723,-3.79022446650269));
#23629=CARTESIAN_POINT('Ctrl Pts',(1.34740585436554,4.11330677534691,-0.626051480379392));
#23630=CARTESIAN_POINT('Ctrl Pts',(1.46612406432757,2.7661462154741,3.10800067548548));
#23631=CARTESIAN_POINT('Ctrl Pts',(1.58484227428961,-1.09896879073751,4.01291672990917));
#23632=CARTESIAN_POINT('Ctrl Pts',(1.67627932019722,-3.30540671418036,1.89644473864501));
#23633=CARTESIAN_POINT('Ctrl Pts',(1.72814362945082,-3.52400110003897,0.366307433305029));
#23634=CARTESIAN_POINT('Ctrl Pts',(1.74043520205041,-3.52117028029313,0.00288554803045071));
#23635=CARTESIAN_POINT('Origin',(-7.03243520205041,0.,0.));
#23636=CARTESIAN_POINT('',(0.0925647979496037,-3.520391836502,0.00262959689127293));
#23637=CARTESIAN_POINT('',(0.240435202050404,-3.52076490314647,-0.00276491524723754));
#23638=CARTESIAN_POINT('',(-7.03243520205041,-3.52375,3.2169090177286E-13));
#23639=CARTESIAN_POINT('Ctrl Pts',(0.0925647979496036,-3.520391836502,0.0026295968912728));
#23640=CARTESIAN_POINT('Ctrl Pts',(0.11877396134637,-3.51497474974621,-0.772722847635471));
#23641=CARTESIAN_POINT('Ctrl Pts',(0.18455586139715,-2.88124574942044,-2.72681485469593));
#23642=CARTESIAN_POINT('Ctrl Pts',(0.289910498101944,0.342796707198351,
-4.1465314310558));
#23643=CARTESIAN_POINT('Ctrl Pts',(0.408628708063982,3.66374931913409,-1.97184518097748));
#23644=CARTESIAN_POINT('Ctrl Pts',(0.52734691802602,3.64968159238416,1.99776294024389));
#23645=CARTESIAN_POINT('Ctrl Pts',(0.64606512798806,0.313399030476065,4.14885689544678));
#23646=CARTESIAN_POINT('Ctrl Pts',(0.751137754629253,-2.89189715861612,
2.71018649449324));
#23647=CARTESIAN_POINT('Ctrl Pts',(0.816637644616435,-3.51502297989571,
0.764563825804819));
#23648=CARTESIAN_POINT('Ctrl Pts',(0.842564797949603,-3.52020153404575,
-0.00255030679734352));
#23649=CARTESIAN_POINT('Ctrl Pts',(0.240435202050404,-3.52076490314647,
-0.00276491524723779));
#23650=CARTESIAN_POINT('Ctrl Pts',(0.253270789602664,-3.52357456820614,
-0.382381961104795));
#23651=CARTESIAN_POINT('Ctrl Pts',(0.305679113808936,-3.29246765048336,
-1.92904800422628));
#23652=CARTESIAN_POINT('Ctrl Pts',(0.397660174669222,-1.04400082814246,
-4.02756692744365));
#23653=CARTESIAN_POINT('Ctrl Pts',(0.516378384631262,2.80838075407454,-3.06989097922772));
#23654=CARTESIAN_POINT('Ctrl Pts',(0.635096594593299,4.10436283463961,0.682230757023696));
#23655=CARTESIAN_POINT('Ctrl Pts',(0.75381480455534,1.66424499718303,3.81333471826842));
#23656=CARTESIAN_POINT('Ctrl Pts',(0.87226100704104,-2.28173208074985,3.47403364657438));
#23657=CARTESIAN_POINT('Ctrl Pts',(0.951134472872727,-3.5287332713303,1.15481052897661));
#23658=CARTESIAN_POINT('Ctrl Pts',(0.990435202050402,-3.5294422032389,-0.000147415198692102));
#23659=CARTESIAN_POINT('Origin',(-7.03243520205041,0.,0.));
#23660=CARTESIAN_POINT('',(-0.657435202050397,-3.5293831919679,0.000432089568584395));
#23661=CARTESIAN_POINT('',(-0.509564797949596,-3.51986320972577,0.00238942109789531));
#23662=CARTESIAN_POINT('',(-7.03243520205041,-3.52375,3.2169090177286E-13));
#23663=CARTESIAN_POINT('Ctrl Pts',(-0.657435202050397,-3.5293831919679,
0.00043208956858453));
#23664=CARTESIAN_POINT('Ctrl Pts',(-0.618662458577708,-3.52740142174523,
-1.13906086225041));
#23665=CARTESIAN_POINT('Ctrl Pts',(-0.540316978451006,-2.31006131649313,
-3.4451963897398));
#23666=CARTESIAN_POINT('Ctrl Pts',(-0.422398761670289,1.61349801702105,
-3.83508235117171));
#23667=CARTESIAN_POINT('Ctrl Pts',(-0.303680551708251,4.09494865907512,
-0.736632860208229));
#23668=CARTESIAN_POINT('Ctrl Pts',(-0.184962341746212,2.84886887415203,
3.0323552940062));
#23669=CARTESIAN_POINT('Ctrl Pts',(-0.0662441317841732,-0.990465746173143,
4.04106546554956));
#23670=CARTESIAN_POINT('Ctrl Pts',(0.0262649147810988,-3.2796457848887,
1.9606934969984));
#23671=CARTESIAN_POINT('Ctrl Pts',(0.0792012246923576,-3.52315391000301,
0.397967633278049));
#23672=CARTESIAN_POINT('Ctrl Pts',(0.0925647979496036,-3.520391836502,0.0026295968912728));
#23673=CARTESIAN_POINT('Ctrl Pts',(-0.509564797949596,-3.51986320972577,
0.00238942109789472));
#23674=CARTESIAN_POINT('Ctrl Pts',(-0.484165630321414,-3.51513982509849,
-0.749284878623226));
#23675=CARTESIAN_POINT('Ctrl Pts',(-0.419193726039219,-2.91159584547546,
-2.67901671514931));
#23676=CARTESIAN_POINT('Ctrl Pts',(-0.31464908510301,0.258318855548078,
-4.15265029265267));
#23677=CARTESIAN_POINT('Ctrl Pts',(-0.195930875140972,3.62285133778538,
-2.04601595020828));
#23678=CARTESIAN_POINT('Ctrl Pts',(-0.0772126651789335,3.68959190165954,
1.92305607911166));
#23679=CARTESIAN_POINT('Ctrl Pts',(0.0415055447831062,0.397788263499511,
4.14161774933685));
#23680=CARTESIAN_POINT('Ctrl Pts',(0.147388167192885,-2.86105940473166,
2.75790715554717));
#23681=CARTESIAN_POINT('Ctrl Pts',(0.213698052948651,-3.51491223506092,
0.787995734807595));
#23682=CARTESIAN_POINT('Ctrl Pts',(0.240435202050404,-3.52076490314647,
-0.00276491524723779));
#23683=CARTESIAN_POINT('Origin',(-7.03243520205041,0.,0.));
#23684=CARTESIAN_POINT('',(-1.4074352020504,-3.52158194415915,-0.00298345148167371));
#23685=CARTESIAN_POINT('',(-1.2595647979496,-3.52918899675462,0.000859749148777282));
#23686=CARTESIAN_POINT('',(-7.03243520205041,-3.52375,3.2169090177286E-13));
#23687=CARTESIAN_POINT('Ctrl Pts',(-1.4074352020504,-3.52158194415915,-0.00298345148167414));
#23688=CARTESIAN_POINT('Ctrl Pts',(-1.3956716151558,-3.5244070910839,-0.350691598451789));
#23689=CARTESIAN_POINT('Ctrl Pts',(-1.34433529160719,-3.31770284706483,
-1.86480632578787));
#23690=CARTESIAN_POINT('Ctrl Pts',(-1.25342623140456,-1.15212076721019,
-3.99798076895909));
#23691=CARTESIAN_POINT('Ctrl Pts',(-1.13470802144252,2.72466151947467,-3.14443191936036));
#23692=CARTESIAN_POINT('Ctrl Pts',(-1.01598981148048,4.12125185197025,0.571415491416797));
#23693=CARTESIAN_POINT('Ctrl Pts',(-0.897271601518446,1.76636861191941,
3.76711752113286));
#23694=CARTESIAN_POINT('Ctrl Pts',(-0.778553391556407,-2.19639626337378,
3.53370569592844));
#23695=CARTESIAN_POINT('Ctrl Pts',(-0.698607925067057,-3.51858688310483,
1.21041940197939));
#23696=CARTESIAN_POINT('Ctrl Pts',(-0.65823519523172,-3.52942408158579,
0.0239431055549515));
#23697=CARTESIAN_POINT('Ctrl Pts',(-0.657435202050397,-3.5293831919679,
0.00043208956858453));
#23698=CARTESIAN_POINT('Ctrl Pts',(-1.2595647979496,-3.52918899675462,0.000859749148777187));
#23699=CARTESIAN_POINT('Ctrl Pts',(-1.22160205024549,-3.5255086737848,-1.11499301985354));
#23700=CARTESIAN_POINT('Ctrl Pts',(-1.14406656588737,-2.3528218011688,-3.40068520645428));
#23701=CARTESIAN_POINT('Ctrl Pts',(-1.02695834487524,1.53509675153174,-3.86713214768211));
#23702=CARTESIAN_POINT('Ctrl Pts',(-0.908240134913205,4.07910533073667,
-0.819837047806264));
#23703=CARTESIAN_POINT('Ctrl Pts',(-0.789521924951166,2.91000527267733,
2.97373542824345));
#23704=CARTESIAN_POINT('Ctrl Pts',(-0.670803714989128,-0.908000571423945,
4.06039013476461));
#23705=CARTESIAN_POINT('Ctrl Pts',(-0.57748467265527,-3.25946475739031,
2.00924411164542));
#23706=CARTESIAN_POINT('Ctrl Pts',(-0.523738366975427,-3.52249901334856,
0.421848346996679));
#23707=CARTESIAN_POINT('Ctrl Pts',(-0.509564797949596,-3.51986320972577,
0.00238942109789472));
#23708=CARTESIAN_POINT('Origin',(-7.03243520205041,0.,0.));
#23709=CARTESIAN_POINT('',(-2.1574352020504,-3.51925399927358,0.00201712429989166));
#23710=CARTESIAN_POINT('',(-2.0095647979496,-3.52224349536472,-0.00309508648049711));
#23711=CARTESIAN_POINT('',(-7.03243520205041,-3.52375,3.2169090177286E-13));
#23712=CARTESIAN_POINT('Ctrl Pts',(-2.1574352020504,-3.51925399927358,0.0020171242998911));
#23713=CARTESIAN_POINT('Ctrl Pts',(-2.13310803507988,-3.51547616379199,
-0.718244932452376));
#23714=CARTESIAN_POINT('Ctrl Pts',(-2.06920813145534,-2.95062385292651,
-2.61558954155717));
#23715=CARTESIAN_POINT('Ctrl Pts',(-1.96573549117679,0.14635662574293,-4.15810199844688));
#23716=CARTESIAN_POINT('Ctrl Pts',(-1.84701728121476,3.56641872576227,-2.14286956292151));
#23717=CARTESIAN_POINT('Ctrl Pts',(-1.72829907125272,3.74005811760244,1.82296400626149));
#23718=CARTESIAN_POINT('Ctrl Pts',(-1.60958086129068,0.509215159922919,
4.12939855331646));
#23719=CARTESIAN_POINT('Ctrl Pts',(-1.50262623822324,-2.81908498068768,
2.82086507657426));
#23720=CARTESIAN_POINT('Ctrl Pts',(-1.43524435180981,-3.51490328954244,
0.818999504762706));
#23721=CARTESIAN_POINT('Ctrl Pts',(-1.4074352020504,-3.52158194415915,-0.00298345148167414));
#23722=CARTESIAN_POINT('Ctrl Pts',(-2.0095647979496,-3.52224349536472,-0.00309508648049749));
#23723=CARTESIAN_POINT('Ctrl Pts',(-1.99861120682358,-3.52501216975828,
-0.326707139459239));
#23724=CARTESIAN_POINT('Ctrl Pts',(-1.94808487904356,-3.33607112434554,
-1.81628010136597));
#23725=CARTESIAN_POINT('Ctrl Pts',(-1.85798581460952,-1.233264991575,-3.97369985590045));
#23726=CARTESIAN_POINT('Ctrl Pts',(-1.73926760464748,2.66008892032246,-3.19924366376966));
#23727=CARTESIAN_POINT('Ctrl Pts',(-1.62054939468544,4.13202971706382,0.487404864048419));
#23728=CARTESIAN_POINT('Ctrl Pts',(-1.5018311847234,1.8426861173841,3.73038080589689));
#23729=CARTESIAN_POINT('Ctrl Pts',(-1.38311297476136,-2.12400905413959,
3.57768341558217));
#23730=CARTESIAN_POINT('Ctrl Pts',(-1.30235751250343,-3.50709119758703,
1.25853137590997));
#23731=CARTESIAN_POINT('Ctrl Pts',(-1.26117478689951,-3.52934507816789,
0.0481827364578268));
#23732=CARTESIAN_POINT('Ctrl Pts',(-1.2595647979496,-3.52918899675462,0.000859749148777187));
#23733=CARTESIAN_POINT('Origin',(-7.03243520205041,0.,0.));
#23734=CARTESIAN_POINT('',(-2.9074352020504,-3.52876079344158,0.00139557051607088));
#23735=CARTESIAN_POINT('',(-2.7595647979496,-3.5188691614322,0.0017004510770105));
#23736=CARTESIAN_POINT('',(-7.03243520205041,-3.52375,3.2169090177286E-13));
#23737=CARTESIAN_POINT('Ctrl Pts',(-2.9074352020504,-3.52876079344158,0.0013955705160707));
#23738=CARTESIAN_POINT('Ctrl Pts',(-2.87054445500395,-3.52327543776816,
-1.08329821888431));
#23739=CARTESIAN_POINT('Ctrl Pts',(-2.7940809713035,-2.40811731696173,-3.34129519327353));
#23740=CARTESIAN_POINT('Ctrl Pts',(-2.67804475094903,1.43036271770746,-3.90708267059147));
#23741=CARTESIAN_POINT('Ctrl Pts',(-2.55932654098699,4.05553922750062,-0.929426740059659));
#23742=CARTESIAN_POINT('Ctrl Pts',(-2.44060833102495,2.9890587402779,2.89426334951592));
#23743=CARTESIAN_POINT('Ctrl Pts',(-2.32189012106291,-0.798287948035305,
4.08337713718073));
#23744=CARTESIAN_POINT('Ctrl Pts',(-2.22749907807139,-3.23179197730365,
2.07349551989286));
#23745=CARTESIAN_POINT('Ctrl Pts',(-2.17268077173389,-3.5216215274842,0.453397483956963));
#23746=CARTESIAN_POINT('Ctrl Pts',(-2.1574352020504,-3.51925399927358,0.0020171242998911));
#23747=CARTESIAN_POINT('Ctrl Pts',(-2.7595647979496,-3.5188691614322,0.00170045107701029));
#23748=CARTESIAN_POINT('Ctrl Pts',(-2.73604762674766,-3.51581077998374,
-0.694770743658778));
#23749=CARTESIAN_POINT('Ctrl Pts',(-2.67295771889171,-2.97926278234442,
-2.56755066425432));
#23750=CARTESIAN_POINT('Ctrl Pts',(-2.57029507438175,0.0616839434797912,
-4.16021972695477));
#23751=CARTESIAN_POINT('Ctrl Pts',(-2.45157686441971,3.52205953641558,-2.21502363553932));
#23752=CARTESIAN_POINT('Ctrl Pts',(-2.33285865445767,3.77639149338881,1.74645365601417));
#23753=CARTESIAN_POINT('Ctrl Pts',(-2.21414044449563,0.593167728051762,
4.11817740399618));
#23754=CARTESIAN_POINT('Ctrl Pts',(-2.10637582565961,-2.78648195150766,
2.86827122209582));
#23755=CARTESIAN_POINT('Ctrl Pts',(-2.0381839434776,-3.5150096033491,0.842426745790324));
#23756=CARTESIAN_POINT('Ctrl Pts',(-2.0095647979496,-3.52224349536472,-0.00309508648049749));
#23757=CARTESIAN_POINT('Origin',(-7.03243520205041,0.,0.));
#23758=CARTESIAN_POINT('',(-3.6574352020504,-3.52316113046627,-0.0031674687847638));
#23759=CARTESIAN_POINT('',(-3.5095647979496,-3.52832659366549,0.00176786622774379));
#23760=CARTESIAN_POINT('',(-7.03243520205041,-3.52375,3.2169090177286E-13));
#23761=CARTESIAN_POINT('Ctrl Pts',(-3.6574352020504,-3.52316113046627,-0.00316746878476385));
#23762=CARTESIAN_POINT('Ctrl Pts',(-3.64755361158204,-3.52577324579835,
-0.294914834651217));
#23763=CARTESIAN_POINT('Ctrl Pts',(-3.59809928445968,-3.35947056833859,
-1.7520841168655));
#23764=CARTESIAN_POINT('Ctrl Pts',(-3.5090722206833,-1.33986509473402,-3.93903455379817));
#23765=CARTESIAN_POINT('Ctrl Pts',(-3.39035401072126,2.57293885887897,-3.26974286547831));
#23766=CARTESIAN_POINT('Ctrl Pts',(-3.27163580075922,4.14366027205377,0.375915015385937));
#23767=CARTESIAN_POINT('Ctrl Pts',(-3.15291759079718,1.94251026639215,3.67938666679367));
#23768=CARTESIAN_POINT('Ctrl Pts',(-3.03419938083515,-2.0268587551866,3.63360373818345));
#23769=CARTESIAN_POINT('Ctrl Pts',(-2.95237191791955,-3.49109730462382,
1.3222721650432));
#23770=CARTESIAN_POINT('Ctrl Pts',(-2.91011719165797,-3.52915958360139,
0.0802537586385255));
#23771=CARTESIAN_POINT('Ctrl Pts',(-2.9074352020504,-3.52876079344158,0.0013955705160707));
#23772=CARTESIAN_POINT('Ctrl Pts',(-3.5095647979496,-3.52832659366549,0.00176786622774375));
#23773=CARTESIAN_POINT('Ctrl Pts',(-3.47348404667174,-3.52178655096766,
-1.05945570162635));
#23774=CARTESIAN_POINT('Ctrl Pts',(-3.39783055873987,-2.44892508739056,
-3.29607736830673));
#23775=CARTESIAN_POINT('Ctrl Pts',(-3.28260433415398,1.35053375419133,-3.93538965177946));
#23776=CARTESIAN_POINT('Ctrl Pts',(-3.16388612419195,4.03577955172485,-1.0117887612591));
#23777=CARTESIAN_POINT('Ctrl Pts',(-3.0451679142299,3.04735509174485,2.83281838700313));
#23778=CARTESIAN_POINT('Ctrl Pts',(-2.92644970426787,-0.715001293115481,
4.09878106793642));
#23779=CARTESIAN_POINT('Ctrl Pts',(-2.83124866550776,-3.21014363212566,
2.122033607616));
#23780=CARTESIAN_POINT('Ctrl Pts',(-2.77562036340167,-3.52095716951368,
0.477192964889438));
#23781=CARTESIAN_POINT('Ctrl Pts',(-2.7595647979496,-3.5188691614322,0.00170045107701029));
#23782=CARTESIAN_POINT('Origin',(-7.03243520205041,0.,0.));
#23783=CARTESIAN_POINT('',(-4.4074352020504,-3.51846707334834,0.00124753304639253));
#23784=CARTESIAN_POINT('',(-4.2595647979496,-3.52387435346743,-0.00316304557197139));
#23785=CARTESIAN_POINT('',(-7.03243520205041,-3.52375,3.2169090177286E-13));
#23786=CARTESIAN_POINT('Ctrl Pts',(-4.4074352020504,-3.51846707334834,0.00124753304639239));
#23787=CARTESIAN_POINT('Ctrl Pts',(-4.38499003150612,-3.51634687456568,
-0.663667541133016));
#23788=CARTESIAN_POINT('Ctrl Pts',(-4.32297212430784,-3.01605608718915,
-2.50384701489226));
#23789=CARTESIAN_POINT('Ctrl Pts',(-4.22138148045554,-0.0504100535793502,
-4.16036696958348));
#23790=CARTESIAN_POINT('Ctrl Pts',(-4.10266327049349,3.46111018837926,-2.30910306912985));
#23791=CARTESIAN_POINT('Ctrl Pts',(-3.98394506053146,3.82206891947539,1.64408864020745));
#23792=CARTESIAN_POINT('Ctrl Pts',(-3.86522685056942,0.703892139470341,
4.1007027146119));
#23793=CARTESIAN_POINT('Ctrl Pts',(-3.75639023107573,-2.7421442575855,2.93077227568166));
#23794=CARTESIAN_POINT('Ctrl Pts',(-3.68712634823606,-3.51531252568681,
0.87344381327186));
#23795=CARTESIAN_POINT('Ctrl Pts',(-3.6574352020504,-3.52316113046627,-0.00316746878476385));
#23796=CARTESIAN_POINT('Ctrl Pts',(-4.2595647979496,-3.52387435346743,-0.0031630455719716));
#23797=CARTESIAN_POINT('Ctrl Pts',(-4.25049320324983,-3.52631361922211,
-0.270857380598162));
#23798=CARTESIAN_POINT('Ctrl Pts',(-4.20184887189605,-3.37647405540411,
-1.70360378513277));
#23799=CARTESIAN_POINT('Ctrl Pts',(-4.11363180388825,-1.41977030063975,
-3.9109435932429));
#23800=CARTESIAN_POINT('Ctrl Pts',(-3.99491359392623,2.50584675349696,-3.32144046072034));
#23801=CARTESIAN_POINT('Ctrl Pts',(-3.87619538396417,4.1504539432636,0.29148889536334));
#23802=CARTESIAN_POINT('Ctrl Pts',(-3.75747717400214,2.01700539684609,3.63908250952178));
#23803=CARTESIAN_POINT('Ctrl Pts',(-3.6387589640401,-1.9524731306016,3.67410969416408));
#23804=CARTESIAN_POINT('Ctrl Pts',(-3.55612150535592,-3.47841478275052,
1.37048332710352));
#23805=CARTESIAN_POINT('Ctrl Pts',(-3.51305678332575,-3.52895955535979,
0.104475738113171));
#23806=CARTESIAN_POINT('Ctrl Pts',(-3.5095647979496,-3.52832659366549,0.00176786622774375));
#23807=CARTESIAN_POINT('Origin',(-7.03243520205041,0.,0.));
#23808=CARTESIAN_POINT('',(-5.1574352020504,-3.52758964538326,0.00244996322663533));
#23809=CARTESIAN_POINT('',(-5.0095647979496,-3.51824182757685,0.00090084872823859));
#23810=CARTESIAN_POINT('',(-7.03243520205041,-3.52375,3.2169090177286E-13));
#23811=CARTESIAN_POINT('Ctrl Pts',(-5.1574352020504,-3.52758964538326,0.0024499632266353));
#23812=CARTESIAN_POINT('Ctrl Pts',(-5.1224264514302,-3.52001727243588,-1.02772586371769));
#23813=CARTESIAN_POINT('Ctrl Pts',(-5.04784496415598,-2.50172051158108,
-3.23619325292719));
#23814=CARTESIAN_POINT('Ctrl Pts',(-4.93369074022778,1.24406479104381,-3.9701278679622));
#23815=CARTESIAN_POINT('Ctrl Pts',(-4.81497253026572,4.0070387833704,-1.12025498671569));
#23816=CARTESIAN_POINT('Ctrl Pts',(-4.69625432030369,3.12257273473017,2.74975698427391));
#23817=CARTESIAN_POINT('Ctrl Pts',(-4.57753611034165,-0.604329863247786,
4.116523575551));
#23818=CARTESIAN_POINT('Ctrl Pts',(-4.48126307092388,-3.18049740052607,
2.18625513612602));
#23819=CARTESIAN_POINT('Ctrl Pts',(-4.42456276816014,-3.52008496458887,
0.508634049353034));
#23820=CARTESIAN_POINT('Ctrl Pts',(-4.4074352020504,-3.51846707334834,0.00124753304639239));
#23821=CARTESIAN_POINT('Ctrl Pts',(-5.0095647979496,-3.51824182757685,0.000900848728238278));
#23822=CARTESIAN_POINT('Ctrl Pts',(-4.98792962317391,-3.51681057818972,
-0.640128378860598));
#23823=CARTESIAN_POINT('Ctrl Pts',(-4.92672171174421,-3.04304236494483,
-2.45565670627494));
#23824=CARTESIAN_POINT('Ctrl Pts',(-4.82594106366048,-0.135078114281208,
-4.15845351012906));
#23825=CARTESIAN_POINT('Ctrl Pts',(-4.70722285369845,3.41338373023632,-2.37909235958642));
#23826=CARTESIAN_POINT('Ctrl Pts',(-4.58850464373641,3.85474686870501,1.56595294230416));
#23827=CARTESIAN_POINT('Ctrl Pts',(-4.46978643377438,0.787218792347394,
4.08552098175258));
#23828=CARTESIAN_POINT('Ctrl Pts',(-4.3601398185121,-2.70773509524305,2.97780255324554));
#23829=CARTESIAN_POINT('Ctrl Pts',(-4.29006593990384,-3.5156728857531,0.896897327847196));
#23830=CARTESIAN_POINT('Ctrl Pts',(-4.2595647979496,-3.52387435346743,-0.0031630455719716));
#23831=CARTESIAN_POINT('Origin',(15.2,0.,0.));
#23832=CARTESIAN_POINT('',(15.4,4.99875513987758,0.111566354908184));
#23833=CARTESIAN_POINT('',(15.4,5.,6.12323399573677E-16));
#23834=CARTESIAN_POINT('Origin',(15.4,0.,0.));
#23835=CARTESIAN_POINT('',(15.,4.6,5.63337527607783E-16));
#23836=CARTESIAN_POINT('',(15.2,4.8,5.87830463590729E-16));
#23837=CARTESIAN_POINT('Origin',(15.,0.,0.));
#23838=CARTESIAN_POINT('',(15.4,4.99875513987758,-0.111566354908184));
#23839=CARTESIAN_POINT('Origin',(15.4,0.,0.));
#23840=CARTESIAN_POINT('',(15.4,4.85730218634588,-1.18600820845369));
#23841=CARTESIAN_POINT('Origin',(15.4,0.,0.));
#23842=CARTESIAN_POINT('',(15.4,4.79955119146007,-1.40153785555518));
#23843=CARTESIAN_POINT('Origin',(15.4,0.,0.));
#23844=CARTESIAN_POINT('',(15.4,4.38483211588611,-2.40275827238067));
#23845=CARTESIAN_POINT('Origin',(15.4,0.,0.));
#23846=CARTESIAN_POINT('',(15.4,4.27326576097792,-2.59599686749691));
#23847=CARTESIAN_POINT('Origin',(15.4,0.,0.));
#23848=CARTESIAN_POINT('',(15.4,3.61354298300638,-3.4557643307907));
#23849=CARTESIAN_POINT('Origin',(15.4,0.,0.));
#23850=CARTESIAN_POINT('',(15.4,3.4557643307907,-3.61354298300639));
#23851=CARTESIAN_POINT('Origin',(15.4,0.,0.));
#23852=CARTESIAN_POINT('',(15.4,2.5959968674969,-4.27326576097793));
#23853=CARTESIAN_POINT('Origin',(15.4,0.,0.));
#23854=CARTESIAN_POINT('',(15.4,2.40275827238067,-4.38483211588611));
#23855=CARTESIAN_POINT('Origin',(15.4,0.,0.));
#23856=CARTESIAN_POINT('',(15.4,1.40153785555518,-4.79955119146007));
#23857=CARTESIAN_POINT('Origin',(15.4,0.,0.));
#23858=CARTESIAN_POINT('',(15.4,1.18600820845368,-4.85730218634588));
#23859=CARTESIAN_POINT('Origin',(15.4,0.,0.));
#23860=CARTESIAN_POINT('',(15.4,0.111566354908183,-4.99875513987758));
#23861=CARTESIAN_POINT('Origin',(15.4,0.,0.));
#23862=CARTESIAN_POINT('',(15.4,-0.111566354908184,-4.99875513987758));
#23863=CARTESIAN_POINT('Origin',(15.4,0.,0.));
#23864=CARTESIAN_POINT('',(15.4,-1.18600820845369,-4.85730218634588));
#23865=CARTESIAN_POINT('Origin',(15.4,0.,0.));
#23866=CARTESIAN_POINT('',(15.4,-1.40153785555518,-4.79955119146007));
#23867=CARTESIAN_POINT('Origin',(15.4,0.,0.));
#23868=CARTESIAN_POINT('',(15.4,-2.40275827238067,-4.38483211588611));
#23869=CARTESIAN_POINT('Origin',(15.4,0.,0.));
#23870=CARTESIAN_POINT('',(15.4,-2.59599686749691,-4.27326576097792));
#23871=CARTESIAN_POINT('Origin',(15.4,0.,0.));
#23872=CARTESIAN_POINT('',(15.4,-3.4557643307907,-3.61354298300638));
#23873=CARTESIAN_POINT('Origin',(15.4,0.,0.));
#23874=CARTESIAN_POINT('',(15.4,-3.61354298300639,-3.4557643307907));
#23875=CARTESIAN_POINT('Origin',(15.4,0.,0.));
#23876=CARTESIAN_POINT('',(15.4,-4.27326576097793,-2.5959968674969));
#23877=CARTESIAN_POINT('Origin',(15.4,0.,0.));
#23878=CARTESIAN_POINT('',(15.4,-4.38483211588611,-2.40275827238067));
#23879=CARTESIAN_POINT('Origin',(15.4,0.,0.));
#23880=CARTESIAN_POINT('',(15.4,-4.79955119146007,-1.40153785555518));
#23881=CARTESIAN_POINT('Origin',(15.4,0.,0.));
#23882=CARTESIAN_POINT('',(15.4,-4.85730218634588,-1.18600820845368));
#23883=CARTESIAN_POINT('Origin',(15.4,0.,0.));
#23884=CARTESIAN_POINT('',(15.4,-4.99875513987758,-0.111566354908183));
#23885=CARTESIAN_POINT('Origin',(15.4,0.,0.));
#23886=CARTESIAN_POINT('',(15.4,-4.99875513987758,0.111566354908184));
#23887=CARTESIAN_POINT('Origin',(15.4,0.,0.));
#23888=CARTESIAN_POINT('',(15.4,-4.85730218634588,1.18600820845369));
#23889=CARTESIAN_POINT('Origin',(15.4,0.,0.));
#23890=CARTESIAN_POINT('',(15.4,-4.79955119146007,1.40153785555518));
#23891=CARTESIAN_POINT('Origin',(15.4,0.,0.));
#23892=CARTESIAN_POINT('',(15.4,-4.38483211588611,2.40275827238067));
#23893=CARTESIAN_POINT('Origin',(15.4,0.,0.));
#23894=CARTESIAN_POINT('',(15.4,-4.27326576097792,2.59599686749691));
#23895=CARTESIAN_POINT('Origin',(15.4,0.,0.));
#23896=CARTESIAN_POINT('',(15.4,-3.61354298300639,3.4557643307907));
#23897=CARTESIAN_POINT('Origin',(15.4,0.,0.));
#23898=CARTESIAN_POINT('',(15.4,-3.4557643307907,3.61354298300639));
#23899=CARTESIAN_POINT('Origin',(15.4,0.,0.));
#23900=CARTESIAN_POINT('',(15.4,-2.5959968674969,4.27326576097793));
#23901=CARTESIAN_POINT('Origin',(15.4,0.,0.));
#23902=CARTESIAN_POINT('',(15.4,-2.40275827238067,4.38483211588611));
#23903=CARTESIAN_POINT('Origin',(15.4,0.,0.));
#23904=CARTESIAN_POINT('',(15.4,-1.40153785555518,4.79955119146007));
#23905=CARTESIAN_POINT('Origin',(15.4,0.,0.));
#23906=CARTESIAN_POINT('',(15.4,-1.18600820845369,4.85730218634588));
#23907=CARTESIAN_POINT('Origin',(15.4,0.,0.));
#23908=CARTESIAN_POINT('',(15.4,-0.111566354908183,4.99875513987758));
#23909=CARTESIAN_POINT('Origin',(15.4,0.,0.));
#23910=CARTESIAN_POINT('',(15.4,0.111566354908184,4.99875513987758));
#23911=CARTESIAN_POINT('Origin',(15.4,0.,0.));
#23912=CARTESIAN_POINT('',(15.4,1.18600820845369,4.85730218634588));
#23913=CARTESIAN_POINT('Origin',(15.4,0.,0.));
#23914=CARTESIAN_POINT('',(15.4,1.40153785555518,4.79955119146007));
#23915=CARTESIAN_POINT('Origin',(15.4,0.,0.));
#23916=CARTESIAN_POINT('',(15.4,2.40275827238067,4.38483211588611));
#23917=CARTESIAN_POINT('Origin',(15.4,0.,0.));
#23918=CARTESIAN_POINT('',(15.4,2.59599686749691,4.27326576097793));
#23919=CARTESIAN_POINT('Origin',(15.4,0.,0.));
#23920=CARTESIAN_POINT('',(15.4,3.4557643307907,3.61354298300638));
#23921=CARTESIAN_POINT('Origin',(15.4,0.,0.));
#23922=CARTESIAN_POINT('',(15.4,3.61354298300639,3.4557643307907));
#23923=CARTESIAN_POINT('Origin',(15.4,0.,0.));
#23924=CARTESIAN_POINT('',(15.4,4.27326576097793,2.59599686749691));
#23925=CARTESIAN_POINT('Origin',(15.4,0.,0.));
#23926=CARTESIAN_POINT('',(15.4,4.38483211588611,2.40275827238067));
#23927=CARTESIAN_POINT('Origin',(15.4,0.,0.));
#23928=CARTESIAN_POINT('',(15.4,4.79955119146007,1.40153785555518));
#23929=CARTESIAN_POINT('Origin',(15.4,0.,0.));
#23930=CARTESIAN_POINT('',(15.4,4.85730218634588,1.18600820845369));
#23931=CARTESIAN_POINT('Origin',(15.4,0.,0.));
#23932=CARTESIAN_POINT('Origin',(15.4,0.,0.));
#23933=CARTESIAN_POINT('Origin',(17.75,0.,0.));
#23934=CARTESIAN_POINT('',(20.5,-5.,-6.12323399573677E-16));
#23935=CARTESIAN_POINT('Origin',(20.5,0.,0.));
#23936=CARTESIAN_POINT('',(20.4,-5.,-6.12323399573677E-16));
#23937=CARTESIAN_POINT('',(17.75,-5.,-6.12323399573677E-16));
#23938=CARTESIAN_POINT('',(20.4,-4.99875513987758,-0.111566354908183));
#23939=CARTESIAN_POINT('Origin',(20.4,0.,0.));
#23940=CARTESIAN_POINT('',(17.75,-4.99875513987758,-0.111566354908183));
#23941=CARTESIAN_POINT('',(20.4,-4.85730218634588,-1.18600820845368));
#23942=CARTESIAN_POINT('',(17.75,-4.85730218634588,-1.18600820845368));
#23943=CARTESIAN_POINT('',(20.4,-4.79955119146007,-1.40153785555518));
#23944=CARTESIAN_POINT('Origin',(20.4,0.,0.));
#23945=CARTESIAN_POINT('',(17.75,-4.79955119146007,-1.40153785555518));
#23946=CARTESIAN_POINT('',(20.4,-4.38483211588611,-2.40275827238067));
#23947=CARTESIAN_POINT('',(17.75,-4.38483211588611,-2.40275827238067));
#23948=CARTESIAN_POINT('',(20.4,-4.27326576097793,-2.5959968674969));
#23949=CARTESIAN_POINT('Origin',(20.4,0.,0.));
#23950=CARTESIAN_POINT('',(17.75,-4.27326576097793,-2.5959968674969));
#23951=CARTESIAN_POINT('',(20.4,-3.61354298300639,-3.4557643307907));
#23952=CARTESIAN_POINT('',(17.75,-3.61354298300639,-3.4557643307907));
#23953=CARTESIAN_POINT('',(20.4,-3.4557643307907,-3.61354298300638));
#23954=CARTESIAN_POINT('Origin',(20.4,0.,0.));
#23955=CARTESIAN_POINT('',(17.75,-3.4557643307907,-3.61354298300638));
#23956=CARTESIAN_POINT('',(20.4,-2.59599686749691,-4.27326576097792));
#23957=CARTESIAN_POINT('',(17.75,-2.59599686749691,-4.27326576097792));
#23958=CARTESIAN_POINT('',(20.4,-2.40275827238067,-4.38483211588611));
#23959=CARTESIAN_POINT('Origin',(20.4,0.,0.));
#23960=CARTESIAN_POINT('',(17.75,-2.40275827238067,-4.38483211588611));
#23961=CARTESIAN_POINT('',(20.4,-1.40153785555518,-4.79955119146007));
#23962=CARTESIAN_POINT('',(17.75,-1.40153785555518,-4.79955119146007));
#23963=CARTESIAN_POINT('',(20.4,-1.18600820845369,-4.85730218634588));
#23964=CARTESIAN_POINT('Origin',(20.4,0.,0.));
#23965=CARTESIAN_POINT('',(17.75,-1.18600820845369,-4.85730218634588));
#23966=CARTESIAN_POINT('',(20.4,-0.111566354908184,-4.99875513987758));
#23967=CARTESIAN_POINT('',(17.75,-0.111566354908184,-4.99875513987758));
#23968=CARTESIAN_POINT('',(20.4,0.111566354908183,-4.99875513987758));
#23969=CARTESIAN_POINT('Origin',(20.4,0.,0.));
#23970=CARTESIAN_POINT('',(17.75,0.111566354908183,-4.99875513987758));
#23971=CARTESIAN_POINT('',(20.4,1.18600820845368,-4.85730218634588));
#23972=CARTESIAN_POINT('',(17.75,1.18600820845368,-4.85730218634588));
#23973=CARTESIAN_POINT('',(20.4,1.40153785555518,-4.79955119146007));
#23974=CARTESIAN_POINT('Origin',(20.4,0.,0.));
#23975=CARTESIAN_POINT('',(17.75,1.40153785555518,-4.79955119146007));
#23976=CARTESIAN_POINT('',(20.4,2.40275827238067,-4.38483211588611));
#23977=CARTESIAN_POINT('',(17.75,2.40275827238067,-4.38483211588611));
#23978=CARTESIAN_POINT('',(20.4,2.5959968674969,-4.27326576097793));
#23979=CARTESIAN_POINT('Origin',(20.4,0.,0.));
#23980=CARTESIAN_POINT('',(17.75,2.5959968674969,-4.27326576097793));
#23981=CARTESIAN_POINT('',(20.4,3.4557643307907,-3.61354298300639));
#23982=CARTESIAN_POINT('',(17.75,3.4557643307907,-3.61354298300639));
#23983=CARTESIAN_POINT('',(20.4,3.61354298300638,-3.4557643307907));
#23984=CARTESIAN_POINT('Origin',(20.4,0.,0.));
#23985=CARTESIAN_POINT('',(17.75,3.61354298300638,-3.4557643307907));
#23986=CARTESIAN_POINT('',(20.4,4.27326576097792,-2.59599686749691));
#23987=CARTESIAN_POINT('',(17.75,4.27326576097792,-2.59599686749691));
#23988=CARTESIAN_POINT('',(20.4,4.38483211588611,-2.40275827238067));
#23989=CARTESIAN_POINT('Origin',(20.4,0.,0.));
#23990=CARTESIAN_POINT('',(17.75,4.38483211588611,-2.40275827238067));
#23991=CARTESIAN_POINT('',(20.4,4.79955119146007,-1.40153785555518));
#23992=CARTESIAN_POINT('',(17.75,4.79955119146007,-1.40153785555518));
#23993=CARTESIAN_POINT('',(20.4,4.85730218634588,-1.18600820845369));
#23994=CARTESIAN_POINT('Origin',(20.4,0.,0.));
#23995=CARTESIAN_POINT('',(17.75,4.85730218634588,-1.18600820845369));
#23996=CARTESIAN_POINT('',(20.4,4.99875513987758,-0.111566354908184));
#23997=CARTESIAN_POINT('',(17.75,4.99875513987758,-0.111566354908184));
#23998=CARTESIAN_POINT('',(20.4,4.99875513987758,0.111566354908184));
#23999=CARTESIAN_POINT('Origin',(20.4,0.,0.));
#24000=CARTESIAN_POINT('',(17.75,4.99875513987758,0.111566354908184));
#24001=CARTESIAN_POINT('',(20.4,4.85730218634588,1.18600820845369));
#24002=CARTESIAN_POINT('',(17.75,4.85730218634588,1.18600820845369));
#24003=CARTESIAN_POINT('',(20.4,4.79955119146007,1.40153785555518));
#24004=CARTESIAN_POINT('Origin',(20.4,0.,0.));
#24005=CARTESIAN_POINT('',(17.75,4.79955119146007,1.40153785555518));
#24006=CARTESIAN_POINT('',(20.4,4.38483211588611,2.40275827238067));
#24007=CARTESIAN_POINT('',(17.75,4.38483211588611,2.40275827238067));
#24008=CARTESIAN_POINT('',(20.4,4.27326576097793,2.59599686749691));
#24009=CARTESIAN_POINT('Origin',(20.4,0.,0.));
#24010=CARTESIAN_POINT('',(17.75,4.27326576097793,2.59599686749691));
#24011=CARTESIAN_POINT('',(20.4,3.61354298300639,3.4557643307907));
#24012=CARTESIAN_POINT('',(17.75,3.61354298300639,3.4557643307907));
#24013=CARTESIAN_POINT('',(20.4,3.4557643307907,3.61354298300638));
#24014=CARTESIAN_POINT('Origin',(20.4,0.,0.));
#24015=CARTESIAN_POINT('',(17.75,3.4557643307907,3.61354298300638));
#24016=CARTESIAN_POINT('',(20.4,2.59599686749691,4.27326576097793));
#24017=CARTESIAN_POINT('',(17.75,2.59599686749691,4.27326576097793));
#24018=CARTESIAN_POINT('',(20.4,2.40275827238067,4.38483211588611));
#24019=CARTESIAN_POINT('Origin',(20.4,0.,0.));
#24020=CARTESIAN_POINT('',(17.75,2.40275827238067,4.38483211588611));
#24021=CARTESIAN_POINT('',(20.4,1.40153785555518,4.79955119146007));
#24022=CARTESIAN_POINT('',(17.75,1.40153785555518,4.79955119146007));
#24023=CARTESIAN_POINT('',(20.4,1.18600820845369,4.85730218634588));
#24024=CARTESIAN_POINT('Origin',(20.4,0.,0.));
#24025=CARTESIAN_POINT('',(17.75,1.18600820845369,4.85730218634588));
#24026=CARTESIAN_POINT('',(20.4,0.111566354908184,4.99875513987758));
#24027=CARTESIAN_POINT('',(17.75,0.111566354908184,4.99875513987758));
#24028=CARTESIAN_POINT('',(20.4,-0.111566354908183,4.99875513987758));
#24029=CARTESIAN_POINT('Origin',(20.4,0.,0.));
#24030=CARTESIAN_POINT('',(17.75,-0.111566354908183,4.99875513987758));
#24031=CARTESIAN_POINT('',(20.4,-1.18600820845369,4.85730218634588));
#24032=CARTESIAN_POINT('',(17.75,-1.18600820845369,4.85730218634588));
#24033=CARTESIAN_POINT('',(20.4,-1.40153785555518,4.79955119146007));
#24034=CARTESIAN_POINT('Origin',(20.4,0.,0.));
#24035=CARTESIAN_POINT('',(17.75,-1.40153785555518,4.79955119146007));
#24036=CARTESIAN_POINT('',(20.4,-2.40275827238067,4.38483211588611));
#24037=CARTESIAN_POINT('',(17.75,-2.40275827238067,4.38483211588611));
#24038=CARTESIAN_POINT('',(20.4,-2.5959968674969,4.27326576097793));
#24039=CARTESIAN_POINT('Origin',(20.4,0.,0.));
#24040=CARTESIAN_POINT('',(17.75,-2.5959968674969,4.27326576097793));
#24041=CARTESIAN_POINT('',(20.4,-3.4557643307907,3.61354298300639));
#24042=CARTESIAN_POINT('',(17.75,-3.4557643307907,3.61354298300639));
#24043=CARTESIAN_POINT('',(20.4,-3.61354298300639,3.4557643307907));
#24044=CARTESIAN_POINT('Origin',(20.4,0.,0.));
#24045=CARTESIAN_POINT('',(17.75,-3.61354298300639,3.4557643307907));
#24046=CARTESIAN_POINT('',(20.4,-4.27326576097792,2.59599686749691));
#24047=CARTESIAN_POINT('',(17.75,-4.27326576097792,2.59599686749691));
#24048=CARTESIAN_POINT('',(20.4,-4.38483211588611,2.40275827238067));
#24049=CARTESIAN_POINT('Origin',(20.4,0.,0.));
#24050=CARTESIAN_POINT('',(17.75,-4.38483211588611,2.40275827238067));
#24051=CARTESIAN_POINT('',(20.4,-4.79955119146007,1.40153785555518));
#24052=CARTESIAN_POINT('',(17.75,-4.79955119146007,1.40153785555518));
#24053=CARTESIAN_POINT('',(20.4,-4.85730218634588,1.18600820845369));
#24054=CARTESIAN_POINT('Origin',(20.4,0.,0.));
#24055=CARTESIAN_POINT('',(17.75,-4.85730218634588,1.18600820845369));
#24056=CARTESIAN_POINT('',(20.4,-4.99875513987758,0.111566354908184));
#24057=CARTESIAN_POINT('',(17.75,-4.99875513987758,0.111566354908184));
#24058=CARTESIAN_POINT('Origin',(20.4,0.,0.));
#24059=CARTESIAN_POINT('Origin',(15.,5.,0.));
#24060=CARTESIAN_POINT('',(15.,-1.03647793659398,-3.81573446232228));
#24061=CARTESIAN_POINT('',(15.,2.28804281094429,-3.22474434572513));
#24062=CARTESIAN_POINT('Origin',(15.,0.,0.));
#24063=CARTESIAN_POINT('Ctrl Pts',(15.,2.29296287427331,-3.22854765929654));
#24064=CARTESIAN_POINT('Ctrl Pts',(15.,2.38802987998202,-3.15422468240186));
#24065=CARTESIAN_POINT('Ctrl Pts',(15.,2.47929003976274,-3.07546894025832));
#24066=CARTESIAN_POINT('Ctrl Pts',(15.,2.56634326510049,-2.99233335005528));
#24067=CARTESIAN_POINT('Ctrl Pts',(15.,2.65493259497213,-2.90773078425721));
#24068=CARTESIAN_POINT('Ctrl Pts',(15.,2.73916570047965,-2.81859185262434));
#24069=CARTESIAN_POINT('Ctrl Pts',(15.,2.81893234754107,-2.72535231130569));
#24070=CARTESIAN_POINT('Ctrl Pts',(15.,2.8655488015903,-2.67086215842129));
#24071=CARTESIAN_POINT('Ctrl Pts',(15.,2.9106390081652,-2.6149708782813));
#24072=CARTESIAN_POINT('Ctrl Pts',(15.,2.95417392507206,-2.55776142184591));
#24073=CARTESIAN_POINT('Ctrl Pts',(15.,2.97044986150209,-2.53637313073853));
#24074=CARTESIAN_POINT('Ctrl Pts',(15.,2.98650835998393,-2.51480057368804));
#24075=CARTESIAN_POINT('Ctrl Pts',(15.,3.00234770735048,-2.49304801108135));
#24076=CARTESIAN_POINT('Ctrl Pts',(15.,3.01345384358298,-2.47779568293138));
#24077=CARTESIAN_POINT('Ctrl Pts',(15.,3.0244501860737,-2.46245759943643));
#24078=CARTESIAN_POINT('Ctrl Pts',(15.,3.03533167348133,-2.44704197570961));
#24079=CARTESIAN_POINT('Ctrl Pts',(15.,3.10579918825424,-2.34721180984998));
#24080=CARTESIAN_POINT('Ctrl Pts',(15.,3.1715131122476,-2.24405067996107));
#24081=CARTESIAN_POINT('Ctrl Pts',(15.,3.23237311287027,-2.13799352531919));
#24082=CARTESIAN_POINT('Ctrl Pts',(15.,3.28913549272338,-2.039077054134));
#24083=CARTESIAN_POINT('Ctrl Pts',(15.,3.34167530236964,-1.93764052209836));
#24084=CARTESIAN_POINT('Ctrl Pts',(15.,3.38987488751025,-1.83402043431015));
#24085=CARTESIAN_POINT('Ctrl Pts',(15.,3.41096220600926,-1.7886866459028));
#24086=CARTESIAN_POINT('Ctrl Pts',(15.,3.43121831216432,-1.74293476505114));
#24087=CARTESIAN_POINT('Ctrl Pts',(15.,3.45063112290763,-1.69679248888462));
#24088=CARTESIAN_POINT('Ctrl Pts',(15.,3.46151559578505,-1.67092120419135));
#24089=CARTESIAN_POINT('Ctrl Pts',(15.,3.47213493890906,-1.64492718836514));
#24090=CARTESIAN_POINT('Ctrl Pts',(15.,3.48248682880138,-1.61881530800709));
#24091=CARTESIAN_POINT('Ctrl Pts',(15.,3.49167793747036,-1.59563141285185));
#24092=CARTESIAN_POINT('Ctrl Pts',(15.,3.50065985969643,-1.57234993370711));
#24093=CARTESIAN_POINT('Ctrl Pts',(15.,3.50942051936889,-1.54900268324877));
#24094=CARTESIAN_POINT('Ctrl Pts',(15.,3.55239670909123,-1.43447068420923));
#24095=CARTESIAN_POINT('Ctrl Pts',(15.,3.590099835495,-1.31824322012931));
#24096=CARTESIAN_POINT('Ctrl Pts',(15.,3.62242629257587,-1.20074292158529));
#24097=CARTESIAN_POINT('Ctrl Pts',(15.,3.65467682719235,-1.08351858623173));
#24098=CARTESIAN_POINT('Ctrl Pts',(15.,3.68157610969259,-0.965026499777471));
#24099=CARTESIAN_POINT('Ctrl Pts',(15.,3.70297113528148,-0.845674315408051));
#24100=CARTESIAN_POINT('Ctrl Pts',(15.,3.72380182912614,-0.729470256573858));
#24101=CARTESIAN_POINT('Ctrl Pts',(15.,3.73941478911051,-0.612450092321461));
#24102=CARTESIAN_POINT('Ctrl Pts',(15.,3.74962026873843,-0.494990953545431));
#24103=CARTESIAN_POINT('Ctrl Pts',(15.,3.75681704041738,-0.412160294507659));
#24104=CARTESIAN_POINT('Ctrl Pts',(15.,3.76132374153974,-0.329111341532594));
#24105=CARTESIAN_POINT('Ctrl Pts',(15.,3.76305869017149,-0.245979715350486));
#24106=CARTESIAN_POINT('Ctrl Pts',(15.,3.76368445161509,-0.215995792220352));
#24107=CARTESIAN_POINT('Ctrl Pts',(15.,3.76394951400646,-0.186001152326826));
#24108=CARTESIAN_POINT('Ctrl Pts',(15.,3.76384962862183,-0.156002306664786));
#24109=CARTESIAN_POINT('Ctrl Pts',(15.,3.76378992941917,-0.138072684895765));
#24110=CARTESIAN_POINT('Ctrl Pts',(15.,3.76359976828237,-0.120140261775781));
#24111=CARTESIAN_POINT('Ctrl Pts',(15.,3.76327872654335,-0.102224379574802));
#24112=CARTESIAN_POINT('Ctrl Pts',(15.,3.7611762610886,0.0151046740680469));
#24113=CARTESIAN_POINT('Ctrl Pts',(15.,3.75346533085488,0.131899636400721));
#24114=CARTESIAN_POINT('Ctrl Pts',(15.,3.74000614617998,0.247789192086024));
#24115=CARTESIAN_POINT('Ctrl Pts',(15.,3.7303579680308,0.330864289567014));
#24116=CARTESIAN_POINT('Ctrl Pts',(15.,3.71775491296525,0.413474227796892));
#24117=CARTESIAN_POINT('Ctrl Pts',(15.,3.70212909055716,0.49547992626668));
#24118=CARTESIAN_POINT('Ctrl Pts',(15.,3.68014511871305,0.610853755504814));
#24119=CARTESIAN_POINT('Ctrl Pts',(15.,3.65217973575864,0.725032707578649));
#24120=CARTESIAN_POINT('Ctrl Pts',(15.,3.61851345531731,0.837703056235049));
#24121=CARTESIAN_POINT('Ctrl Pts',(15.,3.58455108518543,0.951364323051458));
#24122=CARTESIAN_POINT('Ctrl Pts',(15.,3.54478656262233,1.06349105917797));
#24123=CARTESIAN_POINT('Ctrl Pts',(15.,3.4994629109816,1.17373379051609));
#24124=CARTESIAN_POINT('Ctrl Pts',(15.,3.48735010956251,1.20319629550534));
#24125=CARTESIAN_POINT('Ctrl Pts',(15.,3.47484003581574,1.23252405453656));
#24126=CARTESIAN_POINT('Ctrl Pts',(15.,3.46193686781402,1.26170996577144));
#24127=CARTESIAN_POINT('Ctrl Pts',(15.,3.45526116077079,1.27680986938952));
#24128=CARTESIAN_POINT('Ctrl Pts',(15.,3.4484840071925,1.29186323438959));
#24129=CARTESIAN_POINT('Ctrl Pts',(15.,3.44160728857144,1.306867154827));
#24130=CARTESIAN_POINT('Ctrl Pts',(15.,3.39287914176642,1.41318432119845));
#24131=CARTESIAN_POINT('Ctrl Pts',(15.,3.3391404716466,1.51705536326108));
#24132=CARTESIAN_POINT('Ctrl Pts',(15.,3.2806979050605,1.61818973367994));
#24133=CARTESIAN_POINT('Ctrl Pts',(15.,3.22190782882257,1.7199254666314));
#24134=CARTESIAN_POINT('Ctrl Pts',(15.,3.15835716382197,1.81889257743335));
#24135=CARTESIAN_POINT('Ctrl Pts',(15.,3.09031245415742,1.91476797192053));
#24136=CARTESIAN_POINT('Ctrl Pts',(15.,3.02278563717085,2.0099136525909));
#24137=CARTESIAN_POINT('Ctrl Pts',(15.,2.95083228311762,2.10201510480185));
#24138=CARTESIAN_POINT('Ctrl Pts',(15.,2.87467744809909,2.19072013381056));
#24139=CARTESIAN_POINT('Ctrl Pts',(15.,2.82842890210364,2.24459036559741));
#24140=CARTESIAN_POINT('Ctrl Pts',(15.,2.78063016774874,2.29720722102989));
#24141=CARTESIAN_POINT('Ctrl Pts',(15.,2.73132668700375,2.34848374369048));
#24142=CARTESIAN_POINT('Ctrl Pts',(15.,2.71416029468208,2.36633710600045));
#24143=CARTESIAN_POINT('Ctrl Pts',(15.,2.69681145622203,2.384027923152));
#24144=CARTESIAN_POINT('Ctrl Pts',(15.,2.67928200313545,2.40155232826184));
#24145=CARTESIAN_POINT('Ctrl Pts',(15.,2.66457020727519,2.41625988754935));
#24146=CARTESIAN_POINT('Ctrl Pts',(15.,2.64972855828448,2.43085265888608));
#24147=CARTESIAN_POINT('Ctrl Pts',(15.,2.63477716327216,2.44531024066103));
#24148=CARTESIAN_POINT('Ctrl Pts',(15.,2.55170266149999,2.52564096577364));
#24149=CARTESIAN_POINT('Ctrl Pts',(15.,2.46513368308695,2.60191292355531));
#24150=CARTESIAN_POINT('Ctrl Pts',(15.,2.37532241430713,2.67382459269717));
#24151=CARTESIAN_POINT('Ctrl Pts',(15.,2.28654836265619,2.74490576455274));
#24152=CARTESIAN_POINT('Ctrl Pts',(15.,2.19460584593852,2.81172729121945));
#24153=CARTESIAN_POINT('Ctrl Pts',(15.,2.09970897870241,2.87395745757045));
#24154=CARTESIAN_POINT('Ctrl Pts',(15.,2.00713664782224,2.93466327134448));
#24155=CARTESIAN_POINT('Ctrl Pts',(15.,1.91175234806588,2.9910002513087));
#24156=CARTESIAN_POINT('Ctrl Pts',(15.,1.81373561196281,3.04261555880697));
#24157=CARTESIAN_POINT('Ctrl Pts',(15.,1.71571887585974,3.09423086630524));
#24158=CARTESIAN_POINT('Ctrl Pts',(15.,1.61506922876594,3.14112502559283));
#24159=CARTESIAN_POINT('Ctrl Pts',(15.,1.51195443948848,3.18289299779479));
#24160=CARTESIAN_POINT('Ctrl Pts',(15.,-2.52120044613813,2.46936361140965));
#24161=CARTESIAN_POINT('Ctrl Pts',(15.,-2.60179898682872,2.39717859433151));
#24162=CARTESIAN_POINT('Ctrl Pts',(15.,-2.67869877568603,2.3212580895175));
#24163=CARTESIAN_POINT('Ctrl Pts',(15.,-2.75155631737188,2.24172753651207));
#24164=CARTESIAN_POINT('Ctrl Pts',(15.,-2.82661178723241,2.15979774741999));
#24165=CARTESIAN_POINT('Ctrl Pts',(15.,-2.8973785762359,2.07403697418862));
#24166=CARTESIAN_POINT('Ctrl Pts',(15.,-2.96383857017409,1.98486101330688));
#24167=CARTESIAN_POINT('Ctrl Pts',(15.,-3.00474733706439,1.92996966620079));
#24168=CARTESIAN_POINT('Ctrl Pts',(15.,-3.04402362867714,1.87378350573605));
#24169=CARTESIAN_POINT('Ctrl Pts',(15.,-3.08165627846039,1.81639284598983));
#24170=CARTESIAN_POINT('Ctrl Pts',(15.,-3.09368658503351,1.79804635072156));
#24171=CARTESIAN_POINT('Ctrl Pts',(15.,-3.10554887976004,1.77957672978204));
#24172=CARTESIAN_POINT('Ctrl Pts',(15.,-3.11724267731674,1.76098684436662));
#24173=CARTESIAN_POINT('Ctrl Pts',(15.,-3.12837591079725,1.74328809990809));
#24174=CARTESIAN_POINT('Ctrl Pts',(15.,-3.1393524148385,1.72548662453293));
#24175=CARTESIAN_POINT('Ctrl Pts',(15.,-3.15016852685405,1.70759114823924));
#24176=CARTESIAN_POINT('Ctrl Pts',(15.,-3.20879801673494,1.61058747032193));
#24177=CARTESIAN_POINT('Ctrl Pts',(15.,-3.2627518772499,1.51077072777429));
#24178=CARTESIAN_POINT('Ctrl Pts',(15.,-3.31201510422133,1.40857225843896));
#24179=CARTESIAN_POINT('Ctrl Pts',(15.,-3.35951680124557,1.31002815109649));
#24180=CARTESIAN_POINT('Ctrl Pts',(15.,-3.40265730316664,1.20926876756575));
#24181=CARTESIAN_POINT('Ctrl Pts',(15.,-3.44138896342653,1.10665322186668));
#24182=CARTESIAN_POINT('Ctrl Pts',(15.,-3.45833406479024,1.06175892062334));
#24183=CARTESIAN_POINT('Ctrl Pts',(15.,-3.47443483618565,1.01650904659998));
#24184=CARTESIAN_POINT('Ctrl Pts',(15.,-3.48968512212765,0.970932519453672));
#24185=CARTESIAN_POINT('Ctrl Pts',(15.,-3.4983119898275,0.945150532715522));
#24186=CARTESIAN_POINT('Ctrl Pts',(15.,-3.50666667748744,0.91926400607298));
#24187=CARTESIAN_POINT('Ctrl Pts',(15.,-3.51474787552058,0.893278102137526));
#24188=CARTESIAN_POINT('Ctrl Pts',(15.,-3.52046912920241,0.874880836291959));
#24189=CARTESIAN_POINT('Ctrl Pts',(15.,-3.52605061516273,0.856442309316086));
#24190=CARTESIAN_POINT('Ctrl Pts',(15.,-3.53149085344976,0.837969346152265));
#24191=CARTESIAN_POINT('Ctrl Pts',(15.,-3.56477303826427,0.724955808573256));
#24192=CARTESIAN_POINT('Ctrl Pts',(15.,-3.59279001212681,0.610598793555419));
#24193=CARTESIAN_POINT('Ctrl Pts',(15.,-3.61551923482663,0.495347390597081));
#24194=CARTESIAN_POINT('Ctrl Pts',(15.,-3.63850038450621,0.378818559974632));
#24195=CARTESIAN_POINT('Ctrl Pts',(15.,-3.65607624651716,0.261374564334388));
#24196=CARTESIAN_POINT('Ctrl Pts',(15.,-3.66817706892989,0.14345385470107));
#24197=CARTESIAN_POINT('Ctrl Pts',(15.,-3.68015016445688,0.0267778245194678));
#24198=CARTESIAN_POINT('Ctrl Pts',(15.,-3.68676336140009,-0.0903658031962653));
#24199=CARTESIAN_POINT('Ctrl Pts',(15.,-3.68790038379689,-0.207564280302668));
#24200=CARTESIAN_POINT('Ctrl Pts',(15.,-3.68867220478621,-0.287119656521374));
#24201=CARTESIAN_POINT('Ctrl Pts',(15.,-3.68691970242156,-0.366700546990979));
#24202=CARTESIAN_POINT('Ctrl Pts',(15.,-3.68259285188237,-0.446177887149181));
#24203=CARTESIAN_POINT('Ctrl Pts',(15.,-3.68144217396426,-0.467314004396978));
#24204=CARTESIAN_POINT('Ctrl Pts',(15.,-3.68010936634767,-0.488442791064557));
#24205=CARTESIAN_POINT('Ctrl Pts',(15.,-3.67859335009362,-0.509561799177698));
#24206=CARTESIAN_POINT('Ctrl Pts',(15.,-3.67741985285778,-0.525909313644376));
#24207=CARTESIAN_POINT('Ctrl Pts',(15.,-3.67613653785577,-0.542250677006092));
#24208=CARTESIAN_POINT('Ctrl Pts',(15.,-3.67474426482348,-0.558570866196314));
#24209=CARTESIAN_POINT('Ctrl Pts',(15.,-3.66454291715474,-0.67815080496419));
#24210=CARTESIAN_POINT('Ctrl Pts',(15.,-3.64848322229041,-0.796782907711174));
#24211=CARTESIAN_POINT('Ctrl Pts',(15.,-3.62650052051321,-0.914027217005267));
#24212=CARTESIAN_POINT('Ctrl Pts',(15.,-3.61163636836508,-0.993304881302997));
#24213=CARTESIAN_POINT('Ctrl Pts',(15.,-3.59406313593742,-1.07194840668789));
#24214=CARTESIAN_POINT('Ctrl Pts',(15.,-3.57374739672799,-1.14982341224806));
#24215=CARTESIAN_POINT('Ctrl Pts',(15.,-3.54447892467199,-1.26201634801092));
#24216=CARTESIAN_POINT('Ctrl Pts',(15.,-3.50952067095247,-1.37261494887389));
#24217=CARTESIAN_POINT('Ctrl Pts',(15.,-3.46919598978005,-1.48138234197029));
#24218=CARTESIAN_POINT('Ctrl Pts',(15.,-3.42815857585037,-1.59207218260321));
#24219=CARTESIAN_POINT('Ctrl Pts',(15.,-3.38156301779153,-1.70086616239473));
#24220=CARTESIAN_POINT('Ctrl Pts',(15.,-3.32969852456671,-1.80749900795472));
#24221=CARTESIAN_POINT('Ctrl Pts',(15.,-3.31675311277751,-1.8341146366864));
#24222=CARTESIAN_POINT('Ctrl Pts',(15.,-3.30347921086797,-1.86059552333069));
#24223=CARTESIAN_POINT('Ctrl Pts',(15.,-3.28988086646955,-1.8869373191648));
#24224=CARTESIAN_POINT('Ctrl Pts',(15.,-3.28041699897394,-1.90527008513));
#24225=CARTESIAN_POINT('Ctrl Pts',(15.,-3.27079458652134,-1.92353788999526));
#24226=CARTESIAN_POINT('Ctrl Pts',(15.,-3.26102676821148,-1.94171779428929));
#24227=CARTESIAN_POINT('Ctrl Pts',(15.,-3.2023945117954,-2.05084439517136));
#24228=CARTESIAN_POINT('Ctrl Pts',(15.,-3.13844653177481,-2.15696706986354));
#24229=CARTESIAN_POINT('Ctrl Pts',(15.,-3.06959759380989,-2.25981885873531));
#24230=CARTESIAN_POINT('Ctrl Pts',(15.,-3.00218015142085,-2.36053217045558));
#24231=CARTESIAN_POINT('Ctrl Pts',(15.,-2.93006266448803,-2.45810980071153));
#24232=CARTESIAN_POINT('Ctrl Pts',(15.,-2.85358047685615,-2.5522851851895));
#24233=CARTESIAN_POINT('Ctrl Pts',(15.,-2.77668643075426,-2.64696770643963));
#24234=CARTESIAN_POINT('Ctrl Pts',(15.,-2.69538003166737,-2.73821192706575));
#24235=CARTESIAN_POINT('Ctrl Pts',(15.,-2.60995605577262,-2.82572098699874));
#24236=CARTESIAN_POINT('Ctrl Pts',(15.,-2.55533062672409,-2.88167974909572));
#24237=CARTESIAN_POINT('Ctrl Pts',(15.,-2.49902056538751,-2.93611060646992));
#24238=CARTESIAN_POINT('Ctrl Pts',(15.,-2.44109466904705,-2.98892841607831));
#24239=CARTESIAN_POINT('Ctrl Pts',(15.,-2.41749244372008,-3.01044932334795));
#24240=CARTESIAN_POINT('Ctrl Pts',(15.,-2.39362188975801,-3.03170235637655));
#24241=CARTESIAN_POINT('Ctrl Pts',(15.,-2.36948739594367,-3.0526814236989));
#24242=CARTESIAN_POINT('Ctrl Pts',(15.,-2.35462633600607,-3.06559949769335));
#24243=CARTESIAN_POINT('Ctrl Pts',(15.,-2.33966395888483,-3.07841463134345));
#24244=CARTESIAN_POINT('Ctrl Pts',(15.,-2.32461750573873,-3.09111197026854));
#24245=CARTESIAN_POINT('Ctrl Pts',(15.,-2.2294342138806,-3.17143485467153));
#24246=CARTESIAN_POINT('Ctrl Pts',(15.,-2.1307475718697,-3.24717166060831));
#24247=CARTESIAN_POINT('Ctrl Pts',(15.,-2.02890261537899,-3.31805078240874));
#24248=CARTESIAN_POINT('Ctrl Pts',(15.,-1.92724043909641,-3.38880269810018));
#24249=CARTESIAN_POINT('Ctrl Pts',(15.,-1.82243067018098,-3.45471500591087));
#24250=CARTESIAN_POINT('Ctrl Pts',(15.,-1.71477564167398,-3.51548571648839));
#24251=CARTESIAN_POINT('Ctrl Pts',(15.,-1.6070666174637,-3.57628690736305));
#24252=CARTESIAN_POINT('Ctrl Pts',(15.,-1.49650889611397,-3.63194202719247));
#24253=CARTESIAN_POINT('Ctrl Pts',(15.,-1.38337320787942,-3.68210666696541));
#24254=CARTESIAN_POINT('Ctrl Pts',(15.,-1.27023751964487,-3.73227130673836));
#24255=CARTESIAN_POINT('Ctrl Pts',(15.,-1.15452327651166,-3.77694617659555));
#24256=CARTESIAN_POINT('Ctrl Pts',(15.,-1.03647793659398,-3.81573446232228));
#24257=CARTESIAN_POINT('Ctrl Pts',(-5.89440495331884,-1.50460803346933,
3.1863723461202));
#24258=CARTESIAN_POINT('Ctrl Pts',(-5.85483221666482,-2.56096624880367,
2.6875589984119));
#24259=CARTESIAN_POINT('Ctrl Pts',(-5.7756867433568,-4.12083736250477,0.565882107592299));
#24260=CARTESIAN_POINT('Ctrl Pts',(-5.65696853339476,-2.71711677464747,
-3.15455318962618));
#24261=CARTESIAN_POINT('Ctrl Pts',(-5.53825032343272,1.16346364900644,-3.99342346061016));
#24262=CARTESIAN_POINT('Ctrl Pts',(-5.41953211347069,3.98315669070171,-1.20222141896168));
#24263=CARTESIAN_POINT('Ctrl Pts',(-5.30081390350864,3.17803017110567,2.68595570733295));
#24264=CARTESIAN_POINT('Ctrl Pts',(-5.18209569354661,-0.520477180563039,
4.12779813317261));
#24265=CARTESIAN_POINT('Ctrl Pts',(-5.06337748358456,-3.74494492974617,
1.81293102525157));
#24266=CARTESIAN_POINT('Ctrl Pts',(-4.94465927362253,-3.56061979352912,
-2.1525824195332));
#24267=CARTESIAN_POINT('Ctrl Pts',(-4.82594106366048,-0.135078114281208,
-4.15845351012906));
#24268=CARTESIAN_POINT('Ctrl Pts',(-4.70722285369845,3.41338373023632,-2.37909235958642));
#24269=CARTESIAN_POINT('Ctrl Pts',(-4.58850464373641,3.85474686870501,1.56595294230416));
#24270=CARTESIAN_POINT('Ctrl Pts',(-4.46978643377438,0.787218792347394,
4.08552098175258));
#24271=CARTESIAN_POINT('Ctrl Pts',(-4.35106822381233,-2.99688953094326,
2.88615565105121));
#24272=CARTESIAN_POINT('Ctrl Pts',(-4.2323500138503,-4.05300639018084,-0.940413777248205));
#24273=CARTESIAN_POINT('Ctrl Pts',(-4.11363180388825,-1.41977030063975,
-3.9109435932429));
#24274=CARTESIAN_POINT('Ctrl Pts',(-3.99491359392623,2.50584675349696,-3.32144046072034));
#24275=CARTESIAN_POINT('Ctrl Pts',(-3.87619538396417,4.1504539432636,0.29148889536334));
#24276=CARTESIAN_POINT('Ctrl Pts',(-3.75747717400214,2.01700539684609,3.63908250952178));
#24277=CARTESIAN_POINT('Ctrl Pts',(-3.6387589640401,-1.9524731306016,3.67410969416408));
#24278=CARTESIAN_POINT('Ctrl Pts',(-3.52004075407806,-4.14466374650587,
0.364685577384703));
#24279=CARTESIAN_POINT('Ctrl Pts',(-3.40132254411603,-2.56406948928158,
-3.2767027063953));
#24280=CARTESIAN_POINT('Ctrl Pts',(-3.28260433415398,1.35053375419133,-3.93538965177946));
#24281=CARTESIAN_POINT('Ctrl Pts',(-3.16388612419195,4.03577955172485,-1.0117887612591));
#24282=CARTESIAN_POINT('Ctrl Pts',(-3.0451679142299,3.04735509174485,2.83281838700313));
#24283=CARTESIAN_POINT('Ctrl Pts',(-2.92644970426787,-0.715001293115481,
4.09878106793642));
#24284=CARTESIAN_POINT('Ctrl Pts',(-2.80773149430582,-3.82650969623519,
1.63372477135958));
#24285=CARTESIAN_POINT('Ctrl Pts',(-2.68901328434379,-3.4548410165288,-2.31847075303888));
#24286=CARTESIAN_POINT('Ctrl Pts',(-2.57029507438175,0.0616839434797912,
-4.16021972695477));
#24287=CARTESIAN_POINT('Ctrl Pts',(-2.45157686441971,3.52205953641558,-2.21502363553932));
#24288=CARTESIAN_POINT('Ctrl Pts',(-2.33285865445767,3.77639149338881,1.74645365601417));
#24289=CARTESIAN_POINT('Ctrl Pts',(-2.21414044449563,0.593167728051762,
4.11817740399618));
#24290=CARTESIAN_POINT('Ctrl Pts',(-2.09542223453359,-3.13000194108223,
2.74122617326354));
#24291=CARTESIAN_POINT('Ctrl Pts',(-1.97670402457155,-4.00400830115146,
-1.13099540603816));
#24292=CARTESIAN_POINT('Ctrl Pts',(-1.85798581460952,-1.233264991575,-3.97369985590045));
#24293=CARTESIAN_POINT('Ctrl Pts',(-1.73926760464748,2.66008892032246,-3.19924366376966));
#24294=CARTESIAN_POINT('Ctrl Pts',(-1.62054939468544,4.13202971706382,0.487404864048419));
#24295=CARTESIAN_POINT('Ctrl Pts',(-1.5018311847234,1.8426861173841,3.73038080589689));
#24296=CARTESIAN_POINT('Ctrl Pts',(-1.38311297476136,-2.12400905413959,
3.57768341558217));
#24297=CARTESIAN_POINT('Ctrl Pts',(-1.26439476479932,-4.1572713463681,0.168309348719648));
#24298=CARTESIAN_POINT('Ctrl Pts',(-1.14567655483728,-2.40627241167155,
-3.39427255314433));
#24299=CARTESIAN_POINT('Ctrl Pts',(-1.02695834487524,1.53509675153174,-3.86713214768211));
#24300=CARTESIAN_POINT('Ctrl Pts',(-0.908240134913205,4.07910533073667,
-0.819837047806264));
#24301=CARTESIAN_POINT('Ctrl Pts',(-0.789521924951166,2.91000527267733,
2.97373542824345));
#24302=CARTESIAN_POINT('Ctrl Pts',(-0.670803714989128,-0.908000571423945,
4.06039013476461));
#24303=CARTESIAN_POINT('Ctrl Pts',(-0.552085505027088,-3.89947596557817,
1.45097218377135));
#24304=CARTESIAN_POINT('Ctrl Pts',(-0.43336729506505,-3.34135488829783,
-2.47922983901215));
#24305=CARTESIAN_POINT('Ctrl Pts',(-0.31464908510301,0.258318855548078,
-4.15265029265267));
#24306=CARTESIAN_POINT('Ctrl Pts',(-0.195930875140972,3.62285133778538,
-2.04601595020828));
#24307=CARTESIAN_POINT('Ctrl Pts',(-0.0772126651789335,3.68959190165954,
1.92305607911166));
#24308=CARTESIAN_POINT('Ctrl Pts',(0.0415055447831062,0.397788263499511,
4.14161774933685));
#24309=CARTESIAN_POINT('Ctrl Pts',(0.160223754745144,-3.25611218688863,
2.59016727463602));
#24310=CARTESIAN_POINT('Ctrl Pts',(0.278941964707183,-3.94605429230943,
-1.31904837149603));
#24311=CARTESIAN_POINT('Ctrl Pts',(0.397660174669222,-1.04400082814246,
-4.02756692744365));
#24312=CARTESIAN_POINT('Ctrl Pts',(0.516378384631262,2.80838075407454,-3.06989097922772));
#24313=CARTESIAN_POINT('Ctrl Pts',(0.635096594593299,4.10436283463961,0.682230757023696));
#24314=CARTESIAN_POINT('Ctrl Pts',(0.75381480455534,1.66424499718303,3.81333471826842));
#24315=CARTESIAN_POINT('Ctrl Pts',(0.872533014517378,-2.29079387626655,
3.47325445377382));
#24316=CARTESIAN_POINT('Ctrl Pts',(0.991251224479415,-4.16057977425022,
-0.0284433876307468));
#24317=CARTESIAN_POINT('Ctrl Pts',(1.10996943444146,-2.24309286528101,-3.50424991716136));
#24318=CARTESIAN_POINT('Ctrl Pts',(1.22868764440349,1.71622596930723,-3.79022446650269));
#24319=CARTESIAN_POINT('Ctrl Pts',(1.34740585436554,4.11330677534691,-0.626051480379392));
#24320=CARTESIAN_POINT('Ctrl Pts',(1.46612406432757,2.7661462154741,3.10800067548548));
#24321=CARTESIAN_POINT('Ctrl Pts',(1.58484227428961,-1.09896879073751,4.01291672990917));
#24322=CARTESIAN_POINT('Ctrl Pts',(1.70356048425165,-3.96371970283678,1.26497399243763));
#24323=CARTESIAN_POINT('Ctrl Pts',(1.82227869421369,-3.22039465930975,-2.63444326613598));
#24324=CARTESIAN_POINT('Ctrl Pts',(1.94099690417573,0.454375947728439,-4.13579201391049));
#24325=CARTESIAN_POINT('Ctrl Pts',(2.05971511413777,3.71553937395602,-1.87243163954858));
#24326=CARTESIAN_POINT('Ctrl Pts',(2.17843332409981,3.594539256238,2.09535691937294));
#24327=CARTESIAN_POINT('Ctrl Pts',(2.29715153406184,0.201519007352503,4.15579392822546));
#24328=CARTESIAN_POINT('Ctrl Pts',(2.41586974402388,-3.37493900695059,2.43331456732649));
#24329=CARTESIAN_POINT('Ctrl Pts',(2.53458795398592,-3.87927356258216,-1.5041508271617));
#24330=CARTESIAN_POINT('Ctrl Pts',(2.65330616394796,-0.852401394279078,
-4.07242494678922));
#24331=CARTESIAN_POINT('Ctrl Pts',(2.77202437391,2.95039066892461,-2.93367141734082));
#24332=CARTESIAN_POINT('Ctrl Pts',(2.89074258387204,4.06751511929676,0.875530603972367));
#24333=CARTESIAN_POINT('Ctrl Pts',(3.00946079383408,1.48208121505632,3.88775878317795));
#24334=CARTESIAN_POINT('Ctrl Pts',(3.12817900379612,-2.45245454230029,3.36105635212366));
#24335=CARTESIAN_POINT('Ctrl Pts',(3.24689721375816,-4.1545816205045,-0.225132500466264));
#24336=CARTESIAN_POINT('Ctrl Pts',(3.3656154237202,-2.07489586267471,-3.60638880921834));
#24337=CARTESIAN_POINT('Ctrl Pts',(3.48433363368223,1.89351625165984,-3.70483863196498));
#24338=CARTESIAN_POINT('Ctrl Pts',(3.60305184364428,4.13830738080923,-0.430865531390001));
#24339=CARTESIAN_POINT('Ctrl Pts',(3.72177005360631,2.6160997115818,3.23531379981317));
#24340=CARTESIAN_POINT('Ctrl Pts',(3.84048826356835,-1.28747878468051,3.95646704310772));
#24341=CARTESIAN_POINT('Ctrl Pts',(3.95920647353038,-4.01909720438648,1.07614624744637));
#24342=CARTESIAN_POINT('Ctrl Pts',(4.07792468349243,-3.09223089922823,-2.78376384595717));
#24343=CARTESIAN_POINT('Ctrl Pts',(4.19664289345446,0.649416670297701,-4.10968259997526));
#24344=CARTESIAN_POINT('Ctrl Pts',(4.3153611034165,3.79991631591589,-1.69465898523452));
#24345=CARTESIAN_POINT('Ctrl Pts',(4.43407931337854,3.49144617539216,2.26297076616989));
#24346=CARTESIAN_POINT('Ctrl Pts',(4.55279752334059,0.00479898395836184,
4.16067423069304));
#24347=CARTESIAN_POINT('Ctrl Pts',(4.67151573330262,-3.48621660381262,2.27101890690085));
#24348=CARTESIAN_POINT('Ctrl Pts',(4.79023394326466,-3.80381549026664,-1.68588872711323));
#24349=CARTESIAN_POINT('Ctrl Pts',(4.90895215322669,-0.658895268659781,
-4.10817357339461));
#24350=CARTESIAN_POINT('Ctrl Pts',(5.02767036318875,3.08580101037766,-2.79088968046971));
#24351=CARTESIAN_POINT('Ctrl Pts',(5.14638857315077,4.02156899374811,1.06687202265491));
#24352=CARTESIAN_POINT('Ctrl Pts',(5.26510678311282,1.29660224356769,3.95348652535647));
#24353=CARTESIAN_POINT('Ctrl Pts',(5.38382499307485,-2.60862944201661,3.24134008065248));
#24354=CARTESIAN_POINT('Ctrl Pts',(5.5025432030369,-4.13929030208498,-0.421318026276293));
#24355=CARTESIAN_POINT('Ctrl Pts',(5.62126141299893,-1.90205763486351,-3.70046076021046));
#24356=CARTESIAN_POINT('Ctrl Pts',(5.73997962296098,2.06657102730044,-3.61116563914235));
#24357=CARTESIAN_POINT('Ctrl Pts',(5.85869783292301,4.15405122458681,-0.23471580200077));
#24358=CARTESIAN_POINT('Ctrl Pts',(5.97741604288506,2.46020139211735,3.35539002120827));
#24359=CARTESIAN_POINT('Ctrl Pts',(6.09613425284709,-1.47310888518228,3.89116734368968));
#24360=CARTESIAN_POINT('Ctrl Pts',(6.21485246280913,-4.06548459921251,0.884911327628835));
#24361=CARTESIAN_POINT('Ctrl Pts',(6.33357067277116,-2.95715029081375,-2.92685757114013));
#24362=CARTESIAN_POINT('Ctrl Pts',(6.45228888273322,0.843004746942437,-4.07438045361901));
#24363=CARTESIAN_POINT('Ctrl Pts',(6.57100709269524,3.87579342533039,-1.51309563754761));
#24364=CARTESIAN_POINT('Ctrl Pts',(6.68972530265728,3.38054326260136,2.42552269292219));
#24365=CARTESIAN_POINT('Ctrl Pts',(6.80844351261932,-0.191931774030066,
4.15624774024814));
#24366=CARTESIAN_POINT('Ctrl Pts',(6.92716172258136,-3.58969606648277,2.10364332396875));
#24367=CARTESIAN_POINT('Ctrl Pts',(7.0458799325434,-3.71984886354811,-1.86385555142016));
#24368=CARTESIAN_POINT('Ctrl Pts',(7.16459814250543,-0.463915294938845,
-4.13473284304098));
#24369=CARTESIAN_POINT('Ctrl Pts',(7.28331635246748,3.21430888617722,-2.64186514955669));
#24370=CARTESIAN_POINT('Ctrl Pts',(7.40203456242951,3.96662723246049,1.25582701153581));
#24371=CARTESIAN_POINT('Ctrl Pts',(7.52075277239156,1.1082229708534,4.01037092188151));
#24372=CARTESIAN_POINT('Ctrl Pts',(7.63947098235359,-2.75896923601302,3.11437342637868));
#24373=CARTESIAN_POINT('Ctrl Pts',(7.75818919231563,-4.11474002333594,-0.61656112799747));
#24374=CARTESIAN_POINT('Ctrl Pts',(7.87690740227768,-1.7249647945704,-3.78625534554826));
#24375=CARTESIAN_POINT('Ctrl Pts',(7.9956256122397,2.2350031991217,-3.50941502021571));
#24376=CARTESIAN_POINT('Ctrl Pts',(8.11434382220176,4.16050309010526,-0.0380410492039316));
#24377=CARTESIAN_POINT('Ctrl Pts',(8.23306203216378,2.2987999778154,3.46796074749932));
#24378=CARTESIAN_POINT('Ctrl Pts',(8.35178024212583,-1.65544386605393,3.81716369711131));
#24379=CARTESIAN_POINT('Ctrl Pts',(8.47049845208786,-4.10277812579614,0.691696996298736));
#24380=CARTESIAN_POINT('Ctrl Pts',(8.5892166620499,-2.81545498876027,-3.06340436287227));
#24381=CARTESIAN_POINT('Ctrl Pts',(8.70793487201195,1.03470715069641,-4.02996454035241));
#24382=CARTESIAN_POINT('Ctrl Pts',(8.82665308197397,3.9430009766923,-1.32814772597166));
#24383=CARTESIAN_POINT('Ctrl Pts',(8.94537129193603,3.26207859074647,2.58264909579165));
#24384=CARTESIAN_POINT('Ctrl Pts',(9.06408950189805,-0.388233209948286,
4.14252435827397));
#24385=CARTESIAN_POINT('Ctrl Pts',(9.1828077118601,-3.68514592720451,1.93156221215062));
#24386=CARTESIAN_POINT('Ctrl Pts',(9.30152592182213,-3.62756150294873,-2.03765321547226));
#24387=CARTESIAN_POINT('Ctrl Pts',(9.42024413178417,-0.267897613543705,
-4.1520433466978));
#24388=CARTESIAN_POINT('Ctrl Pts',(9.53896234174623,3.33562684382852,-2.48693116972114));
#24389=CARTESIAN_POINT('Ctrl Pts',(9.65768055170824,3.90281273176416,1.44197290715868));
#24390=CARTESIAN_POINT('Ctrl Pts',(9.77639876167031,0.917364772580788,4.05828473104436));
#24391=CARTESIAN_POINT('Ctrl Pts',(9.89511697163233,-2.90313763712753,2.98044039431988));
#24392=CARTESIAN_POINT('Ctrl Pts',(10.0138351815944,-4.08098569948204,-0.810425076625216));
#24393=CARTESIAN_POINT('Ctrl Pts',(10.1325533915564,-1.54401347143674,-3.86358065584526));
#24394=CARTESIAN_POINT('Ctrl Pts',(10.2512716015185,2.3984360100751,-3.39981437578226));
#24395=CARTESIAN_POINT('Ctrl Pts',(10.3699898114805,4.15764854552659,0.158718795611215));
#24396=CARTESIAN_POINT('Ctrl Pts',(10.4887080214425,2.13225649899359,3.57277417516111));
#24397=CARTESIAN_POINT('Ctrl Pts',(10.6074262314046,-1.83407587178631,3.73462163822996));
#24398=CARTESIAN_POINT('Ctrl Pts',(10.7261444413666,-4.13089436421284,0.496935444410325));
#24399=CARTESIAN_POINT('Ctrl Pts',(10.8448626513286,-2.66746194382199,-3.1930987868298));
#24400=CARTESIAN_POINT('Ctrl Pts',(10.9635808612907,1.22409507255686,-3.97653421179419));
#24401=CARTESIAN_POINT('Ctrl Pts',(11.0822990712527,4.00138863696973,-1.14022895073704));
#24402=CARTESIAN_POINT('Ctrl Pts',(11.2010172812148,3.13631714721284,2.73399850699711));
#24403=CARTESIAN_POINT('Ctrl Pts',(11.3197354911768,-0.583666227467498,
4.11953478190202));
#24404=CARTESIAN_POINT('Ctrl Pts',(11.4384537011388,-3.77235267919998,1.75516049057551));
#24405=CARTESIAN_POINT('Ctrl Pts',(11.5571719111009,-3.52715984122978,-2.20689296035622));
#24406=CARTESIAN_POINT('Ctrl Pts',(11.6758901210629,-0.071280686042087,
-4.16006636356011));
#24407=CARTESIAN_POINT('Ctrl Pts',(11.7946083310249,3.44948351348419,-2.32643430433509));
#24408=CARTESIAN_POINT('Ctrl Pts',(11.913326540987,3.83026823514579,1.62489332904317));
#24409=CARTESIAN_POINT('Ctrl Pts',(12.032044750949,0.724454569027592,4.09712077799104));
#24410=CARTESIAN_POINT('Ctrl Pts',(12.1507629609111,-3.04081216196281,2.83984057027597));
#24411=CARTESIAN_POINT('Ctrl Pts',(12.2694811708731,-4.03810283512032,-1.00247622441819));
#24412=CARTESIAN_POINT('Ctrl Pts',(12.3881993808351,-1.35960842341351,-3.93226373321093));
#24413=CARTESIAN_POINT('Ctrl Pts',(12.5069175907972,2.55650388111248,-3.28260885239469));
#24414=CARTESIAN_POINT('Ctrl Pts',(12.6256358007592,4.14549398517236,0.355123585322626));
#24415=CARTESIAN_POINT('Ctrl Pts',(12.7443540107213,1.96094347059736,3.66959590085791));
#24416=CARTESIAN_POINT('Ctrl Pts',(12.8630722206833,-2.008605296796,3.64372570917414));
#24417=CARTESIAN_POINT('Ctrl Pts',(12.9817904306453,-4.14977048561323,0.301062498504729));
#24418=CARTESIAN_POINT('Ctrl Pts',(13.1005086406074,-2.51350207424876,-3.31565106862418));
#24419=CARTESIAN_POINT('Ctrl Pts',(13.2192268505694,1.41074465321508,-3.91420835157396));
#24420=CARTESIAN_POINT('Ctrl Pts',(13.3379450605315,4.05082623445229,-0.949760859141879));
#24421=CARTESIAN_POINT('Ctrl Pts',(13.4566632704935,3.00353941846475,2.8792346664523));
#24422=CARTESIAN_POINT('Ctrl Pts',(13.5753814804555,-0.777792108158467,
4.08732608875924));
#24423=CARTESIAN_POINT('Ctrl Pts',(13.6940996904176,-3.85112422993177,1.57484100941476));
#24424=CARTESIAN_POINT('Ctrl Pts',(13.8128179003796,-3.4188628023499,-2.37121194413166));
#24425=CARTESIAN_POINT('Ctrl Pts',(13.9315361103417,0.125484922544878,-4.15875404743734));
#24426=CARTESIAN_POINT('Ctrl Pts',(14.0502543203037,3.55564468470245,-2.16079042553925));
#24427=CARTESIAN_POINT('Ctrl Pts',(14.1689725302657,3.74911708348173,1.80428726191164));
#24428=CARTESIAN_POINT('Ctrl Pts',(14.2876907402278,0.529997911397081,4.12658649947203));
#24429=CARTESIAN_POINT('Ctrl Pts',(14.4064089501898,-3.1718256804096,2.69327972615298));
#24430=CARTESIAN_POINT('Ctrl Pts',(14.5251271601518,-3.98591940928569,-1.19302976726136));
#24431=CARTESIAN_POINT('Ctrl Pts',(14.6438453701139,-1.17267268992146,-3.99072892597622));
#24432=CARTESIAN_POINT('Ctrl Pts',(14.7625635800759,2.70983253704952,-3.16081271422384));
#24433=CARTESIAN_POINT('Ctrl Pts',(14.881281790038,4.12213179013054,0.556374543543842));
#24434=CARTESIAN_POINT('Ctrl Pts',(14.960427263346,2.56715916810242,2.68164414176901));
#24435=CARTESIAN_POINT('Ctrl Pts',(15.,1.51195443948848,3.18289299779479));
#24436=CARTESIAN_POINT('Ctrl Pts',(-5.81160330221256,-1.56584559822282,
3.31605773828462));
#24437=CARTESIAN_POINT('Ctrl Pts',(-5.77203056555855,-2.66519760541219,
2.79694268142636));
#24438=CARTESIAN_POINT('Ctrl Pts',(-5.69288509225052,-4.28855549188565,
0.588913516062578));
#24439=CARTESIAN_POINT('Ctrl Pts',(-5.57416688228849,-2.82770345950423,
-3.28294354174507));
#24440=CARTESIAN_POINT('Ctrl Pts',(-5.45544867232644,1.21081663327842,-4.15595584267732));
#24441=CARTESIAN_POINT('Ctrl Pts',(-5.33673046236441,4.1452712151122,-1.2511518449291));
#24442=CARTESIAN_POINT('Ctrl Pts',(-5.21801225240236,3.30737603664836,2.79527413638156));
#24443=CARTESIAN_POINT('Ctrl Pts',(-5.09929404244033,-0.541660607966363,
4.29579956600198));
#24444=CARTESIAN_POINT('Ctrl Pts',(-4.98057583247828,-3.89736423266904,
1.88671733941634));
#24445=CARTESIAN_POINT('Ctrl Pts',(-4.86185762251625,-3.70553706122838,
-2.24019254946148));
#24446=CARTESIAN_POINT('Ctrl Pts',(-4.74313941255421,-0.140575795129675,
-4.32770261716304));
#24447=CARTESIAN_POINT('Ctrl Pts',(-4.62442120259217,3.55230848841859,-2.47592144675321));
#24448=CARTESIAN_POINT('Ctrl Pts',(-4.50570299263013,4.01163511184185,1.6296872455726));
#24449=CARTESIAN_POINT('Ctrl Pts',(-4.3869847826681,0.819258606504406,4.25180173401925));
#24450=CARTESIAN_POINT('Ctrl Pts',(-4.26826657270605,-3.11886297028946,
3.0036222201764));
#24451=CARTESIAN_POINT('Ctrl Pts',(-4.14954836274402,-4.21796379818607,
-0.978688629102168));
#24452=CARTESIAN_POINT('Ctrl Pts',(-4.03083015278197,-1.47755496866388,
-4.07011904373294));
#24453=CARTESIAN_POINT('Ctrl Pts',(-3.91211194281994,2.60783474599474,-3.4566231267461));
#24454=CARTESIAN_POINT('Ctrl Pts',(-3.7933937328579,4.31937746783157,0.303352496851359));
#24455=CARTESIAN_POINT('Ctrl Pts',(-3.67467552289586,2.09909754034784,3.78719321068975));
#24456=CARTESIAN_POINT('Ctrl Pts',(-3.55595731293382,-2.03193881010417,
3.82364600216115));
#24457=CARTESIAN_POINT('Ctrl Pts',(-3.43723910297178,-4.31335160999734,
0.37952828469648));
#24458=CARTESIAN_POINT('Ctrl Pts',(-3.31852089300974,-2.66842714781423,
-3.41006454529105));
#24459=CARTESIAN_POINT('Ctrl Pts',(-3.1998026830477,1.40550049395635,-4.09556005714099));
#24460=CARTESIAN_POINT('Ctrl Pts',(-3.08108447308566,4.20003582720122,-1.05296857580625));
#24461=CARTESIAN_POINT('Ctrl Pts',(-2.96236626312363,3.17138248001238,2.94811412885089));
#24462=CARTESIAN_POINT('Ctrl Pts',(-2.84364805316159,-0.744101854199846,
4.26560150586757));
#24463=CARTESIAN_POINT('Ctrl Pts',(-2.72492984319955,-3.98224868611863,
1.70021738887191));
#24464=CARTESIAN_POINT('Ctrl Pts',(-2.60621163323751,-3.59545308675336,
-2.41283254010238));
#24465=CARTESIAN_POINT('Ctrl Pts',(-2.48749342327547,0.0641944807088134,
-4.32954071903444));
#24466=CARTESIAN_POINT('Ctrl Pts',(-2.36877521331343,3.66540740119438,-2.30517512369736));
#24467=CARTESIAN_POINT('Ctrl Pts',(-2.25005700335139,3.93009067182376,1.81753434046494));
#24468=CARTESIAN_POINT('Ctrl Pts',(-2.13133879338935,0.617309661597382,
4.28578727303431));
#24469=CARTESIAN_POINT('Ctrl Pts',(-2.01262058342732,-3.25739305709507,
2.85279411092906));
#24470=CARTESIAN_POINT('Ctrl Pts',(-1.89390237346528,-4.16697148635381,
-1.17702693243741));
#24471=CARTESIAN_POINT('Ctrl Pts',(-1.77518416350324,-1.28345889131487,
-4.13542948702271));
#24472=CARTESIAN_POINT('Ctrl Pts',(-1.6564659535412,2.76835457083388,-3.32945291871461));
#24473=CARTESIAN_POINT('Ctrl Pts',(-1.53774774357916,4.3002033754076,0.507242247778535));
#24474=CARTESIAN_POINT('Ctrl Pts',(-1.41902953361712,1.91768346415051,3.88220734880688));
#24475=CARTESIAN_POINT('Ctrl Pts',(-1.30031132365508,-2.21045624775848,
3.72329517290076));
#24476=CARTESIAN_POINT('Ctrl Pts',(-1.18159311369304,-4.32647233932304,
0.175159541202699));
#24477=CARTESIAN_POINT('Ctrl Pts',(-1.062874903731,-2.5042077272796,-3.53241948619297));
#24478=CARTESIAN_POINT('Ctrl Pts',(-0.944156693768965,1.59757520747088,
-4.02452447181977));
#24479=CARTESIAN_POINT('Ctrl Pts',(-0.825438483806927,4.24512496593113,
-0.853204425346146));
#24480=CARTESIAN_POINT('Ctrl Pts',(-0.706720273844886,3.02844252168471,
3.09476649533597));
#24481=CARTESIAN_POINT('Ctrl Pts',(-0.588002063882849,-0.944956205417587,
4.22564806126171));
#24482=CARTESIAN_POINT('Ctrl Pts',(-0.46928385392081,-4.05818468348666,
1.51002676880789));
#24483=CARTESIAN_POINT('Ctrl Pts',(-0.350565643958771,-3.47734807176147,
-2.58013452277567));
#24484=CARTESIAN_POINT('Ctrl Pts',(-0.231847433996732,0.268832436023395,
-4.32166320866675));
#24485=CARTESIAN_POINT('Ctrl Pts',(-0.113129224034693,3.77030143007175,
-2.1292888235749));
#24486=CARTESIAN_POINT('Ctrl Pts',(0.00558898592734564,3.83975833568475,
2.00132448427074));
#24487=CARTESIAN_POINT('Ctrl Pts',(0.124307195889385,0.413978250527581,
4.31018164070752));
#24488=CARTESIAN_POINT('Ctrl Pts',(0.243025405851424,-3.38863599139698,
2.69558711334118));
#24489=CARTESIAN_POINT('Ctrl Pts',(0.361743615813462,-4.10665874866663,
-1.37273365581305));
#24490=CARTESIAN_POINT('Ctrl Pts',(0.480461825775502,-1.08649167419266,
-4.19148894901468));
#24491=CARTESIAN_POINT('Ctrl Pts',(0.59918003573754,2.92268188397315,-3.19483557838227));
#24492=CARTESIAN_POINT('Ctrl Pts',(0.717898245699579,4.27141045054158,0.709997556901627));
#24493=CARTESIAN_POINT('Ctrl Pts',(0.836616455661619,1.73197978824728,3.96853748639282));
#24494=CARTESIAN_POINT('Ctrl Pts',(0.955334665623657,-2.38402921411817,
3.61461595111198));
#24495=CARTESIAN_POINT('Ctrl Pts',(1.0740528755857,-4.32991542025907,-0.0296010338436595));
#24496=CARTESIAN_POINT('Ctrl Pts',(1.19277108554774,-2.33438677142145,-3.64687293022593));
#24497=CARTESIAN_POINT('Ctrl Pts',(1.31148929550977,1.78607638655161,-3.94448664710694));
#24498=CARTESIAN_POINT('Ctrl Pts',(1.43020750547181,4.28071840974142,-0.651531783033579));
#24499=CARTESIAN_POINT('Ctrl Pts',(1.54892571543385,2.87872839915225,3.23449633972838));
#24500=CARTESIAN_POINT('Ctrl Pts',(1.66764392539589,-1.14369683351533,4.17624248826731));
#24501=CARTESIAN_POINT('Ctrl Pts',(1.78636213535792,-4.12504314161134,1.31645844888754));
#24502=CARTESIAN_POINT('Ctrl Pts',(1.90508034531997,-3.35146476002329,-2.74166513821877));
#24503=CARTESIAN_POINT('Ctrl Pts',(2.023798555282,0.472869054173783,-4.30411879778042));
#24504=CARTESIAN_POINT('Ctrl Pts',(2.14251676524405,3.86676187041052,-1.94863962941881));
#24505=CARTESIAN_POINT('Ctrl Pts',(2.26123497520608,3.7408370464706,2.18063797076803));
#24506=CARTESIAN_POINT('Ctrl Pts',(2.37995318516813,0.2097208333346,4.32493479024452));
#24507=CARTESIAN_POINT('Ctrl Pts',(2.49867139513016,-3.51229906444054,2.53235049898945));
#24508=CARTESIAN_POINT('Ctrl Pts',(2.6173896050922,-4.03716004244981,-1.56536978361307));
#24509=CARTESIAN_POINT('Ctrl Pts',(2.73610781505424,-0.88709414110546,-4.23817269027803));
#24510=CARTESIAN_POINT('Ctrl Pts',(2.85482602501628,3.07047160403682,-3.05307187871585));
#24511=CARTESIAN_POINT('Ctrl Pts',(2.97354423497831,4.23306303274856,0.911164709906788));
#24512=CARTESIAN_POINT('Ctrl Pts',(3.09226244494036,1.542401938034,4.04599061162419));
#24513=CARTESIAN_POINT('Ctrl Pts',(3.2109806549024,-2.55226947117104,3.49785138539797));
#24514=CARTESIAN_POINT('Ctrl Pts',(3.32969886486443,-4.32367314158497,-0.234295395897341));
#24515=CARTESIAN_POINT('Ctrl Pts',(3.44841707482648,-2.15934414882022,-3.75316887639737));
#24516=CARTESIAN_POINT('Ctrl Pts',(3.56713528478851,1.97058238549235,-3.8556256080939));
#24517=CARTESIAN_POINT('Ctrl Pts',(3.68585349475056,4.30673654014168,-0.448401763612337));
#24518=CARTESIAN_POINT('Ctrl Pts',(3.80457170471259,2.7225750007773,3.36699110972162));
#24519=CARTESIAN_POINT('Ctrl Pts',(3.92328991467463,-1.33987918644085,4.11749529854554));
#24520=CARTESIAN_POINT('Ctrl Pts',(4.04200812463667,-4.18267450812892,1.11994541244234));
#24521=CARTESIAN_POINT('Ctrl Pts',(4.16072633459871,-3.21808473339097,-2.89706306740433));
#24522=CARTESIAN_POINT('Ctrl Pts',(4.27944454456075,0.675847936457875,-4.27694673038929));
#24523=CARTESIAN_POINT('Ctrl Pts',(4.39816275452279,3.95457295490588,-1.76363162597209));
#24524=CARTESIAN_POINT('Ctrl Pts',(4.51688096448482,3.6335480760153,2.35507370311157));
#24525=CARTESIAN_POINT('Ctrl Pts',(4.63559917444687,0.00499430266219868,
4.33001372108024));
#24526=CARTESIAN_POINT('Ctrl Pts',(4.7543173844089,-3.62810566081065,2.36344940326542));
#24527=CARTESIAN_POINT('Ctrl Pts',(4.87303559437094,-3.9586308256988,-1.75450441824159));
#24528=CARTESIAN_POINT('Ctrl Pts',(4.99175380433298,-0.685712313885341,
-4.27537628640897));
#24529=CARTESIAN_POINT('Ctrl Pts',(5.11047201429502,3.21139314798817,-2.90447892346575));
#24530=CARTESIAN_POINT('Ctrl Pts',(5.22919022425705,4.18524689934679,1.11029372659223));
#24531=CARTESIAN_POINT('Ctrl Pts',(5.3479084342191,1.34937397021258,4.11439347368658));
#24532=CARTESIAN_POINT('Ctrl Pts',(5.46662664418113,-2.7148006911525,3.37326266026232));
#24533=CARTESIAN_POINT('Ctrl Pts',(5.58534485414318,-4.30775946632497,-0.438465674927635));
#24534=CARTESIAN_POINT('Ctrl Pts',(5.7040630641052,-1.97947140309336,-3.85106955690723));
#24535=CARTESIAN_POINT('Ctrl Pts',(5.82278127406726,2.1506804925478,-3.75814012335574));
#24536=CARTESIAN_POINT('Ctrl Pts',(5.94149948402928,4.32312115854718,-0.244268737917595));
#24537=CARTESIAN_POINT('Ctrl Pts',(6.06021769399133,2.56033161786722,3.49195443474735));
#24538=CARTESIAN_POINT('Ctrl Pts',(6.17893590395336,-1.53306443422802,4.04953790058903));
#24539=CARTESIAN_POINT('Ctrl Pts',(6.2976541139154,-4.23094987047288,0.920927229126973));
#24540=CARTESIAN_POINT('Ctrl Pts',(6.41637232387744,-3.07750634261675,-3.04598070889424));
#24541=CARTESIAN_POINT('Ctrl Pts',(6.53509053383949,0.87731505011114,-4.24020778625891));
#24542=CARTESIAN_POINT('Ctrl Pts',(6.65380874380152,4.03353826357076,-1.57467864788741));
#24543=CARTESIAN_POINT('Ctrl Pts',(6.77252695376357,3.51813141336254,2.52424149520478));
#24544=CARTESIAN_POINT('Ctrl Pts',(6.89124516372559,-0.199743399502607,
4.32540707242189));
#24545=CARTESIAN_POINT('Ctrl Pts',(7.00996337368766,-3.73579673883507,2.18926163212884));
#24546=CARTESIAN_POINT('Ctrl Pts',(7.12868158364966,-3.87124675627995,-1.93971449440218));
#24547=CARTESIAN_POINT('Ctrl Pts',(7.24739979361173,-0.482796652928421,
-4.30301651864399));
#24548=CARTESIAN_POINT('Ctrl Pts',(7.36611800357374,3.34513129585232,-2.74938909238243));
#24549=CARTESIAN_POINT('Ctrl Pts',(7.4848362135358,4.12806900772511,1.30693918575489));
#24550=CARTESIAN_POINT('Ctrl Pts',(7.60355442349783,1.15332765887133,4.17359306582282));
#24551=CARTESIAN_POINT('Ctrl Pts',(7.72227263345988,-2.87125931654226,3.24112846165826));
#24552=CARTESIAN_POINT('Ctrl Pts',(7.8409908434219,-4.28220999094055,-0.641655173197523));
#24553=CARTESIAN_POINT('Ctrl Pts',(7.95970905338396,-1.79517088210629,-3.94035598288275));
#24554=CARTESIAN_POINT('Ctrl Pts',(8.07842726334599,2.32596785575382,-3.65224825303564));
#24555=CARTESIAN_POINT('Ctrl Pts',(8.19714547330803,4.32983561506851,-0.039589320356336));
#24556=CARTESIAN_POINT('Ctrl Pts',(8.31586368327006,2.39236116409469,3.60910679092953));
#24557=CARTESIAN_POINT('Ctrl Pts',(8.43458189323211,-1.72282045097718,3.97252230471988));
#24558=CARTESIAN_POINT('Ctrl Pts',(8.55330010319414,-4.26976124402944,0.719849072227066));
#24559=CARTESIAN_POINT('Ctrl Pts',(8.67201831315618,-2.93004404009421,-3.18808495666448));
#24560=CARTESIAN_POINT('Ctrl Pts',(8.79073652311822,1.07681974396469,-4.19398414479716));
#24561=CARTESIAN_POINT('Ctrl Pts',(8.90945473308027,4.10348116306779,-1.38220335412341));
#24562=CARTESIAN_POINT('Ctrl Pts',(9.0281729430423,3.39484522796237,2.68776294452898));
#24563=CARTESIAN_POINT('Ctrl Pts',(9.14689115300434,-0.40403430618387,4.3111251486391));
#24564=CARTESIAN_POINT('Ctrl Pts',(9.26560936296638,-3.83513141001683,2.01017681702494));
#24565=CARTESIAN_POINT('Ctrl Pts',(9.38432757292842,-3.77520329901292,-2.12058572543627));
#24566=CARTESIAN_POINT('Ctrl Pts',(9.50304578289045,-0.278801049582681,
-4.32103156000434));
#24567=CARTESIAN_POINT('Ctrl Pts',(9.62176399285249,3.47138689581455,-2.58814929773555));
#24568=CARTESIAN_POINT('Ctrl Pts',(9.74048220281454,4.06165725609586,1.50066122153069));
#24569=CARTESIAN_POINT('Ctrl Pts',(9.85920041277656,0.954701529672213,4.22345696758516));
#24570=CARTESIAN_POINT('Ctrl Pts',(9.97791862273862,-3.02129537328685,3.10174435361097));
#24571=CARTESIAN_POINT('Ctrl Pts',(10.0966368327006,-4.24708186570667,-0.843409386826764));
#24572=CARTESIAN_POINT('Ctrl Pts',(10.2153550426627,-1.60685483798142,-4.02082843422318));
#24573=CARTESIAN_POINT('Ctrl Pts',(10.3340732526247,2.49605238404554,-3.53818686107777));
#24574=CARTESIAN_POINT('Ctrl Pts',(10.4527914625868,4.32686489049173,0.165178652469378));
#24575=CARTESIAN_POINT('Ctrl Pts',(10.5715096725488,2.21903936371554,3.71818612633653));
#24576=CARTESIAN_POINT('Ctrl Pts',(10.6902278825108,-1.9087227814551,3.88662078306603));
#24577=CARTESIAN_POINT('Ctrl Pts',(10.8089460924729,-4.29902181368216,0.517160722873837));
#24578=CARTESIAN_POINT('Ctrl Pts',(10.9276643024349,-2.77602767647701,-3.32305794521066));
#24579=CARTESIAN_POINT('Ctrl Pts',(11.046382512397,1.27391575648429,-4.13837920123483));
#24580=CARTESIAN_POINT('Ctrl Pts',(11.165100722359,4.16424520180891,-1.18663628251469));
#24581=CARTESIAN_POINT('Ctrl Pts',(11.2838189323211,3.26396529218985,2.84527227856014));
#24582=CARTESIAN_POINT('Ctrl Pts',(11.4025371422831,-0.607421449827014,
4.28719989623697));
#24583=CARTESIAN_POINT('Ctrl Pts',(11.5212553522451,-3.9258874778497,1.82659554329586));
#24584=CARTESIAN_POINT('Ctrl Pts',(11.6399735622072,-3.6707152884748,-2.29671352993819));
#24585=CARTESIAN_POINT('Ctrl Pts',(11.7586917721692,-0.0741818108068467,
-4.32938111374782));
#24586=CARTESIAN_POINT('Ctrl Pts',(11.8774099821312,3.5898775332715,-2.42112020803049));
#24587=CARTESIAN_POINT('Ctrl Pts',(11.9961281920933,3.98616019760731,1.69102650674882));
#24588=CARTESIAN_POINT('Ctrl Pts',(12.1148464020553,0.753939878553332,4.26387364210179));
#24589=CARTESIAN_POINT('Ctrl Pts',(12.2335646120174,-3.16457325291087,2.95542211506595));
#24590=CARTESIAN_POINT('Ctrl Pts',(12.3522828219794,-4.20245366825836,-1.04327701860583));
#24591=CARTESIAN_POINT('Ctrl Pts',(12.4710010319414,-1.41494450232315,-4.09230691364976));
#24592=CARTESIAN_POINT('Ctrl Pts',(12.5897192419035,2.66055361930321,-3.41621107150242));
#24593=CARTESIAN_POINT('Ctrl Pts',(12.7084374518655,4.31421563938737,0.369577119444437));
#24594=CARTESIAN_POINT('Ctrl Pts',(12.8271556618275,2.04075389303788,3.81894849741406));
#24595=CARTESIAN_POINT('Ctrl Pts',(12.9458738717896,-2.09035555612641,3.79202538862284));
#24596=CARTESIAN_POINT('Ctrl Pts',(13.0645920817516,-4.31866619344675,0.31331574575378));
#24597=CARTESIAN_POINT('Ctrl Pts',(13.1833102917137,-2.61580163839163,-3.45059810632319));
#24598=CARTESIAN_POINT('Ctrl Pts',(13.3020285016757,1.46816197728233,-4.07351667776667));
#24599=CARTESIAN_POINT('Ctrl Pts',(13.4207467116377,4.2156949100936,-0.98841613733941));
#24600=CARTESIAN_POINT('Ctrl Pts',(13.5394649215998,3.12578350831168,2.9964195514225));
#24601=CARTESIAN_POINT('Ctrl Pts',(13.6581831315618,-0.809448256157549,
4.25368030890243));
#24602=CARTESIAN_POINT('Ctrl Pts',(13.7769013415239,-4.00786503162771,1.63893705711967));
#24603=CARTESIAN_POINT('Ctrl Pts',(13.8956195514859,-3.55801055883195,-2.46772029829628));
#24604=CARTESIAN_POINT('Ctrl Pts',(14.0143377614479,0.130592160376269,-4.32801538634333));
#24605=CARTESIAN_POINT('Ctrl Pts',(14.13305597141,3.70035946541365,-2.248734621409));
#24606=CARTESIAN_POINT('Ctrl Pts',(14.251774181372,3.90170619311096,1.87772177480629));
#24607=CARTESIAN_POINT('Ctrl Pts',(14.370492391334,0.551568832657898,4.29453861879547));
#24608=CARTESIAN_POINT('Ctrl Pts',(14.4892106012961,-3.30091902310761,2.80289624285414));
#24609=CARTESIAN_POINT('Ctrl Pts',(14.6079288112581,-4.14814637637521,-1.24158609289592));
#24610=CARTESIAN_POINT('Ctrl Pts',(14.7266470212202,-1.22040048226755,-4.15315164045192));
#24611=CARTESIAN_POINT('Ctrl Pts',(14.8453652311822,2.82012275334993,-3.28945782906785));
#24612=CARTESIAN_POINT('Ctrl Pts',(14.9640834411443,4.2899026027311,0.579018994044959));
#24613=CARTESIAN_POINT('Ctrl Pts',(15.0432289144523,2.67164257659961,2.79078709004819));
#24614=CARTESIAN_POINT('Ctrl Pts',(15.0828016511063,1.57349100305379,3.31243678044123));
#24615=CARTESIAN_POINT('Ctrl Pts',(-5.72880165110628,-1.62708316297631,
3.44574313044905));
#24616=CARTESIAN_POINT('Ctrl Pts',(-5.68922891445227,-2.76942896202072,
2.90632636444082));
#24617=CARTESIAN_POINT('Ctrl Pts',(-5.61008344114424,-4.45627362126654,
0.611944924532856));
#24618=CARTESIAN_POINT('Ctrl Pts',(-5.4913652311822,-2.93829014436098,-3.41133389386395));
#24619=CARTESIAN_POINT('Ctrl Pts',(-5.37264702122016,1.2581696175504,-4.31848822474448));
#24620=CARTESIAN_POINT('Ctrl Pts',(-5.25392881125812,4.3073857395227,-1.30008227089652));
#24621=CARTESIAN_POINT('Ctrl Pts',(-5.13521060129609,3.43672190219105,2.90459256543017));
#24622=CARTESIAN_POINT('Ctrl Pts',(-5.01649239133405,-0.562844035369692,
4.46380099883135));
#24623=CARTESIAN_POINT('Ctrl Pts',(-4.89777418137201,-4.04978353559191,
1.96050365358111));
#24624=CARTESIAN_POINT('Ctrl Pts',(-4.77905597140997,-3.85045432892764,
-2.32780267938976));
#24625=CARTESIAN_POINT('Ctrl Pts',(-4.66033776144793,-0.146073475978136,
-4.49695172419703));
#24626=CARTESIAN_POINT('Ctrl Pts',(-4.54161955148589,3.69123324660085,-2.57275053391999));
#24627=CARTESIAN_POINT('Ctrl Pts',(-4.42290134152385,4.16852335497868,1.69342154884104));
#24628=CARTESIAN_POINT('Ctrl Pts',(-4.30418313156181,0.851298420661415,
4.41808248628593));
#24629=CARTESIAN_POINT('Ctrl Pts',(-4.18546492159977,-3.24083640963565,
3.12108878930159));
#24630=CARTESIAN_POINT('Ctrl Pts',(-4.06674671163774,-4.3829212061913,-1.01696348095613));
#24631=CARTESIAN_POINT('Ctrl Pts',(-3.9480285016757,-1.53533963668801,-4.22929449422298));
#24632=CARTESIAN_POINT('Ctrl Pts',(-3.82931029171366,2.70982273849253,-3.59180579277186));
#24633=CARTESIAN_POINT('Ctrl Pts',(-3.71059208175162,4.48830099239954,0.31521609833938));
#24634=CARTESIAN_POINT('Ctrl Pts',(-3.59187387178958,2.18118968384959,3.93530391185771));
#24635=CARTESIAN_POINT('Ctrl Pts',(-3.47315566182754,-2.11140448960673,
3.97318231015822));
#24636=CARTESIAN_POINT('Ctrl Pts',(-3.3544374518655,-4.4820394734888,0.394370992008255));
#24637=CARTESIAN_POINT('Ctrl Pts',(-3.23571924190347,-2.77278480634688,
-3.5434263841868));
#24638=CARTESIAN_POINT('Ctrl Pts',(-3.11700103194142,1.46046723372137,-4.25573046250252));
#24639=CARTESIAN_POINT('Ctrl Pts',(-2.99828282197939,4.3642921026776,-1.0941483903534));
#24640=CARTESIAN_POINT('Ctrl Pts',(-2.87956461201734,3.2954098682799,3.06340987069866));
#24641=CARTESIAN_POINT('Ctrl Pts',(-2.76084640205531,-0.773202415284208,
4.43242194379871));
#24642=CARTESIAN_POINT('Ctrl Pts',(-2.64212819209327,-4.13798767600206,
1.76671000638425));
#24643=CARTESIAN_POINT('Ctrl Pts',(-2.52340998213123,-3.73606515697793,
-2.50719432716589));
#24644=CARTESIAN_POINT('Ctrl Pts',(-2.40469177216919,0.066705017937841,
-4.49886171111413));
#24645=CARTESIAN_POINT('Ctrl Pts',(-2.28597356220715,3.80875526597318,-2.3953266118554));
#24646=CARTESIAN_POINT('Ctrl Pts',(-2.16725535224511,4.08378985025871,1.88861502491571));
#24647=CARTESIAN_POINT('Ctrl Pts',(-2.04853714228307,0.641451595143002,
4.45339714207245));
#24648=CARTESIAN_POINT('Ctrl Pts',(-1.92981893232104,-3.38478417310792,
2.96436204859457));
#24649=CARTESIAN_POINT('Ctrl Pts',(-1.811100722359,-4.32993467155617,-1.22305845883667));
#24650=CARTESIAN_POINT('Ctrl Pts',(-1.69238251239696,-1.33365279105472,
-4.29715911814497));
#24651=CARTESIAN_POINT('Ctrl Pts',(-1.57366430243492,2.8766202213453,-3.45966217365956));
#24652=CARTESIAN_POINT('Ctrl Pts',(-1.45494609247288,4.46837703375138,0.527079631508651));
#24653=CARTESIAN_POINT('Ctrl Pts',(-1.33622788251084,1.99268081091691,4.03403389171687));
#24654=CARTESIAN_POINT('Ctrl Pts',(-1.2175096725488,-2.29690344137737,3.86890693021935));
#24655=CARTESIAN_POINT('Ctrl Pts',(-1.09879146258676,-4.49567333227797,
0.182009733685751));
#24656=CARTESIAN_POINT('Ctrl Pts',(-0.980073252624724,-2.60214304288765,
-3.67056641924161));
#24657=CARTESIAN_POINT('Ctrl Pts',(-0.861355042662687,1.66005366341003,
-4.18191679595742));
#24658=CARTESIAN_POINT('Ctrl Pts',(-0.742636832700647,4.4111446011256,-0.886571802886027));
#24659=CARTESIAN_POINT('Ctrl Pts',(-0.623918622738608,3.1468797706921,3.2157975624285));
#24660=CARTESIAN_POINT('Ctrl Pts',(-0.50520041277657,-0.981911839411234,
4.3909059877588));
#24661=CARTESIAN_POINT('Ctrl Pts',(-0.38648220281453,-4.21689340139514,
1.56908135384443));
#24662=CARTESIAN_POINT('Ctrl Pts',(-0.267763992852492,-3.61334125522512,
-2.68103920653919));
#24663=CARTESIAN_POINT('Ctrl Pts',(-0.149045782890452,0.279346016498718,
-4.49067612468082));
#24664=CARTESIAN_POINT('Ctrl Pts',(-0.0303275729284138,3.91775152235812,
-2.21256169694153));
#24665=CARTESIAN_POINT('Ctrl Pts',(0.0883906370336246,3.98992476970996,
2.07959288942982));
#24666=CARTESIAN_POINT('Ctrl Pts',(0.207108846995664,0.430168237555651,
4.47874553207819));
#24667=CARTESIAN_POINT('Ctrl Pts',(0.325827056957703,-3.52115979590533,
2.80100695204636));
#24668=CARTESIAN_POINT('Ctrl Pts',(0.444545266919741,-4.26726320502384,
-1.42641894013007));
#24669=CARTESIAN_POINT('Ctrl Pts',(0.563263476881781,-1.12898252024285,
-4.35541097058569));
#24670=CARTESIAN_POINT('Ctrl Pts',(0.681981686843819,3.03698301387176,-3.31978017753683));
#24671=CARTESIAN_POINT('Ctrl Pts',(0.800699896805858,4.43845806644354,0.737764356779564));
#24672=CARTESIAN_POINT('Ctrl Pts',(0.919418106767898,1.79971457931152,4.12374025451722));
#24673=CARTESIAN_POINT('Ctrl Pts',(1.03813631672994,-2.47726455196977,3.75597744845015));
#24674=CARTESIAN_POINT('Ctrl Pts',(1.15685452669197,-4.49925106626794,-0.0307586800565765));
#24675=CARTESIAN_POINT('Ctrl Pts',(1.27557273665401,-2.42568067756187,-3.78949594329049));
#24676=CARTESIAN_POINT('Ctrl Pts',(1.39429094661605,1.85592680379598,-4.09874882771119));
#24677=CARTESIAN_POINT('Ctrl Pts',(1.51300915657809,4.44813004413594,-0.677012085687766));
#24678=CARTESIAN_POINT('Ctrl Pts',(1.63172736654013,2.9913105828304,3.36099200397128));
#24679=CARTESIAN_POINT('Ctrl Pts',(1.75044557650217,-1.18842487629314,4.33956824662543));
#24680=CARTESIAN_POINT('Ctrl Pts',(1.86916378646421,-4.2863665803859,1.36794290533745));
#24681=CARTESIAN_POINT('Ctrl Pts',(1.98788199642625,-3.48253486073682,-2.84888701030155));
#24682=CARTESIAN_POINT('Ctrl Pts',(2.10660020638828,0.491362160619126,-4.47244558165035));
#24683=CARTESIAN_POINT('Ctrl Pts',(2.22531841635033,4.01798436686502,-2.02484761928903));
#24684=CARTESIAN_POINT('Ctrl Pts',(2.34403662631236,3.88713483670319,2.26591902216312));
#24685=CARTESIAN_POINT('Ctrl Pts',(2.46275483627441,0.217922659316698,4.49407565226358));
#24686=CARTESIAN_POINT('Ctrl Pts',(2.58147304623644,-3.64965912193048,2.63138643065241));
#24687=CARTESIAN_POINT('Ctrl Pts',(2.70019125619848,-4.19504652231746,-1.62658874006443));
#24688=CARTESIAN_POINT('Ctrl Pts',(2.81890946616052,-0.921786887931848,
-4.40392043376685));
#24689=CARTESIAN_POINT('Ctrl Pts',(2.93762767612256,3.19055253914903,-3.17247234009088));
#24690=CARTESIAN_POINT('Ctrl Pts',(3.0563458860846,4.39861094620036,0.946798815841214));
#24691=CARTESIAN_POINT('Ctrl Pts',(3.17506409604663,1.60272266101169,4.20422244007044));
#24692=CARTESIAN_POINT('Ctrl Pts',(3.29378230600868,-2.65208440004178,3.63464641867228));
#24693=CARTESIAN_POINT('Ctrl Pts',(3.41250051597071,-4.49276466266545,-0.243458291328418));
#24694=CARTESIAN_POINT('Ctrl Pts',(3.53121872593276,-2.24379243496572,-3.89994894357639));
#24695=CARTESIAN_POINT('Ctrl Pts',(3.64993693589478,2.04764851932484,-4.00641258422282));
#24696=CARTESIAN_POINT('Ctrl Pts',(3.76865514585684,4.47516569947413,-0.465937995834673));
#24697=CARTESIAN_POINT('Ctrl Pts',(3.88737335581886,2.8290502899728,3.49866841963007));
#24698=CARTESIAN_POINT('Ctrl Pts',(4.00609156578091,-1.39227958820118,4.27852355398336));
#24699=CARTESIAN_POINT('Ctrl Pts',(4.12480977574294,-4.34625181187136,1.16374457743831));
#24700=CARTESIAN_POINT('Ctrl Pts',(4.24352798570499,-3.34393856755371,-3.01036228885148));
#24701=CARTESIAN_POINT('Ctrl Pts',(4.36224619566702,0.702279202618052,-4.44421086080332));
#24702=CARTESIAN_POINT('Ctrl Pts',(4.48096440562906,4.10922959389586,-1.83260426670965));
#24703=CARTESIAN_POINT('Ctrl Pts',(4.5996826155911,3.77564997663844,2.44717664005326));
#24704=CARTESIAN_POINT('Ctrl Pts',(4.71840082555314,0.0051896213660362,
4.49935321146743));
#24705=CARTESIAN_POINT('Ctrl Pts',(4.83711903551518,-3.76999471780869,2.45587989962999));
#24706=CARTESIAN_POINT('Ctrl Pts',(4.95583724547722,-4.11344616113095,-1.82312010936994));
#24707=CARTESIAN_POINT('Ctrl Pts',(5.07455545543925,-0.712529359110903,
-4.44257899942333));
#24708=CARTESIAN_POINT('Ctrl Pts',(5.1932736654013,3.33698528559868,-3.0180681664618));
#24709=CARTESIAN_POINT('Ctrl Pts',(5.31199187536333,4.34892480494547,1.15371543052956));
#24710=CARTESIAN_POINT('Ctrl Pts',(5.43071008532538,1.40214569685748,4.27530042201669));
#24711=CARTESIAN_POINT('Ctrl Pts',(5.54942829528741,-2.82097194028839,3.50518523987218));
#24712=CARTESIAN_POINT('Ctrl Pts',(5.66814650524945,-4.47622863056497,-0.455613323578985));
#24713=CARTESIAN_POINT('Ctrl Pts',(5.78686471521149,-2.05688517132322,-4.00167835360398));
#24714=CARTESIAN_POINT('Ctrl Pts',(5.90558292517353,2.23478995779516,-3.90511460756914));
#24715=CARTESIAN_POINT('Ctrl Pts',(6.02430113513557,4.49219109250754,-0.253821673834409));
#24716=CARTESIAN_POINT('Ctrl Pts',(6.1430193450976,2.66046184361709,3.62851884828642));
#24717=CARTESIAN_POINT('Ctrl Pts',(6.26173755505965,-1.59301998327376,4.20790845748841));
#24718=CARTESIAN_POINT('Ctrl Pts',(6.38045576502168,-4.39641514173326,0.956943130625105));
#24719=CARTESIAN_POINT('Ctrl Pts',(6.49917397498372,-3.19786239441975,-3.16510384664836));
#24720=CARTESIAN_POINT('Ctrl Pts',(6.61789218494576,0.911625353279838,-4.4060351188988));
#24721=CARTESIAN_POINT('Ctrl Pts',(6.73661039490781,4.19128310181113,-1.63626165822722));
#24722=CARTESIAN_POINT('Ctrl Pts',(6.85532860486984,3.65571956412372,2.62296029748738));
#24723=CARTESIAN_POINT('Ctrl Pts',(6.97404681483188,-0.207555024975147,
4.49456640459564));
#24724=CARTESIAN_POINT('Ctrl Pts',(7.09276502479392,-3.88189741118738,2.27487994028893));
#24725=CARTESIAN_POINT('Ctrl Pts',(7.21148323475596,-4.0226446490118,-2.01557343738419));
#24726=CARTESIAN_POINT('Ctrl Pts',(7.330201444718,-0.501678010917997,-4.47130019424702));
#24727=CARTESIAN_POINT('Ctrl Pts',(7.44891965468003,3.47595370552743,-2.85691303520817));
#24728=CARTESIAN_POINT('Ctrl Pts',(7.56763786464208,4.28951078298972,1.35805135997396));
#24729=CARTESIAN_POINT('Ctrl Pts',(7.68635607460411,1.19843234688926,4.33681520976413));
#24730=CARTESIAN_POINT('Ctrl Pts',(7.80507428456615,-2.9835493970715,3.36788349693785));
#24731=CARTESIAN_POINT('Ctrl Pts',(7.92379249452818,-4.44967995854515,-0.666749218397577));
#24732=CARTESIAN_POINT('Ctrl Pts',(8.04251070449024,-1.86537696964218,-4.09445662021724));
#24733=CARTESIAN_POINT('Ctrl Pts',(8.16122891445226,2.41693251238594,-3.79508148585558));
#24734=CARTESIAN_POINT('Ctrl Pts',(8.27994712441432,4.49916814003176,-0.0411375915087343));
#24735=CARTESIAN_POINT('Ctrl Pts',(8.39866533437633,2.48592235037398,3.75025283435974));
#24736=CARTESIAN_POINT('Ctrl Pts',(8.51738354433839,-1.79019703590043,4.12788091232845));
#24737=CARTESIAN_POINT('Ctrl Pts',(8.63610175430042,-4.43674436226274,0.748001148155393));
#24738=CARTESIAN_POINT('Ctrl Pts',(8.75481996426246,-3.04463309142816,-3.31276555045668));
#24739=CARTESIAN_POINT('Ctrl Pts',(8.8735381742245,1.11893233723297,-4.35800374924192));
#24740=CARTESIAN_POINT('Ctrl Pts',(8.99225638418654,4.26396134944328,-1.43625898227515));
#24741=CARTESIAN_POINT('Ctrl Pts',(9.11097459414858,3.52761186517828,2.7928767932663));
#24742=CARTESIAN_POINT('Ctrl Pts',(9.22969280411062,-0.419835402419459,
4.47972593900423));
#24743=CARTESIAN_POINT('Ctrl Pts',(9.34841101407265,-3.98511689282915,2.08879142189926));
#24744=CARTESIAN_POINT('Ctrl Pts',(9.46712922403471,-3.92284509507712,-2.20351823540029));
#24745=CARTESIAN_POINT('Ctrl Pts',(9.58584743399672,-0.289704485621651,
-4.49001977331088));
#24746=CARTESIAN_POINT('Ctrl Pts',(9.70456564395878,3.60714694780058,-2.68936742574997));
#24747=CARTESIAN_POINT('Ctrl Pts',(9.82328385392081,4.22050178042756,1.55934953590272));
#24748=CARTESIAN_POINT('Ctrl Pts',(9.94200206388286,0.992038286763637,4.38862920412596));
#24749=CARTESIAN_POINT('Ctrl Pts',(10.0607202738449,-3.13945310944617,3.22304831290207));
#24750=CARTESIAN_POINT('Ctrl Pts',(10.1794384838069,-4.4131780319313,-0.876393697028316));
#24751=CARTESIAN_POINT('Ctrl Pts',(10.298156693769,-1.66969620452611,-4.17807621260108));
#24752=CARTESIAN_POINT('Ctrl Pts',(10.416874903731,2.59366875801597,-3.67655934637329));
#24753=CARTESIAN_POINT('Ctrl Pts',(10.5355931136931,4.49608123545688,0.171638509327548));
#24754=CARTESIAN_POINT('Ctrl Pts',(10.6543113236551,2.30582222843748,3.86359807751195));
#24755=CARTESIAN_POINT('Ctrl Pts',(10.7730295336171,-1.9833696911239,4.03861992790211));
#24756=CARTESIAN_POINT('Ctrl Pts',(10.8917477435792,-4.46714926315148,0.537386001337347));
#24757=CARTESIAN_POINT('Ctrl Pts',(11.0104659535412,-2.88459340913202,-3.45301710359151));
#24758=CARTESIAN_POINT('Ctrl Pts',(11.1291841635032,1.32373644041171,-4.30022419067547));
#24759=CARTESIAN_POINT('Ctrl Pts',(11.2479023734653,4.3271017666481,-1.23304361429234));
#24760=CARTESIAN_POINT('Ctrl Pts',(11.3666205834273,3.39161343716686,2.95654605012316));
#24761=CARTESIAN_POINT('Ctrl Pts',(11.4853387933893,-0.631176672186531,
4.45486501057192));
#24762=CARTESIAN_POINT('Ctrl Pts',(11.6040570033514,-4.07942227649942,1.8980305960162));
#24763=CARTESIAN_POINT('Ctrl Pts',(11.7227752133134,-3.81427073571983,-2.38653409952016));
#24764=CARTESIAN_POINT('Ctrl Pts',(11.8414934232755,-0.0770829355716051,
-4.49869586393552));
#24765=CARTESIAN_POINT('Ctrl Pts',(11.9602116332375,3.73027155305882,-2.5158061117259));
#24766=CARTESIAN_POINT('Ctrl Pts',(12.0789298431996,4.14205216006884,1.75715968445449));
#24767=CARTESIAN_POINT('Ctrl Pts',(12.1976480531616,0.783425188079069,4.43062650621253));
#24768=CARTESIAN_POINT('Ctrl Pts',(12.3163662631236,-3.28833434385892,3.07100365985594));
#24769=CARTESIAN_POINT('Ctrl Pts',(12.4350844730857,-4.36680450139639,-1.08407781279347));
#24770=CARTESIAN_POINT('Ctrl Pts',(12.5538026830477,-1.47028058123278,-4.2523500940886));
#24771=CARTESIAN_POINT('Ctrl Pts',(12.6725208930097,2.76460335749394,-3.54981329061017));
#24772=CARTESIAN_POINT('Ctrl Pts',(12.7912391029718,4.48293729360237,0.38403065356625));
#24773=CARTESIAN_POINT('Ctrl Pts',(12.9099573129338,2.1205643154784,3.96830109397022));
#24774=CARTESIAN_POINT('Ctrl Pts',(13.0286755228959,-2.17210581545682,3.94032506807154));
#24775=CARTESIAN_POINT('Ctrl Pts',(13.1473937328579,-4.48756190128028,0.325568993002829));
#24776=CARTESIAN_POINT('Ctrl Pts',(13.2661119428199,-2.71810120253451,-3.5855451440222));
#24777=CARTESIAN_POINT('Ctrl Pts',(13.384830152782,1.52557930134958,-4.23282500395937));
#24778=CARTESIAN_POINT('Ctrl Pts',(13.503548362744,4.38056358573491,-1.02707141553694));
#24779=CARTESIAN_POINT('Ctrl Pts',(13.6222665727061,3.2480275981586,3.1136044363927));
#24780=CARTESIAN_POINT('Ctrl Pts',(13.7409847826681,-0.841104404156636,
4.42003452904562));
#24781=CARTESIAN_POINT('Ctrl Pts',(13.8597029926301,-4.16460583332365,1.70303310482458));
#24782=CARTESIAN_POINT('Ctrl Pts',(13.9784212025922,-3.69715831531401,-2.5642286524609));
#24783=CARTESIAN_POINT('Ctrl Pts',(14.0971394125542,0.135699398207657,-4.49727672524931));
#24784=CARTESIAN_POINT('Ctrl Pts',(14.2158576225163,3.84507424612486,-2.33667881727876));
#24785=CARTESIAN_POINT('Ctrl Pts',(14.3345758324783,4.05429530274018,1.95115628770095));
#24786=CARTESIAN_POINT('Ctrl Pts',(14.4532940424403,0.57313975391872,4.46249073811889));
#24787=CARTESIAN_POINT('Ctrl Pts',(14.5720122524024,-3.43001236580562,2.91251275955532));
#24788=CARTESIAN_POINT('Ctrl Pts',(14.6907304623644,-4.31037334346474,-1.29014241853049));
#24789=CARTESIAN_POINT('Ctrl Pts',(14.8094486723265,-1.26812827461363,-4.31557435492763));
#24790=CARTESIAN_POINT('Ctrl Pts',(14.9281668822885,2.93041296965033,-3.41810294391185));
#24791=CARTESIAN_POINT('Ctrl Pts',(15.0468850922505,4.45767341533165,0.60166344454607));
#24792=CARTESIAN_POINT('Ctrl Pts',(15.1260305655585,2.77612598509681,2.89993003832736));
#24793=CARTESIAN_POINT('Ctrl Pts',(15.1656033022126,1.6350275666191,3.44198056308768));
#24794=CARTESIAN_POINT('Ctrl Pts',(-5.646,-1.68832072772979,3.57542852261347));
#24795=CARTESIAN_POINT('Ctrl Pts',(-5.60642726334599,-2.87366031862924,
3.01571004745528));
#24796=CARTESIAN_POINT('Ctrl Pts',(-5.52728179003796,-4.62399175064742,
0.634976333003133));
#24797=CARTESIAN_POINT('Ctrl Pts',(-5.40856358007592,-3.04887682921773,
-3.53972424598284));
#24798=CARTESIAN_POINT('Ctrl Pts',(-5.28984537011389,1.30552260182238,-4.48102060681164));
#24799=CARTESIAN_POINT('Ctrl Pts',(-5.17112716015184,4.4695002639332,-1.34901269686395));
#24800=CARTESIAN_POINT('Ctrl Pts',(-5.0524089501898,3.56606776773373,3.01391099447878));
#24801=CARTESIAN_POINT('Ctrl Pts',(-4.93369074022777,-0.584027462773018,
4.63180243166073));
#24802=CARTESIAN_POINT('Ctrl Pts',(-4.81497253026573,-4.20220283851478,
2.03428996774588));
#24803=CARTESIAN_POINT('Ctrl Pts',(-4.69625432030369,-3.9953715966269,-2.41541280931804));
#24804=CARTESIAN_POINT('Ctrl Pts',(-4.57753611034165,-0.151571156826602,
-4.66620083123102));
#24805=CARTESIAN_POINT('Ctrl Pts',(-4.45881790037962,3.83015800478312,-2.66957962108678));
#24806=CARTESIAN_POINT('Ctrl Pts',(-4.34009969041757,4.32541159811552,1.75715585210948));
#24807=CARTESIAN_POINT('Ctrl Pts',(-4.22138148045554,0.883338234818426,
4.5843632385526));
#24808=CARTESIAN_POINT('Ctrl Pts',(-4.10266327049349,-3.36280984898184,
3.23855535842678));
#24809=CARTESIAN_POINT('Ctrl Pts',(-3.98394506053146,-4.54787861419652,
-1.05523833281009));
#24810=CARTESIAN_POINT('Ctrl Pts',(-3.86522685056942,-1.59312430471214,
-4.38846994471302));
#24811=CARTESIAN_POINT('Ctrl Pts',(-3.74650864060738,2.81181073099031,-3.72698845879762));
#24812=CARTESIAN_POINT('Ctrl Pts',(-3.62779043064534,4.65722451696751,0.327079699827401));
#24813=CARTESIAN_POINT('Ctrl Pts',(-3.5090722206833,2.26328182735134,4.08341461302567));
#24814=CARTESIAN_POINT('Ctrl Pts',(-3.39035401072126,-2.1908701691093,4.12271861815529));
#24815=CARTESIAN_POINT('Ctrl Pts',(-3.27163580075922,-4.65072733698027,
0.409213699320028));
#24816=CARTESIAN_POINT('Ctrl Pts',(-3.15291759079718,-2.87714246487953,
-3.67678822308255));
#24817=CARTESIAN_POINT('Ctrl Pts',(-3.03419938083514,1.51543397348639,-4.41590086786405));
#24818=CARTESIAN_POINT('Ctrl Pts',(-2.91548117087311,4.52854837815398,-1.13532820490054));
#24819=CARTESIAN_POINT('Ctrl Pts',(-2.79676296091107,3.41943725654743,3.17870561254643));
#24820=CARTESIAN_POINT('Ctrl Pts',(-2.67804475094903,-0.802302976368572,
4.59924238172985));
#24821=CARTESIAN_POINT('Ctrl Pts',(-2.55932654098699,-4.2937266658855,1.83320262389659));
#24822=CARTESIAN_POINT('Ctrl Pts',(-2.44060833102495,-3.87667722720249,
-2.6015561142294));
#24823=CARTESIAN_POINT('Ctrl Pts',(-2.32189012106291,0.0692155551668676,
-4.6681827031938));
#24824=CARTESIAN_POINT('Ctrl Pts',(-2.20317191110087,3.95210313075198,-2.48547810001344));
#24825=CARTESIAN_POINT('Ctrl Pts',(-2.08445370113884,4.23748902869366,1.95969570936649));
#24826=CARTESIAN_POINT('Ctrl Pts',(-1.96573549117679,0.665593528688616,
4.62100701111058));
#24827=CARTESIAN_POINT('Ctrl Pts',(-1.84701728121476,-3.51217528912075,
3.07592998626008));
#24828=CARTESIAN_POINT('Ctrl Pts',(-1.72829907125272,-4.49289785675852,
-1.26908998523592));
#24829=CARTESIAN_POINT('Ctrl Pts',(-1.60958086129068,-1.38384669079458,
-4.45888874926723));
#24830=CARTESIAN_POINT('Ctrl Pts',(-1.49086265132864,2.98488587185672,-3.58987142860451));
#24831=CARTESIAN_POINT('Ctrl Pts',(-1.3721444413666,4.63655069209516,0.546917015238768));
#24832=CARTESIAN_POINT('Ctrl Pts',(-1.25342623140456,2.06767815768332,4.18586043462686));
#24833=CARTESIAN_POINT('Ctrl Pts',(-1.13470802144252,-2.38335063499626,
4.01451868753794));
#24834=CARTESIAN_POINT('Ctrl Pts',(-1.01598981148048,-4.66487432523292,
0.188859926168807));
#24835=CARTESIAN_POINT('Ctrl Pts',(-0.897271601518447,-2.70007835849569,
-3.80871335229026));
#24836=CARTESIAN_POINT('Ctrl Pts',(-0.778553391556407,1.72253211934917,
-4.33930912009507));
#24837=CARTESIAN_POINT('Ctrl Pts',(-0.659835181594369,4.57716423632007,
-0.919939180425913));
#24838=CARTESIAN_POINT('Ctrl Pts',(-0.541116971632329,3.26531701969948,
3.33682862952102));
#24839=CARTESIAN_POINT('Ctrl Pts',(-0.422398761670291,-1.01886747340488,
4.5561639142559));
#24840=CARTESIAN_POINT('Ctrl Pts',(-0.303680551708251,-4.37560211930362,
1.62813593888096));
#24841=CARTESIAN_POINT('Ctrl Pts',(-0.184962341746213,-3.74933443868876,
-2.78194389030271));
#24842=CARTESIAN_POINT('Ctrl Pts',(-0.0662441317841735,0.289859596974037,
-4.6596890406949));
#24843=CARTESIAN_POINT('Ctrl Pts',(0.0524740781778654,4.06520161464448,
-2.29583457030816));
#24844=CARTESIAN_POINT('Ctrl Pts',(0.171192288139903,4.14009120373516,2.1578612945889));
#24845=CARTESIAN_POINT('Ctrl Pts',(0.289910498101944,0.446358224583725,
4.64730942344886));
#24846=CARTESIAN_POINT('Ctrl Pts',(0.40862870806398,-3.65368360041369,2.90642679075152));
#24847=CARTESIAN_POINT('Ctrl Pts',(0.527346918026022,-4.42786766138104,
-1.4801042244471));
#24848=CARTESIAN_POINT('Ctrl Pts',(0.646065127988058,-1.17147336629305,
-4.51933299215671));
#24849=CARTESIAN_POINT('Ctrl Pts',(0.764783337950099,3.15128414377037,-3.44472477669139));
#24850=CARTESIAN_POINT('Ctrl Pts',(0.883501547912136,4.60550568234552,0.765531156657499));
#24851=CARTESIAN_POINT('Ctrl Pts',(1.00221975787418,1.86744937037575,4.27894302264161));
#24852=CARTESIAN_POINT('Ctrl Pts',(1.12093796783621,-2.57049988982138,3.89733894578832));
#24853=CARTESIAN_POINT('Ctrl Pts',(1.23965617779826,-4.6685867122768,-0.0319163262694973));
#24854=CARTESIAN_POINT('Ctrl Pts',(1.35837438776029,-2.5169745837023,-3.93211895635505));
#24855=CARTESIAN_POINT('Ctrl Pts',(1.47709259772233,1.92577722104035,-4.25301100831545));
#24856=CARTESIAN_POINT('Ctrl Pts',(1.59581080768437,4.61554167853046,-0.70249238834195));
#24857=CARTESIAN_POINT('Ctrl Pts',(1.71452901764641,3.10389276650854,3.48748766821418));
#24858=CARTESIAN_POINT('Ctrl Pts',(1.83324722760845,-1.23315291907095,4.50289400498357));
#24859=CARTESIAN_POINT('Ctrl Pts',(1.95196543757049,-4.44769001916047,1.41942736178737));
#24860=CARTESIAN_POINT('Ctrl Pts',(2.07068364753253,-3.61360496145035,-2.95610888238434));
#24861=CARTESIAN_POINT('Ctrl Pts',(2.18940185749457,0.509855267064465,-4.64077236552028));
#24862=CARTESIAN_POINT('Ctrl Pts',(2.3081200674566,4.16920686331953,-2.10105560915926));
#24863=CARTESIAN_POINT('Ctrl Pts',(2.42683827741864,4.03343262693579,2.35120007355821));
#24864=CARTESIAN_POINT('Ctrl Pts',(2.54555648738068,0.226124485298797,4.66321651428264));
#24865=CARTESIAN_POINT('Ctrl Pts',(2.66427469734272,-3.78701917942043,2.73042236231537));
#24866=CARTESIAN_POINT('Ctrl Pts',(2.78299290730476,-4.35293300218511,-1.6878076965158));
#24867=CARTESIAN_POINT('Ctrl Pts',(2.9017111172668,-0.956479634758229,-4.56966817725565));
#24868=CARTESIAN_POINT('Ctrl Pts',(3.02042932722884,3.31063347426123,-3.29187280146591));
#24869=CARTESIAN_POINT('Ctrl Pts',(3.13914753719087,4.56415885965217,0.982432921775639));
#24870=CARTESIAN_POINT('Ctrl Pts',(3.25786574715291,1.66304338398937,4.36245426851668));
#24871=CARTESIAN_POINT('Ctrl Pts',(3.37658395711496,-2.75189932891252,3.7714414519466));
#24872=CARTESIAN_POINT('Ctrl Pts',(3.49530216707699,-4.66185618374594,-0.252621186759496));
#24873=CARTESIAN_POINT('Ctrl Pts',(3.61402037703904,-2.32824072111122,-4.04672901075542));
#24874=CARTESIAN_POINT('Ctrl Pts',(3.73273858700106,2.12471465315734,-4.15719956035174));
#24875=CARTESIAN_POINT('Ctrl Pts',(3.85145679696312,4.64359485880658,-0.483474228057011));
#24876=CARTESIAN_POINT('Ctrl Pts',(3.97017500692514,2.93552557916831,3.63034572953853));
#24877=CARTESIAN_POINT('Ctrl Pts',(4.08889321688719,-1.44467998996152,4.43955180942118));
#24878=CARTESIAN_POINT('Ctrl Pts',(4.20761142684922,-4.50982911561381,1.20754374243428));
#24879=CARTESIAN_POINT('Ctrl Pts',(4.32632963681127,-3.46979240171644,-3.12366151029863));
#24880=CARTESIAN_POINT('Ctrl Pts',(4.4450478467733,0.728710468778227,-4.61147499121735));
#24881=CARTESIAN_POINT('Ctrl Pts',(4.56376605673534,4.26388623288585,-1.90157690744722));
#24882=CARTESIAN_POINT('Ctrl Pts',(4.68248426669738,3.91775187726159,2.53927957699493));
#24883=CARTESIAN_POINT('Ctrl Pts',(4.80120247665942,0.00538494006987035,
4.66869270185463));
#24884=CARTESIAN_POINT('Ctrl Pts',(4.91992068662146,-3.91188377480672,2.54831039599456));
#24885=CARTESIAN_POINT('Ctrl Pts',(5.03863889658349,-4.2682614965631,-1.8917358004983));
#24886=CARTESIAN_POINT('Ctrl Pts',(5.15735710654554,-0.739346404336463,
-4.60978171243769));
#24887=CARTESIAN_POINT('Ctrl Pts',(5.27607531650758,3.46257742320919,-3.13165740945785));
#24888=CARTESIAN_POINT('Ctrl Pts',(5.39479352646961,4.51260271054416,1.19713713446688));
#24889=CARTESIAN_POINT('Ctrl Pts',(5.51351173643165,1.45491742350237,4.4362073703468));
#24890=CARTESIAN_POINT('Ctrl Pts',(5.63222994639369,-2.92714318942428,3.63710781948203));
#24891=CARTESIAN_POINT('Ctrl Pts',(5.75094815635573,-4.64469779480496,-0.47276097223033));
#24892=CARTESIAN_POINT('Ctrl Pts',(5.86966636631777,-2.13429893955308,-4.15228715030074));
#24893=CARTESIAN_POINT('Ctrl Pts',(5.98838457627981,2.31889942304252,-4.05208909178254));
#24894=CARTESIAN_POINT('Ctrl Pts',(6.10710278624184,4.6612610264679,-0.263374609751229));
#24895=CARTESIAN_POINT('Ctrl Pts',(6.2258209962039,2.76059206936697,3.76508326182549));
#24896=CARTESIAN_POINT('Ctrl Pts',(6.34453920616592,-1.65297553231951,4.36627901438777));
#24897=CARTESIAN_POINT('Ctrl Pts',(6.46325741612797,-4.56188041299363,0.992959032123235));
#24898=CARTESIAN_POINT('Ctrl Pts',(6.58197562609,-3.31821844622275,-3.28422698440246));
#24899=CARTESIAN_POINT('Ctrl Pts',(6.70069383605205,0.945935656448541,-4.57186245153871));
#24900=CARTESIAN_POINT('Ctrl Pts',(6.81941204601407,4.34902794005149,-1.69784466856703));
#24901=CARTESIAN_POINT('Ctrl Pts',(6.93813025597612,3.7933077148849,2.72167909976998));
#24902=CARTESIAN_POINT('Ctrl Pts',(7.05684846593816,-0.215366650447688,
4.66372573676938));
#24903=CARTESIAN_POINT('Ctrl Pts',(7.1755666759002,-4.02799808353968,2.36049824844903));
#24904=CARTESIAN_POINT('Ctrl Pts',(7.29428488586223,-4.17404254174364,-2.09143238036622));
#24905=CARTESIAN_POINT('Ctrl Pts',(7.41300309582428,-0.520559368907565,
-4.63958386985003));
#24906=CARTESIAN_POINT('Ctrl Pts',(7.53172130578631,3.60677611520251,-2.96443697803392));
#24907=CARTESIAN_POINT('Ctrl Pts',(7.65043951574836,4.45095255825434,1.40916353419305));
#24908=CARTESIAN_POINT('Ctrl Pts',(7.76915772571038,1.24353703490719,4.50003735370544));
#24909=CARTESIAN_POINT('Ctrl Pts',(7.88787593567244,-3.09583947760073,3.49463853221744));
#24910=CARTESIAN_POINT('Ctrl Pts',(8.00659414563446,-4.61714992614977,-0.691843263597633));
#24911=CARTESIAN_POINT('Ctrl Pts',(8.12531235559652,-1.93558305717806,-4.24855725755173));
#24912=CARTESIAN_POINT('Ctrl Pts',(8.24403056555854,2.50789716901805,-3.93791471867551));
#24913=CARTESIAN_POINT('Ctrl Pts',(8.36274877552059,4.66850066499502,-0.0426858626611376));
#24914=CARTESIAN_POINT('Ctrl Pts',(8.48146698548262,2.57948353665327,3.89139887778996));
#24915=CARTESIAN_POINT('Ctrl Pts',(8.60018519544467,-1.85757362082367,4.28323951993702));
#24916=CARTESIAN_POINT('Ctrl Pts',(8.7189034054067,-4.60372748049605,0.776153224083728));
#24917=CARTESIAN_POINT('Ctrl Pts',(8.83762161536874,-3.15922214276211,-3.4374461442489));
#24918=CARTESIAN_POINT('Ctrl Pts',(8.95633982533078,1.16104493050125,-4.52202335368666));
#24919=CARTESIAN_POINT('Ctrl Pts',(9.07505803529283,4.42444153581877,-1.4903146104269));
#24920=CARTESIAN_POINT('Ctrl Pts',(9.19377624525485,3.66037850239417,2.89799064200363));
#24921=CARTESIAN_POINT('Ctrl Pts',(9.3124944552169,-0.435636498655038,4.64832672936936));
#24922=CARTESIAN_POINT('Ctrl Pts',(9.43121266517893,-4.13510237564149,2.16740602677358));
#24923=CARTESIAN_POINT('Ctrl Pts',(9.54993087514098,-4.07048689114132,-2.2864507453643));
#24924=CARTESIAN_POINT('Ctrl Pts',(9.66864908510301,-0.300607921660628,
-4.65900798661742));
#24925=CARTESIAN_POINT('Ctrl Pts',(9.78736729506505,3.74290699978661,-2.79058555376438));
#24926=CARTESIAN_POINT('Ctrl Pts',(9.90608550502709,4.37934630475926,1.61803785027473));
#24927=CARTESIAN_POINT('Ctrl Pts',(10.0248037149891,1.02937504385506,4.55380144066675));
#24928=CARTESIAN_POINT('Ctrl Pts',(10.1435219249512,-3.2576108456055,3.34435227219316));
#24929=CARTESIAN_POINT('Ctrl Pts',(10.2622401349132,-4.57927419815593,-0.909378007229871));
#24930=CARTESIAN_POINT('Ctrl Pts',(10.3809583448752,-1.73253757107079,-4.33532399097899));
#24931=CARTESIAN_POINT('Ctrl Pts',(10.4996765548373,2.69128513198641,-3.8149318316688));
#24932=CARTESIAN_POINT('Ctrl Pts',(10.6183947647993,4.66529758042202,0.178098366185712));
#24933=CARTESIAN_POINT('Ctrl Pts',(10.7371129747614,2.39260509315942,4.00901002868737));
#24934=CARTESIAN_POINT('Ctrl Pts',(10.8558311847234,-2.05801660079268,4.19061907273819));
#24935=CARTESIAN_POINT('Ctrl Pts',(10.9745493946854,-4.63527671262081,0.557611279800856));
#24936=CARTESIAN_POINT('Ctrl Pts',(11.0932676046475,-2.99315914178703,-3.58297626197237));
#24937=CARTESIAN_POINT('Ctrl Pts',(11.2119858146095,1.37355712433912,-4.46206918011612));
#24938=CARTESIAN_POINT('Ctrl Pts',(11.3307040245716,4.48995833148729,-1.27945094606998));
#24939=CARTESIAN_POINT('Ctrl Pts',(11.4494222345336,3.51926158214387,3.06781982168619));
#24940=CARTESIAN_POINT('Ctrl Pts',(11.5681404444956,-0.654931894546049,
4.62253012490687));
#24941=CARTESIAN_POINT('Ctrl Pts',(11.6868586544577,-4.23295707514914,1.96946564873655));
#24942=CARTESIAN_POINT('Ctrl Pts',(11.8055768644197,-3.95782618296486,-2.47635466910213));
#24943=CARTESIAN_POINT('Ctrl Pts',(11.9242950743818,-0.0799840603363634,
-4.66801061412323));
#24944=CARTESIAN_POINT('Ctrl Pts',(12.0430132843438,3.87066557284614,-2.61049201542129));
#24945=CARTESIAN_POINT('Ctrl Pts',(12.1617314943058,4.29794412253036,1.82329286216014));
#24946=CARTESIAN_POINT('Ctrl Pts',(12.2804497042679,0.812910497604809,4.59737937032327));
#24947=CARTESIAN_POINT('Ctrl Pts',(12.3991679142299,-3.41209543480698,3.18658520464592));
#24948=CARTESIAN_POINT('Ctrl Pts',(12.5178861241919,-4.53115533453443,-1.12487860698111));
#24949=CARTESIAN_POINT('Ctrl Pts',(12.636604334154,-1.52561666014242,-4.41239327452744));
#24950=CARTESIAN_POINT('Ctrl Pts',(12.755322544116,2.86865309568467,-3.68341550971791));
#24951=CARTESIAN_POINT('Ctrl Pts',(12.8740407540781,4.65165894781738,0.398484187688063));
#24952=CARTESIAN_POINT('Ctrl Pts',(12.9927589640401,2.20037473791892,4.11765369052636));
#24953=CARTESIAN_POINT('Ctrl Pts',(13.1114771740021,-2.25385607478723,4.08862474752024));
#24954=CARTESIAN_POINT('Ctrl Pts',(13.2301953839642,-4.6564576091138,0.337822240251874));
#24955=CARTESIAN_POINT('Ctrl Pts',(13.3489135939262,-2.82040076667739,-3.72049218172121));
#24956=CARTESIAN_POINT('Ctrl Pts',(13.4676318038883,1.58299662541684,-4.39213333015208));
#24957=CARTESIAN_POINT('Ctrl Pts',(13.5863500138503,4.54543226137621,-1.06572669373447));
#24958=CARTESIAN_POINT('Ctrl Pts',(13.7050682238123,3.37027168800554,3.2307893213629));
#24959=CARTESIAN_POINT('Ctrl Pts',(13.8237864337744,-0.872760552155723,
4.58638874918879));
#24960=CARTESIAN_POINT('Ctrl Pts',(13.9425046437364,-4.32134663501959,1.76712915252949));
#24961=CARTESIAN_POINT('Ctrl Pts',(14.0612228536984,-3.83630607179607,-2.66073700662553));
#24962=CARTESIAN_POINT('Ctrl Pts',(14.1799410636605,0.140806636039052,-4.6665380641553));
#24963=CARTESIAN_POINT('Ctrl Pts',(14.2986592736225,3.98978902683606,-2.42462301314851));
#24964=CARTESIAN_POINT('Ctrl Pts',(14.4173774835846,4.20688441236941,2.0245908005956));
#24965=CARTESIAN_POINT('Ctrl Pts',(14.5360956935466,0.594710675179534,4.63044285744233));
#24966=CARTESIAN_POINT('Ctrl Pts',(14.6548139035086,-3.55910570850363,3.02212927625648));
#24967=CARTESIAN_POINT('Ctrl Pts',(14.7735321134707,-4.47260031055426,-1.33869874416505));
#24968=CARTESIAN_POINT('Ctrl Pts',(14.8922503234327,-1.31585606695972,-4.47799706940333));
#24969=CARTESIAN_POINT('Ctrl Pts',(15.0109685333948,3.04070318595074,-3.54674805875586));
#24970=CARTESIAN_POINT('Ctrl Pts',(15.1296867433568,4.62544422793221,0.624307895047183));
#24971=CARTESIAN_POINT('Ctrl Pts',(15.2088322166648,2.880609393594,3.00907298660654));
#24972=CARTESIAN_POINT('Ctrl Pts',(15.2484049533188,1.69656413018441,3.57152434573413));
#24973=CARTESIAN_POINT('Ctrl Pts',(14.7388401553692,-3.95165589089271,-0.00363582964324092));
#24974=CARTESIAN_POINT('Ctrl Pts',(14.7504041414031,-3.95480700531195,-0.38716052775308));
#24975=CARTESIAN_POINT('Ctrl Pts',(14.7619681274369,-3.90348129134194,-0.769828015324074));
#24976=CARTESIAN_POINT('Ctrl Pts',(14.7735321134707,-3.79422716961339,-1.13511046163454));
#24977=CARTESIAN_POINT('Ctrl Pts',(14.8131048501247,-3.42035222935605,-2.38513151924453));
#24978=CARTESIAN_POINT('Ctrl Pts',(14.8526775867787,-2.36810414815783,-3.43156429432397));
#24979=CARTESIAN_POINT('Ctrl Pts',(14.8922503234327,-1.11588689874029,-3.79957251342241));
#24980=CARTESIAN_POINT('Ctrl Pts',(14.9281668822885,0.0206363326986077,
-4.13357996345584));
#24981=CARTESIAN_POINT('Ctrl Pts',(14.9640834411442,1.32188486567401,-3.90873281330822));
#24982=CARTESIAN_POINT('Ctrl Pts',(15.,2.29296287427331,-3.22854765929654));
#24983=CARTESIAN_POINT('',(-5.646,-2.04569608541847,-2.86913603522098));
#24984=CARTESIAN_POINT('Ctrl Pts',(-5.646,-2.05008858489997,-2.8725153718199));
#24985=CARTESIAN_POINT('Ctrl Pts',(-5.646,-2.14207707493584,-2.81555118308838));
#24986=CARTESIAN_POINT('Ctrl Pts',(-5.646,-2.23107770091101,-2.7542618031163));
#24987=CARTESIAN_POINT('Ctrl Pts',(-5.646,-2.31673031453871,-2.68871061623223));
#24988=CARTESIAN_POINT('Ctrl Pts',(-5.646,-2.4049668623091,-2.6211819070904));
#24989=CARTESIAN_POINT('Ctrl Pts',(-5.646,-2.48965143582115,-2.54913073294227));
#24990=CARTESIAN_POINT('Ctrl Pts',(-5.646,-2.57069342680521,-2.47296330102159));
#24991=CARTESIAN_POINT('Ctrl Pts',(-5.646,-2.62057798544578,-2.42607922675328));
#24992=CARTESIAN_POINT('Ctrl Pts',(-5.646,-2.66908188885062,-2.37763460603863));
#24993=CARTESIAN_POINT('Ctrl Pts',(-5.646,-2.71617833586228,-2.32771640428473));
#24994=CARTESIAN_POINT('Ctrl Pts',(-5.646,-2.73123404318985,-2.31175864348508));
#24995=CARTESIAN_POINT('Ctrl Pts',(-5.646,-2.74614588109029,-2.29565025093888));
#24996=CARTESIAN_POINT('Ctrl Pts',(-5.646,-2.76091287095153,-2.27939395874847));
#24997=CARTESIAN_POINT('Ctrl Pts',(-5.646,-2.77497190065622,-2.26391702696071));
#24998=CARTESIAN_POINT('Ctrl Pts',(-5.646,-2.78889460108938,-2.24831151965524));
#24999=CARTESIAN_POINT('Ctrl Pts',(-5.646,-2.80267583839923,-2.2325853908502));
#25000=CARTESIAN_POINT('Ctrl Pts',(-5.646,-2.87737822131438,-2.14734055619902));
#25001=CARTESIAN_POINT('Ctrl Pts',(-5.646,-2.94796949551254,-2.05850773745867));
#25002=CARTESIAN_POINT('Ctrl Pts',(-5.646,-3.01435939466491,-1.96650898761472));
#25003=CARTESIAN_POINT('Ctrl Pts',(-5.646,-3.07837534811936,-1.87779989537221));
#25004=CARTESIAN_POINT('Ctrl Pts',(-5.646,-3.13848514835476,-1.78614641339449));
#25005=CARTESIAN_POINT('Ctrl Pts',(-5.646,-3.19457903134324,-1.69189377245409));
#25006=CARTESIAN_POINT('Ctrl Pts',(-5.646,-3.2191201051507,-1.65065824204266));
#25007=CARTESIAN_POINT('Ctrl Pts',(-5.646,-3.24289211518763,-1.60892485034322));
#25008=CARTESIAN_POINT('Ctrl Pts',(-5.646,-3.26588393940166,-1.56672099319786));
#25009=CARTESIAN_POINT('Ctrl Pts',(-5.646,-3.27889011824424,-1.54284681476081));
#25010=CARTESIAN_POINT('Ctrl Pts',(-5.646,-3.29164661390766,-1.51882207153166));
#25011=CARTESIAN_POINT('Ctrl Pts',(-5.646,-3.30415123343052,-1.49465161725134));
#25012=CARTESIAN_POINT('Ctrl Pts',(-5.646,-3.31300408836539,-1.47753973911205));
#25013=CARTESIAN_POINT('Ctrl Pts',(-5.646,-3.32172655541921,-1.46036277478602));
#25014=CARTESIAN_POINT('Ctrl Pts',(-5.646,-3.3303159831105,-1.44312718454166));
#25015=CARTESIAN_POINT('Ctrl Pts',(-5.646,-3.38286439723767,-1.33768326366137));
#25016=CARTESIAN_POINT('Ctrl Pts',(-5.646,-3.43046401145348,-1.22999506945072));
#25017=CARTESIAN_POINT('Ctrl Pts',(-5.646,-3.473014032799,-1.12050081343609));
#25018=CARTESIAN_POINT('Ctrl Pts',(-5.646,-3.51603566968294,-1.00979294598551));
#25019=CARTESIAN_POINT('Ctrl Pts',(-5.646,-3.55389562836961,-0.897237988908388));
#25020=CARTESIAN_POINT('Ctrl Pts',(-5.646,-3.5864484949203,-0.783255416256629));
#25021=CARTESIAN_POINT('Ctrl Pts',(-5.646,-3.6186577594367,-0.670475952516229));
#25022=CARTESIAN_POINT('Ctrl Pts',(-5.646,-3.64567169970723,-0.556298001248345));
#25023=CARTESIAN_POINT('Ctrl Pts',(-5.646,-3.66730359446243,-0.441107587639058));
#25024=CARTESIAN_POINT('Ctrl Pts',(-5.646,-3.68198751655827,-0.362915312816758));
#25025=CARTESIAN_POINT('Ctrl Pts',(-5.646,-3.69419054645532,-0.284256101620809));
#25026=CARTESIAN_POINT('Ctrl Pts',(-5.646,-3.70384084236009,-0.205248270572724));
#25027=CARTESIAN_POINT('Ctrl Pts',(-5.646,-3.70640721713813,-0.184237131964063));
#25028=CARTESIAN_POINT('Ctrl Pts',(-5.646,-3.70879299259457,-0.163201334056653));
#25029=CARTESIAN_POINT('Ctrl Pts',(-5.646,-3.71099667802055,-0.142143098155404));
#25030=CARTESIAN_POINT('Ctrl Pts',(-5.646,-3.71270249148621,-0.125842485581626));
#25031=CARTESIAN_POINT('Ctrl Pts',(-5.646,-3.71429910512685,-0.109528708261293));
#25032=CARTESIAN_POINT('Ctrl Pts',(-5.646,-3.71578473600114,-0.0932167080416795));
#25033=CARTESIAN_POINT('Ctrl Pts',(-5.646,-3.72667009638022,0.0263028872816144));
#25034=CARTESIAN_POINT('Ctrl Pts',(-5.646,-3.73162164541571,0.145914627178937));
#25035=CARTESIAN_POINT('Ctrl Pts',(-5.646,-3.73049871915079,0.26519666316469));
#25036=CARTESIAN_POINT('Ctrl Pts',(-5.646,-3.72973942409088,0.345852235564089));
#25037=CARTESIAN_POINT('Ctrl Pts',(-5.646,-3.72620187382023,0.426357611138785));
#25038=CARTESIAN_POINT('Ctrl Pts',(-5.646,-3.71982963805668,0.506586333723297));
#25039=CARTESIAN_POINT('Ctrl Pts',(-5.646,-3.71064929233637,0.622170162909031));
#25040=CARTESIAN_POINT('Ctrl Pts',(-5.646,-3.69558794607162,0.7371801151484));
#25041=CARTESIAN_POINT('Ctrl Pts',(-5.646,-3.67492250378245,0.851326378345511));
#25042=CARTESIAN_POINT('Ctrl Pts',(-5.646,-3.65389180309679,0.967490158539211));
#25043=CARTESIAN_POINT('Ctrl Pts',(-5.646,-3.62705693335592,1.08276014959161));
#25044=CARTESIAN_POINT('Ctrl Pts',(-5.646,-3.59465621011333,1.19682455346059));
#25045=CARTESIAN_POINT('Ctrl Pts',(-5.646,-3.58656895937205,1.22529513505337));
#25046=CARTESIAN_POINT('Ctrl Pts',(-5.646,-3.57813470527536,1.25369054778353));
#25047=CARTESIAN_POINT('Ctrl Pts',(-5.646,-3.56935667185545,1.28200580159195));
#25048=CARTESIAN_POINT('Ctrl Pts',(-5.646,-3.5632475546913,1.30171194700898));
#25049=CARTESIAN_POINT('Ctrl Pts',(-5.646,-3.5569709708608,1.32138188327048));
#25050=CARTESIAN_POINT('Ctrl Pts',(-5.646,-3.55053584166857,1.34099072546513));
#25051=CARTESIAN_POINT('Ctrl Pts',(-5.646,-3.51190829019201,1.45869489870602));
#25052=CARTESIAN_POINT('Ctrl Pts',(-5.646,-3.46752131199915,1.57437189095583));
#25053=CARTESIAN_POINT('Ctrl Pts',(-5.646,-3.4177365460153,1.68768626856115));
#25054=CARTESIAN_POINT('Ctrl Pts',(-5.646,-3.36898689227503,1.79864464233047));
#25055=CARTESIAN_POINT('Ctrl Pts',(-5.646,-3.31506092584505,1.90733835387831));
#25056=CARTESIAN_POINT('Ctrl Pts',(-5.646,-3.25624215907454,2.01344625944578));
#25057=CARTESIAN_POINT('Ctrl Pts',(-5.646,-3.19710665592352,2.1201255512527));
#25058=CARTESIAN_POINT('Ctrl Pts',(-5.646,-3.13302512594978,2.22419187938599));
#25059=CARTESIAN_POINT('Ctrl Pts',(-5.646,-3.06423583750868,2.32530137231072));
#25060=CARTESIAN_POINT('Ctrl Pts',(-5.646,-3.02024766893345,2.38995709880711));
#25061=CARTESIAN_POINT('Ctrl Pts',(-5.646,-2.97433345310045,2.45340335435671));
#25062=CARTESIAN_POINT('Ctrl Pts',(-5.646,-2.92654602325611,2.515544268775));
#25063=CARTESIAN_POINT('Ctrl Pts',(-5.646,-2.9070747480676,2.54086395742628));
#25064=CARTESIAN_POINT('Ctrl Pts',(-5.646,-2.88729240115396,2.56596686978521));
#25065=CARTESIAN_POINT('Ctrl Pts',(-5.646,-2.86720223741143,2.59084624023121));
#25066=CARTESIAN_POINT('Ctrl Pts',(-5.646,-2.8548315572927,2.60616591294702));
#25067=CARTESIAN_POINT('Ctrl Pts',(-5.646,-2.84234310750814,2.62140196742225));
#25068=CARTESIAN_POINT('Ctrl Pts',(-5.646,-2.82975126313558,2.63653676106713));
#25069=CARTESIAN_POINT('Ctrl Pts',(-5.646,-2.75009555303069,2.73227910820889));
#25070=CARTESIAN_POINT('Ctrl Pts',(-5.646,-2.66618789926205,2.82411933161441));
#25071=CARTESIAN_POINT('Ctrl Pts',(-5.646,-2.57832047400345,2.91172962772101));
#25072=CARTESIAN_POINT('Ctrl Pts',(-5.646,-2.49061075100628,2.99918268305518));
#25073=CARTESIAN_POINT('Ctrl Pts',(-5.646,-2.39895497729817,3.0824217324784));
#25074=CARTESIAN_POINT('Ctrl Pts',(-5.646,-2.30359796366059,3.16109653178087));
#25075=CARTESIAN_POINT('Ctrl Pts',(-5.646,-2.20819311932976,3.23981079404521));
#25076=CARTESIAN_POINT('Ctrl Pts',(-5.646,-2.10908286731295,3.31395700277454));
#25077=CARTESIAN_POINT('Ctrl Pts',(-5.646,-2.00647347901961,3.38314868003774));
#25078=CARTESIAN_POINT('Ctrl Pts',(-5.646,-1.90386409072627,3.45234035730095));
#25079=CARTESIAN_POINT('Ctrl Pts',(-5.646,-1.79775511151038,3.51657830519508));
#25080=CARTESIAN_POINT('Ctrl Pts',(-5.646,-1.68832072772984,3.57542852261345));
#25081=CARTESIAN_POINT('Ctrl Pts',(-5.646,-2.05008858490001,-2.87251537181987));
#25082=CARTESIAN_POINT('Ctrl Pts',(-5.61008344114424,-1.18607795770181,
-3.48068169523233));
#25083=CARTESIAN_POINT('Ctrl Pts',(-5.53459414563446,1.25030204642021,-3.90746250366534));
#25084=CARTESIAN_POINT('Ctrl Pts',(-5.41953211347069,3.98315669070171,-1.20222141896168));
#25085=CARTESIAN_POINT('Ctrl Pts',(-5.30081390350864,3.17803017110567,2.68595570733295));
#25086=CARTESIAN_POINT('Ctrl Pts',(-5.18209569354661,-0.520477180563039,
4.12779813317261));
#25087=CARTESIAN_POINT('Ctrl Pts',(-5.08501265836025,-3.1573187910564,2.23479178678414));
#25088=CARTESIAN_POINT('Ctrl Pts',(-5.02750235982792,-3.51942846575801,
0.532373395398288));
#25089=CARTESIAN_POINT('Ctrl Pts',(-5.0095647979496,-3.51824182757685,0.000900848728238278));
#25090=CARTESIAN_POINT('Origin',(-5.646,-9.39637619619865E-16,-2.12715743287418E-16));
#25091=CARTESIAN_POINT('',(-5.646,-3.954,-4.84225344382864E-16));
#25092=CARTESIAN_POINT('Origin',(-5.646,0.,0.));
#25093=CARTESIAN_POINT('Origin',(-5.646,0.,0.));
#25094=CARTESIAN_POINT('',(-5.646,2.04569608541843,-2.86913603522101));
#25095=CARTESIAN_POINT('Ctrl Pts',(-5.646,1.69249901178079,3.58003443294051));
#25096=CARTESIAN_POINT('Ctrl Pts',(-5.646,1.79910683175878,3.52349759682845));
#25097=CARTESIAN_POINT('Ctrl Pts',(-5.646,1.90274240538976,3.46193012866522));
#25098=CARTESIAN_POINT('Ctrl Pts',(-5.646,2.00300255842392,3.3953141034615));
#25099=CARTESIAN_POINT('Ctrl Pts',(-5.646,2.10503185727917,3.32752260166971));
#25100=CARTESIAN_POINT('Ctrl Pts',(-5.646,2.20356614449629,3.25450231195095));
#25101=CARTESIAN_POINT('Ctrl Pts',(-5.646,2.29842061962347,3.17666297164194));
#25102=CARTESIAN_POINT('Ctrl Pts',(-5.646,2.35385455809869,3.13117285432428));
#25103=CARTESIAN_POINT('Ctrl Pts',(-5.646,2.40803103805464,3.08403610735246));
#25104=CARTESIAN_POINT('Ctrl Pts',(-5.646,2.46090694714461,3.03532931840981));
#25105=CARTESIAN_POINT('Ctrl Pts',(-5.646,2.48067509371497,3.0171198358806));
#25106=CARTESIAN_POINT('Ctrl Pts',(-5.646,2.50026140964636,2.99869087503606));
#25107=CARTESIAN_POINT('Ctrl Pts',(-5.646,2.51966346254713,2.98004633066214));
#25108=CARTESIAN_POINT('Ctrl Pts',(-5.646,2.5332676652907,2.96697327272226));
#25109=CARTESIAN_POINT('Ctrl Pts',(-5.646,2.54677877844966,2.95379656682823));
#25110=CARTESIAN_POINT('Ctrl Pts',(-5.646,2.5601903809623,2.94052341544533));
#25111=CARTESIAN_POINT('Ctrl Pts',(-5.646,2.64704277931223,2.85456761484802));
#25112=CARTESIAN_POINT('Ctrl Pts',(-5.646,2.72979795902533,2.76450027536008));
#25113=CARTESIAN_POINT('Ctrl Pts',(-5.646,2.80828101128637,2.67073206305303));
#25114=CARTESIAN_POINT('Ctrl Pts',(-5.646,2.88147991128195,2.58327713109399));
#25115=CARTESIAN_POINT('Ctrl Pts',(-5.646,2.95096248865815,2.49260198813964));
#25116=CARTESIAN_POINT('Ctrl Pts',(-5.646,3.01655400858887,2.39901735366309));
#25117=CARTESIAN_POINT('Ctrl Pts',(-5.646,3.04525029855856,2.35807407607961));
#25118=CARTESIAN_POINT('Ctrl Pts',(-5.646,3.07320138235663,2.3165736780614));
#25119=CARTESIAN_POINT('Ctrl Pts',(-5.646,3.10039051575116,2.27454131446345));
#25120=CARTESIAN_POINT('Ctrl Pts',(-5.646,3.11563505786325,2.25097439426627));
#25121=CARTESIAN_POINT('Ctrl Pts',(-5.646,3.13064004341249,2.22724023348114));
#25122=CARTESIAN_POINT('Ctrl Pts',(-5.646,3.14540233301013,2.2033432169401));
#25123=CARTESIAN_POINT('Ctrl Pts',(-5.646,3.15850930411529,2.182125810031));
#25124=CARTESIAN_POINT('Ctrl Pts',(-5.646,3.1714273968094,2.16077571267399));
#25125=CARTESIAN_POINT('Ctrl Pts',(-5.646,3.18413915338665,2.13932213297246));
#25126=CARTESIAN_POINT('Ctrl Pts',(-5.646,3.24649773775284,2.0340798046093));
#25127=CARTESIAN_POINT('Ctrl Pts',(-5.646,3.30396139749785,1.92624527420896));
#25128=CARTESIAN_POINT('Ctrl Pts',(-5.646,3.35635415521047,1.8162165162223));
#25129=CARTESIAN_POINT('Ctrl Pts',(-5.646,3.40862386086259,1.7064461768793));
#25130=CARTESIAN_POINT('Ctrl Pts',(-5.646,3.45584679995269,1.59449106356881));
#25131=CARTESIAN_POINT('Ctrl Pts',(-5.646,3.49780098019105,1.48072575857657));
#25132=CARTESIAN_POINT('Ctrl Pts',(-5.646,3.53864854028781,1.36996122674223));
#25133=CARTESIAN_POINT('Ctrl Pts',(-5.646,3.57450174328363,1.2574799650644));
#25134=CARTESIAN_POINT('Ctrl Pts',(-5.646,3.60510776453686,1.14362007387887));
#25135=CARTESIAN_POINT('Ctrl Pts',(-5.646,3.62669073740589,1.06332754183119));
#25136=CARTESIAN_POINT('Ctrl Pts',(-5.646,3.64566336814893,0.982349262158363));
#25137=CARTESIAN_POINT('Ctrl Pts',(-5.646,3.66192149868813,0.900804466306592));
#25138=CARTESIAN_POINT('Ctrl Pts',(-5.646,3.66778547684093,0.871392911257449));
#25139=CARTESIAN_POINT('Ctrl Pts',(-5.646,3.67329619980581,0.841907674560768));
#25140=CARTESIAN_POINT('Ctrl Pts',(-5.646,3.67844834487312,0.812354423083884));
#25141=CARTESIAN_POINT('Ctrl Pts',(-5.646,3.68152767470266,0.794691060029537));
#25142=CARTESIAN_POINT('Ctrl Pts',(-5.646,3.68447904596225,0.777002104932098));
#25143=CARTESIAN_POINT('Ctrl Pts',(-5.646,3.68729866107252,0.759306528355325));
#25144=CARTESIAN_POINT('Ctrl Pts',(-5.646,3.70576394677868,0.643420542344302));
#25145=CARTESIAN_POINT('Ctrl Pts',(-5.646,3.71861385866923,0.52707879665178));
#25146=CARTESIAN_POINT('Ctrl Pts',(-5.646,3.72564577564316,0.410622409434895));
#25147=CARTESIAN_POINT('Ctrl Pts',(-5.646,3.73068658626485,0.327140963930941));
#25148=CARTESIAN_POINT('Ctrl Pts',(-5.646,3.73273671488304,0.243600328307105));
#25149=CARTESIAN_POINT('Ctrl Pts',(-5.646,3.7317049764916,0.160125554237579));
#25150=CARTESIAN_POINT('Ctrl Pts',(-5.646,3.730253423903,0.0426849070845082));
#25151=CARTESIAN_POINT('Ctrl Pts',(-5.646,3.72270365442221,-0.0746261863591401));
#25152=CARTESIAN_POINT('Ctrl Pts',(-5.646,3.70927694293084,-0.191449747144352));
#25153=CARTESIAN_POINT('Ctrl Pts',(-5.646,3.69573214444074,-0.309300763065067));
#25154=CARTESIAN_POINT('Ctrl Pts',(-5.646,3.67620617301247,-0.426656441051207));
#25155=CARTESIAN_POINT('Ctrl Pts',(-5.646,3.65087713531433,-0.543130167681983));
#25156=CARTESIAN_POINT('Ctrl Pts',(-5.646,3.64410795568506,-0.574257744933452));
#25157=CARTESIAN_POINT('Ctrl Pts',(-5.646,3.63692405661425,-0.605322188393886));
#25158=CARTESIAN_POINT('Ctrl Pts',(-5.646,3.62932830866254,-0.636315774732953));
#25159=CARTESIAN_POINT('Ctrl Pts',(-5.646,3.62539844276379,-0.652351145944345));
#25160=CARTESIAN_POINT('Ctrl Pts',(-5.646,3.6213605487996,-0.668358452270878));
#25161=CARTESIAN_POINT('Ctrl Pts',(-5.646,3.61721597080615,-0.684334502599823));
#25162=CARTESIAN_POINT('Ctrl Pts',(-5.646,3.58784792720512,-0.797539114353967));
#25163=CARTESIAN_POINT('Ctrl Pts',(-5.646,3.55311857210295,-0.90921231416928));
#25164=CARTESIAN_POINT('Ctrl Pts',(-5.646,3.51327894740302,-1.0190143738027));
#25165=CARTESIAN_POINT('Ctrl Pts',(-5.646,3.47320242549391,-1.12946934625056));
#25166=CARTESIAN_POINT('Ctrl Pts',(-5.646,3.42795422369401,-1.23803164326406));
#25167=CARTESIAN_POINT('Ctrl Pts',(-5.646,3.37774022348495,-1.34433650746171));
#25168=CARTESIAN_POINT('Ctrl Pts',(-5.646,3.32790839941417,-1.44983229087888));
#25169=CARTESIAN_POINT('Ctrl Pts',(-5.646,3.27318555283625,-1.55310558042916));
#25170=CARTESIAN_POINT('Ctrl Pts',(-5.646,3.21373162439723,-1.65377022854507));
#25171=CARTESIAN_POINT('Ctrl Pts',(-5.646,3.17762547871062,-1.71490348829414));
#25172=CARTESIAN_POINT('Ctrl Pts',(-5.646,3.13977370288082,-1.77507403709529));
#25173=CARTESIAN_POINT('Ctrl Pts',(-5.646,3.10020581820815,-1.83418830757275));
#25174=CARTESIAN_POINT('Ctrl Pts',(-5.646,3.08642921800113,-1.85477049632594));
#25175=CARTESIAN_POINT('Ctrl Pts',(-5.646,3.07244454081104,-1.87522458253508));
#25176=CARTESIAN_POINT('Ctrl Pts',(-5.646,3.05825291307383,-1.89554643852077));
#25177=CARTESIAN_POINT('Ctrl Pts',(-5.646,3.04634228662547,-1.91260198985464));
#25178=CARTESIAN_POINT('Ctrl Pts',(-5.646,3.03428371887915,-1.92956725129706));
#25179=CARTESIAN_POINT('Ctrl Pts',(-5.646,3.02209343607064,-1.94641861659085));
#25180=CARTESIAN_POINT('Ctrl Pts',(-5.646,2.95436095457071,-2.04004932278038));
#25181=CARTESIAN_POINT('Ctrl Pts',(-5.646,2.88247755796715,-2.13029552606011));
#25182=CARTESIAN_POINT('Ctrl Pts',(-5.646,2.80663876729683,-2.21681622171986));
#25183=CARTESIAN_POINT('Ctrl Pts',(-5.646,2.73167582096858,-2.30233771023118));
#25184=CARTESIAN_POINT('Ctrl Pts',(-5.646,2.65284778055453,-2.38421985926057));
#25185=CARTESIAN_POINT('Ctrl Pts',(-5.646,2.57030739842824,-2.46209859964859));
#25186=CARTESIAN_POINT('Ctrl Pts',(-5.646,2.48978889553354,-2.53806965068848));
#25187=CARTESIAN_POINT('Ctrl Pts',(-5.646,2.40573718380752,-2.61023146648245));
#25188=CARTESIAN_POINT('Ctrl Pts',(-5.646,2.31826727017074,-2.6782052332885));
#25189=CARTESIAN_POINT('Ctrl Pts',(-5.646,2.23079735653395,-2.74617900009456));
#25190=CARTESIAN_POINT('Ctrl Pts',(-5.646,2.13990886542514,-2.80996531714783));
#25191=CARTESIAN_POINT('Ctrl Pts',(-5.646,2.0456960854184,-2.86913603522103));
#25192=CARTESIAN_POINT('Origin',(-5.646,0.,0.));
#25193=CARTESIAN_POINT('Origin',(-7.03243520205041,0.,0.));
#25194=CARTESIAN_POINT('Ctrl Pts',(-5.646,2.04569608541839,-2.86913603522103));
#25195=CARTESIAN_POINT('Ctrl Pts',(-5.60642726334599,2.99688291874876,-2.19093912940735));
#25196=CARTESIAN_POINT('Ctrl Pts',(-5.52728179003796,4.15588292084424,0.17368053733326));
#25197=CARTESIAN_POINT('Ctrl Pts',(-5.40856358007592,2.11478894550069,3.58630724545133));
#25198=CARTESIAN_POINT('Ctrl Pts',(-5.28984537011388,-1.85304107076213,
3.72388412481386));
#25199=CARTESIAN_POINT('Ctrl Pts',(-5.20613591077205,-3.46080642106957,
1.43446279409787));
#25200=CARTESIAN_POINT('Ctrl Pts',(-5.16199918808422,-3.52857683297957,
0.136750902370548));
#25201=CARTESIAN_POINT('Ctrl Pts',(-5.1574352020504,-3.52758964538326,0.0024499632266353));
#25202=CARTESIAN_POINT('Ctrl Pts',(-5.89440495331884,2.29547565001616,-3.2194576469));
#25203=CARTESIAN_POINT('Ctrl Pts',(-5.85483221666482,3.36280242943815,-2.45845287482839));
#25204=CARTESIAN_POINT('Ctrl Pts',(-5.7756867433568,4.66331637290333,0.194886937102771));
#25205=CARTESIAN_POINT('Ctrl Pts',(-5.65696853339476,2.37300475076541,4.02419548734008));
#25206=CARTESIAN_POINT('Ctrl Pts',(-5.53825032343272,-2.07929745123621,
4.17857050855309));
#25207=CARTESIAN_POINT('Ctrl Pts',(-5.41953211347068,-4.63786592085608,
0.535227138001458));
#25208=CARTESIAN_POINT('Ctrl Pts',(-5.30081390350864,-2.97522613263464,
-3.59840638997019));
#25209=CARTESIAN_POINT('Ctrl Pts',(-5.1820956935466,1.39596514616172,-4.45488062147499));
#25210=CARTESIAN_POINT('Ctrl Pts',(-5.06337748358457,4.49629836096393,-1.25703816033307));
#25211=CARTESIAN_POINT('Ctrl Pts',(-4.94465927362252,3.5038389764095,3.08550240959749));
#25212=CARTESIAN_POINT('Ctrl Pts',(-4.82594106366049,-0.67811856098812,
4.61915125015357));
#25213=CARTESIAN_POINT('Ctrl Pts',(-4.70722285369845,-4.24278039300494,
1.94822471606856));
#25214=CARTESIAN_POINT('Ctrl Pts',(-4.58850464373641,-3.94535535609007,
-2.49618760971672));
#25215=CARTESIAN_POINT('Ctrl Pts',(-4.46978643377437,-0.0565651229095746,
-4.66834792415271));
#25216=CARTESIAN_POINT('Ctrl Pts',(-4.35106822381233,3.88371186515834,-2.5910446357827));
#25217=CARTESIAN_POINT('Ctrl Pts',(-4.2323500138503,4.28874367012574,1.84483192149852));
#25218=CARTESIAN_POINT('Ctrl Pts',(-4.11363180388825,0.789837394669197,
4.60139866153259));
#25219=CARTESIAN_POINT('Ctrl Pts',(-3.99491359392622,-3.42803786777068,
3.16942868543038));
#25220=CARTESIAN_POINT('Ctrl Pts',(-3.87619538396417,-4.52545532779526,
-1.14759516447504));
#25221=CARTESIAN_POINT('Ctrl Pts',(-3.75747717400214,-1.5034626703308,-4.41999081254857));
#25222=CARTESIAN_POINT('Ctrl Pts',(-3.6387589640401,2.88709478481946,-3.66897858534264));
#25223=CARTESIAN_POINT('Ctrl Pts',(-3.52004075407806,4.64960133826196,0.421814252099659));
#25224=CARTESIAN_POINT('Ctrl Pts',(-3.40132254411602,2.17969083882637,4.12863990933018));
#25225=CARTESIAN_POINT('Ctrl Pts',(-3.28260433415398,-2.27433828109485,
4.07726688351253));
#25226=CARTESIAN_POINT('Ctrl Pts',(-3.16388612419194,-4.65809355158234,
0.3144586843738));
#25227=CARTESIAN_POINT('Ctrl Pts',(-3.0451679142299,-2.80170153293177,-3.73459345798));
#25228=CARTESIAN_POINT('Ctrl Pts',(-2.92644970426786,1.60501005627966,-4.38413760326885));
#25229=CARTESIAN_POINT('Ctrl Pts',(-2.80773149430583,4.55072071104292,-1.04290977799098));
#25230=CARTESIAN_POINT('Ctrl Pts',(-2.68901328434378,3.3540229184984,3.24765300716171));
#25231=CARTESIAN_POINT('Ctrl Pts',(-2.57029507438175,-0.89575893480859,
4.58195763048246));
#25232=CARTESIAN_POINT('Ctrl Pts',(-2.45157686441971,-4.33015359714177,
1.74541961151293));
#25233=CARTESIAN_POINT('Ctrl Pts',(-2.33285865445767,-3.82291659791893,
-2.67993068572906));
#25234=CARTESIAN_POINT('Ctrl Pts',(-2.21414044449563,0.164226774937983,
-4.66580639995998));
#25235=CARTESIAN_POINT('Ctrl Pts',(-2.09542223453359,4.00187857869148,-2.40451401256942));
#25236=CARTESIAN_POINT('Ctrl Pts',(-1.97670402457155,4.1967193464349,2.0455479760931));
#25237=CARTESIAN_POINT('Ctrl Pts',(-1.85798581460952,0.57139034901314,4.63359826316093));
#25238=CARTESIAN_POINT('Ctrl Pts',(-1.73926760464748,-3.57406114296456,
3.00379871855954));
#25239=CARTESIAN_POINT('Ctrl Pts',(-1.62054939468544,-4.46613322351616,
-1.36028446476434));
#25240=CARTESIAN_POINT('Ctrl Pts',(-1.5018311847234,-1.29279475375635,-4.48613436267166));
#25241=CARTESIAN_POINT('Ctrl Pts',(-1.38311297476136,3.05734278765604,-3.52836716825847));
#25242=CARTESIAN_POINT('Ctrl Pts',(-1.26439476479932,4.62445684929134,0.641185343188987));
#25243=CARTESIAN_POINT('Ctrl Pts',(-1.14567655483728,1.98204228209413,4.22708270409631));
#25244=CARTESIAN_POINT('Ctrl Pts',(-1.02695834487524,-2.46457632504579,
3.96517128675444));
#25245=CARTESIAN_POINT('Ctrl Pts',(-0.908240134913205,-4.6677520941769,
0.0938625728684425));
#25246=CARTESIAN_POINT('Ctrl Pts',(-0.789521924951166,-2.62198864448019,
-3.86288691828992));
#25247=CARTESIAN_POINT('Ctrl Pts',(-0.670803714989127,1.8105061821359,-4.30334604229383));
#25248=CARTESIAN_POINT('Ctrl Pts',(-0.552085505027087,4.59494203561066,
-0.826575758570605));
#25249=CARTESIAN_POINT('Ctrl Pts',(-0.433367295065051,3.19671586474552,
3.40260598297286));
#25250=CARTESIAN_POINT('Ctrl Pts',(-0.314649085103009,-1.11140164891628,
4.53447970224418));
#25251=CARTESIAN_POINT('Ctrl Pts',(-0.195930875140972,-4.40783774534056,
1.53872876298241));
#25252=CARTESIAN_POINT('Ctrl Pts',(-0.0772126651789329,-3.69192822260236,
-2.85768889042012));
#25253=CARTESIAN_POINT('Ctrl Pts',(0.0415055447831063,0.38465219730754,
-4.65282306587999));
#25254=CARTESIAN_POINT('Ctrl Pts',(0.160223754745145,4.11109324096666,-2.21260754752318));
#25255=CARTESIAN_POINT('Ctrl Pts',(0.278941964707184,4.09530784428149,2.24168986611549));
#25256=CARTESIAN_POINT('Ctrl Pts',(0.397660174669223,0.351665063214532,
4.65543246955561));
#25257=CARTESIAN_POINT('Ctrl Pts',(0.516378384631261,-3.71208972226839,
2.83145010358787));
#25258=CARTESIAN_POINT('Ctrl Pts',(0.635096594593301,-4.39682109636873,
-1.5699312219984));
#25259=CARTESIAN_POINT('Ctrl Pts',(0.753814804555339,-1.07923503423744,
-4.54224300716648));
#25260=CARTESIAN_POINT('Ctrl Pts',(0.872533014517378,3.22075197181392,-3.37986338944861));
#25261=CARTESIAN_POINT('Ctrl Pts',(0.991251224479416,4.58896816162396,0.859122230465463));
#25262=CARTESIAN_POINT('Ctrl Pts',(1.10996943444146,1.7799601967492,4.31607014461849));
#25263=CARTESIAN_POINT('Ctrl Pts',(1.22868764440349,-2.64930148668855,3.84420621558056));
#25264=CARTESIAN_POINT('Ctrl Pts',(1.34740585436553,-4.66696958885342,-0.126943499225333));
#25265=CARTESIAN_POINT('Ctrl Pts',(1.46612406432757,-2.43641076742186,-3.9825396881474));
#25266=CARTESIAN_POINT('Ctrl Pts',(1.58484227428961,2.01195248192434,-4.21292855455169));
#25267=CARTESIAN_POINT('Ctrl Pts',(1.70356048425165,4.62888517660782,-0.608392814765849));
#25268=CARTESIAN_POINT('Ctrl Pts',(1.82227869421369,3.03225824568999,3.5499478484512));
#25269=CARTESIAN_POINT('Ctrl Pts',(1.94099690417573,-1.32455832721829,4.47685883550902));
#25270=CARTESIAN_POINT('Ctrl Pts',(2.05971511413777,-4.47566223360264,1.32859601308357));
#25271=CARTESIAN_POINT('Ctrl Pts',(2.1784333240998,-3.55268156760687,-3.02905488138869));
#25272=CARTESIAN_POINT('Ctrl Pts',(2.29715153406185,0.60421721144437,-4.62943207712054));
#25273=CARTESIAN_POINT('Ctrl Pts',(2.41586974402388,4.21111201543463,-2.01575181724849));
#25274=CARTESIAN_POINT('Ctrl Pts',(2.53458795398592,3.98473576383927,2.43281743821001));
#25275=CARTESIAN_POINT('Ctrl Pts',(2.65330616394796,0.131153156369908,4.66685318441158));
#25276=CARTESIAN_POINT('Ctrl Pts',(2.77202437391,-3.84181492370588,2.65276796709946));
#25277=CARTESIAN_POINT('Ctrl Pts',(2.89074258387204,-4.31767395183015,-1.77606628281883));
#25278=CARTESIAN_POINT('Ctrl Pts',(3.00946079383408,-0.863261230747963,
-4.58819134766261));
#25279=CARTESIAN_POINT('Ctrl Pts',(3.12817900379611,3.37695682562491,-3.22379937234679));
#25280=CARTESIAN_POINT('Ctrl Pts',(3.24689721375816,4.54321465292177,1.07513739250159));
#25281=CARTESIAN_POINT('Ctrl Pts',(3.36561542372019,1.57389661224691,4.39540319529804));
#25282=CARTESIAN_POINT('Ctrl Pts',(3.48433363368224,-2.82810056545818,3.71464224211883));
#25283=CARTESIAN_POINT('Ctrl Pts',(3.60305184364427,-4.6557477852134,-0.34746561809583));
#25284=CARTESIAN_POINT('Ctrl Pts',(3.72177005360631,-2.2453830115206,-4.09328412486269));
#25285=CARTESIAN_POINT('Ctrl Pts',(3.84048826356835,2.20889835123907,-4.11308738895392));
#25286=CARTESIAN_POINT('Ctrl Pts',(3.9592064735304,4.6524742083031,-0.388848989137025));
#25287=CARTESIAN_POINT('Ctrl Pts',(4.07792468349242,2.86101792796951,3.68934902267531));
#25288=CARTESIAN_POINT('Ctrl Pts',(4.19664289345447,-1.53475217080446,4.4092239191823));
#25289=CARTESIAN_POINT('Ctrl Pts',(4.3153611034165,-4.5334753488889,1.11549139678222));
#25290=CARTESIAN_POINT('Ctrl Pts',(4.43407931337854,-3.40548810644487,-3.1936453391291));
#25291=CARTESIAN_POINT('Ctrl Pts',(4.55279752334059,0.822430683944178,-4.59568575572627));
#25292=CARTESIAN_POINT('Ctrl Pts',(4.67151573330262,4.30171117536757,-1.81438715796713));
#25293=CARTESIAN_POINT('Ctrl Pts',(4.79023394326467,3.86525043796889,2.61850316919032));
#25294=CARTESIAN_POINT('Ctrl Pts',(4.9089521532267,-0.0896521200581657,
4.66783486132999));
#25295=CARTESIAN_POINT('Ctrl Pts',(5.02767036318874,-3.96294657181035,2.46815199375055));
#25296=CARTESIAN_POINT('Ctrl Pts',(5.14638857315078,-4.22886882997703,-1.97822855457275));
#25297=CARTESIAN_POINT('Ctrl Pts',(5.26510678311281,-0.645356443706703,
-4.62387660473814));
#25298=CARTESIAN_POINT('Ctrl Pts',(5.38382499307485,3.52560794268368,-3.06052420832841));
#25299=CARTESIAN_POINT('Ctrl Pts',(5.5025432030369,4.48729866679715,1.28874763636593));
#25300=CARTESIAN_POINT('Ctrl Pts',(5.62126141299893,1.36431246135956,4.46490440021477));
#25301=CARTESIAN_POINT('Ctrl Pts',(5.73997962296097,-3.00057361511833,3.57676918119331));
#25302=CARTESIAN_POINT('Ctrl Pts',(5.85869783292301,-4.63411178471802,-0.567210509437168));
#25303=CARTESIAN_POINT('Ctrl Pts',(5.97741604288506,-2.04933267669613,-4.19487251004172));
#25304=CARTESIAN_POINT('Ctrl Pts',(6.09613425284708,2.40090325224437,-4.00404587494208));
#25305=CARTESIAN_POINT('Ctrl Pts',(6.21485246280913,4.66565636563465,-0.168435367697401));
#25306=CARTESIAN_POINT('Ctrl Pts',(6.33357067277117,2.68337795002623,3.82049768650519));
#25307=CARTESIAN_POINT('Ctrl Pts',(6.4522888827332,-1.7415130081437,4.33172624224391));
#25308=CARTESIAN_POINT('Ctrl Pts',(6.57100709269525,-4.58114777208862,0.899891596563583));
#25309=CARTESIAN_POINT('Ctrl Pts',(6.68972530265728,-3.25067708841222,-3.35109209992061));
#25310=CARTESIAN_POINT('Ctrl Pts',(6.80844351261933,1.03880450459045,-4.55165958706503));
#25311=CARTESIAN_POINT('Ctrl Pts',(6.92716172258136,4.38268806427942,-1.6089639916732));
#25312=CARTESIAN_POINT('Ctrl Pts',(7.0458799325434,3.73711913709867,2.79833170843078));
#25313=CARTESIAN_POINT('Ctrl Pts',(7.16459814250544,-0.310256858383678,
4.65837530444943));
#25314=CARTESIAN_POINT('Ctrl Pts',(7.28331635246748,-4.07521371358196,2.27801514128243));
#25315=CARTESIAN_POINT('Ctrl Pts',(7.40203456242951,-4.13060437430629,-2.1759658311288));
#25316=CARTESIAN_POINT('Ctrl Pts',(7.52075277239156,-0.426008092847812,
-4.64921895592221));
#25317=CARTESIAN_POINT('Ctrl Pts',(7.63947098235358,3.66637281314061,-2.89040311900293));
#25318=CARTESIAN_POINT('Ctrl Pts',(7.75818919231564,4.42134527877262,1.4994751485615));
#25319=CARTESIAN_POINT('Ctrl Pts',(7.87690740227767,1.1516765518288,4.52441829578632));
#25320=CARTESIAN_POINT('Ctrl Pts',(7.99562561223971,-3.16633483979384,3.4308954337878));
#25321=CARTESIAN_POINT('Ctrl Pts',(8.11434382220175,-4.6021099837965,-0.785686637482825));
#25322=CARTESIAN_POINT('Ctrl Pts',(8.23306203216379,-1.84869829761031,-4.28707760597953));
#25323=CARTESIAN_POINT('Ctrl Pts',(8.35178024212583,2.58753769929621,-3.8860479217322));
#25324=CARTESIAN_POINT('Ctrl Pts',(8.47049845208786,4.66840216212944,0.0523550179394298));
#25325=CARTESIAN_POINT('Ctrl Pts',(8.58921666204991,2.49973566536485,3.94310048040643));
#25326=CARTESIAN_POINT('Ctrl Pts',(8.70793487201194,-1.94437834681552,4.24453915516319));
#25327=CARTESIAN_POINT('Ctrl Pts',(8.82665308197398,-4.6185728672708,0.682278876258279));
#25328=CARTESIAN_POINT('Ctrl Pts',(8.94537129193602,-3.08859480211636,-3.50104297940172));
#25329=CARTESIAN_POINT('Ctrl Pts',(9.06408950189806,1.25285467818704,-4.49745205095322));
#25330=CARTESIAN_POINT('Ctrl Pts',(9.18280771186011,4.45386154923497,-1.39994181862131));
#25331=CARTESIAN_POINT('Ctrl Pts',(9.30152592182213,3.60062847138283,2.97190080694926));
#25332=CARTESIAN_POINT('Ctrl Pts',(9.42024413178418,-0.530167599493716,
4.63849567335416));
#25333=CARTESIAN_POINT('Ctrl Pts',(9.53896234174621,-4.17836522456791,2.08278271679982));
#25334=CARTESIAN_POINT('Ctrl Pts',(9.65768055170827,-4.02310038740015,-2.36883580439405));
#25335=CARTESIAN_POINT('Ctrl Pts',(9.77639876167028,-0.205706826937308,
-4.66416171424508));
#25336=CARTESIAN_POINT('Ctrl Pts',(9.89511697163234,3.79893656747558,-2.71381663926939));
#25337=CARTESIAN_POINT('Ctrl Pts',(10.0138351815944,4.34550201650593,1.70684856382205));
#25338=CARTESIAN_POINT('Ctrl Pts',(10.1325533915564,0.936464517714484,4.57381175851606));
#25339=CARTESIAN_POINT('Ctrl Pts',(10.2512716015184,-3.32501345693721,3.27734729720019));
#25340=CARTESIAN_POINT('Ctrl Pts',(10.3699898114805,-4.55981396559068,-1.00240530449618));
#25341=CARTESIAN_POINT('Ctrl Pts',(10.4887080214425,-1.64392866273208,-4.3696931639561));
#25342=CARTESIAN_POINT('Ctrl Pts',(10.6074262314046,2.76838421963613,-3.75935747272765));
#25343=CARTESIAN_POINT('Ctrl Pts',(10.7261444413666,4.66070545585953,0.273028293396762));
#25344=CARTESIAN_POINT('Ctrl Pts',(10.8448626513287,2.31050185373462,4.05688316064908));
#25345=CARTESIAN_POINT('Ctrl Pts',(10.9635808612907,-2.14289440803709,4.14785768214349));
#25346=CARTESIAN_POINT('Ctrl Pts',(11.0822990712527,-4.64566692020879,0.463140002285691));
#25347=CARTESIAN_POINT('Ctrl Pts',(11.2010172812147,-2.91960380088829,-3.64316256034107));
#25348=CARTESIAN_POINT('Ctrl Pts',(11.3197354911768,1.46410240719433,-4.43318440139384));
#25349=CARTESIAN_POINT('Ctrl Pts',(11.4384537011388,4.51507242599213,-1.18778818945209));
#25350=CARTESIAN_POINT('Ctrl Pts',(11.5571719111009,3.45608374964487,3.13882221709585));
#25351=CARTESIAN_POINT('Ctrl Pts',(11.6758901210629,-0.748892436729798,
4.60824043589683));
#25352=CARTESIAN_POINT('Ctrl Pts',(11.794608331025,-4.27217037042104,1.882891425132));
#25353=CARTESIAN_POINT('Ctrl Pts',(11.913326540987,-3.90659733958176,-2.55640705313474));
#25354=CARTESIAN_POINT('Ctrl Pts',(12.032044750949,0.0150545743428436,-4.66867145609391));
#25355=CARTESIAN_POINT('Ctrl Pts',(12.150762960911,3.92300267965357,-2.53115976411015));
#25356=CARTESIAN_POINT('Ctrl Pts',(12.2694811708731,4.2599385319979,1.91040401566542));
#25357=CARTESIAN_POINT('Ctrl Pts',(12.3881993808351,0.719157751281456,4.61297431003179));
#25358=CARTESIAN_POINT('Ctrl Pts',(12.5069175907972,-3.47625451873963,3.11646822135571));
#25359=CARTESIAN_POINT('Ctrl Pts',(12.6256358007592,-4.50731835499655,-1.21688171765083));
#25360=CARTESIAN_POINT('Ctrl Pts',(12.7443540107213,-1.4354817816321,-4.44253443552631));
#25361=CARTESIAN_POINT('Ctrl Pts',(12.8630722206833,2.94303823237952,-3.62425782013981));
#25362=CARTESIAN_POINT('Ctrl Pts',(12.9817904306454,4.64258356746131,0.493090665633712));
#25363=CARTESIAN_POINT('Ctrl Pts',(13.1005086406074,2.11609960396394,4.1615915562441));
#25364=CARTESIAN_POINT('Ctrl Pts',(13.2192268505694,-2.33661676455732,4.04189743164783));
#25365=CARTESIAN_POINT('Ctrl Pts',(13.3379450605315,-4.66237004285371,0.242966397108652));
#25366=CARTESIAN_POINT('Ctrl Pts',(13.4566632704935,-2.74408072785275,-3.77713530538915));
#25367=CARTESIAN_POINT('Ctrl Pts',(13.5753814804556,1.67207256885561,-4.35899590256187));
#25368=CARTESIAN_POINT('Ctrl Pts',(13.6940996904176,4.56618870795816,-0.972986203420864));
#25369=CARTESIAN_POINT('Ctrl Pts',(13.8128179003796,3.30379891551882,3.29873880951256));
#25370=CARTESIAN_POINT('Ctrl Pts',(13.9315361103416,-0.965924276211378,
4.56764636844593));
#25371=CARTESIAN_POINT('Ctrl Pts',(14.0502543203037,-4.35645324991307,1.67884715610445));
#25372=CARTESIAN_POINT('Ctrl Pts',(14.1689725302657,-3.78129131083658,-2.73837176255018));
#25373=CARTESIAN_POINT('Ctrl Pts',(14.2876907402277,0.235659599280402,-4.66252555962526));
#25374=CARTESIAN_POINT('Ctrl Pts',(14.4064089501898,4.03852700863023,-2.34324533249394));
#25375=CARTESIAN_POINT('Ctrl Pts',(14.5251271601518,4.16440214623227,2.11045567438585));
#25376=CARTESIAN_POINT('Ctrl Pts',(14.6438453701139,0.501089014228282,4.64034903703233));
#25377=CARTESIAN_POINT('Ctrl Pts',(14.7625635800759,-3.6213485503704,2.95146328864409));
#25378=CARTESIAN_POINT('Ctrl Pts',(14.881281790038,-4.44148208883051,-1.43448156720096));
#25379=CARTESIAN_POINT('Ctrl Pts',(14.960427263346,-2.30148466178617,-3.47211737542815));
#25380=CARTESIAN_POINT('Ctrl Pts',(15.,-1.03647793659398,-3.81573446232228));
#25381=CARTESIAN_POINT('Ctrl Pts',(-5.81160330221256,2.21221579515024,-3.10268377634035));
#25382=CARTESIAN_POINT('Ctrl Pts',(-5.77203056555854,3.24082925920835,-2.36928162635471));
#25383=CARTESIAN_POINT('Ctrl Pts',(-5.69288509225051,4.49417188888364,0.187818137179599));
#25384=CARTESIAN_POINT('Ctrl Pts',(-5.57416688228849,2.28693281567717,3.87823274004383));
#25385=CARTESIAN_POINT('Ctrl Pts',(-5.45544867232644,-2.00387865774485,
4.02700838064001));
#25386=CARTESIAN_POINT('Ctrl Pts',(-5.33673046236441,-4.46964455747315,
0.515813761157338));
#25387=CARTESIAN_POINT('Ctrl Pts',(-5.21801225240236,-2.8673108532917,-3.46788756099659));
#25388=CARTESIAN_POINT('Ctrl Pts',(-5.09929404244033,1.34533169445575,-4.29329637030406));
#25389=CARTESIAN_POINT('Ctrl Pts',(-4.98057583247828,4.33321183509941,-1.21144376912727));
#25390=CARTESIAN_POINT('Ctrl Pts',(-4.86185762251625,3.37675022918306,2.97358726782297));
#25391=CARTESIAN_POINT('Ctrl Pts',(-4.74313941255421,-0.653522328408015,
4.45160869195271));
#25392=CARTESIAN_POINT('Ctrl Pts',(-4.62442120259217,-4.08888928997927,
1.87756009930171));
#25393=CARTESIAN_POINT('Ctrl Pts',(-4.50570299263013,-3.80225224177903,
-2.40564767386436));
#25394=CARTESIAN_POINT('Ctrl Pts',(-4.3869847826681,-0.0545134331328301,
-4.4990209392963));
#25395=CARTESIAN_POINT('Ctrl Pts',(-4.26826657270605,3.74284463956531,-2.49706411356509));
#25396=CARTESIAN_POINT('Ctrl Pts',(-4.14954836274402,4.13318541990895,1.7779174944015));
#25397=CARTESIAN_POINT('Ctrl Pts',(-4.03083015278198,0.761188976269582,
4.43450001255902));
#25398=CARTESIAN_POINT('Ctrl Pts',(-3.91211194281993,-3.30369852426972,
3.05446942966354));
#25399=CARTESIAN_POINT('Ctrl Pts',(-3.7933937328579,-4.36131124123449,-1.10597041152313));
#25400=CARTESIAN_POINT('Ctrl Pts',(-3.67467552289586,-1.44893014513188,
-4.25967205963177));
#25401=CARTESIAN_POINT('Ctrl Pts',(-3.55595731293382,2.78237614283929,-3.53590001205453));
#25402=CARTESIAN_POINT('Ctrl Pts',(-3.43723910297178,4.48095431619256,0.406514506528419));
#25403=CARTESIAN_POINT('Ctrl Pts',(-3.31852089300974,2.10063064801496,3.97888882848467));
#25404=CARTESIAN_POINT('Ctrl Pts',(-3.1998026830477,-2.19184510579209,3.92937916840284));
#25405=CARTESIAN_POINT('Ctrl Pts',(-3.08108447308566,-4.48913850601091,
0.30305286335275));
#25406=CARTESIAN_POINT('Ctrl Pts',(-2.96236626312363,-2.70008021405268,
-3.59913494885035));
#25407=CARTESIAN_POINT('Ctrl Pts',(-2.84364805316158,1.54679427675559,-4.2251192923764));
#25408=CARTESIAN_POINT('Ctrl Pts',(-2.72492984319955,4.38566021652883,-1.00508209868054));
#25409=CARTESIAN_POINT('Ctrl Pts',(-2.60621163323751,3.23236819242489,3.12985645461311));
#25410=CARTESIAN_POINT('Ctrl Pts',(-2.48749342327547,-0.863268605884161,
4.41576413271522));
#25411=CARTESIAN_POINT('Ctrl Pts',(-2.36877521331343,-4.17309335559985,
1.68211099678916));
#25412=CARTESIAN_POINT('Ctrl Pts',(-2.25005700335139,-3.68425449487943,
-2.58272615213143));
#25413=CARTESIAN_POINT('Ctrl Pts',(-2.13133879338935,0.158270058539632,
-4.49657159945561));
#25414=CARTESIAN_POINT('Ctrl Pts',(-2.01262058342732,3.85672529438174,-2.31729919602012));
#25415=CARTESIAN_POINT('Ctrl Pts',(-1.89390237346527,4.04449893682408,1.97135331948257));
#25416=CARTESIAN_POINT('Ctrl Pts',(-1.77518416350324,0.550665285983065,
4.46553169321277));
#25417=CARTESIAN_POINT('Ctrl Pts',(-1.6564659535412,-3.44442534741907,2.89484707476759));
#25418=CARTESIAN_POINT('Ctrl Pts',(-1.53774774357916,-4.30414082599316,
-1.31094519727446));
#25419=CARTESIAN_POINT('Ctrl Pts',(-1.41902953361712,-1.24590342490763,
-4.3234164981008));
#25420=CARTESIAN_POINT('Ctrl Pts',(-1.30031132365508,2.94644903159558,-3.4003887519591));
#25421=CARTESIAN_POINT('Ctrl Pts',(-1.18159311369304,4.45672185018431,0.617928725931589));
#25422=CARTESIAN_POINT('Ctrl Pts',(-1.062874903731,1.91015105870255,4.07376097644183));
#25423=CARTESIAN_POINT('Ctrl Pts',(-0.944156693768964,-2.37518297115512,
3.82134942314577));
#25424=CARTESIAN_POINT('Ctrl Pts',(-0.825438483806927,-4.49844672084023,
0.0904580565999837));
#25425=CARTESIAN_POINT('Ctrl Pts',(-0.706720273844886,-2.52688574325886,
-3.7227750403103));
#25426=CARTESIAN_POINT('Ctrl Pts',(-0.588002063882848,1.74483679376428,
-4.14725814525313));
#25427=CARTESIAN_POINT('Ctrl Pts',(-0.469283853920809,4.42827757676548,
-0.79659479244981));
#25428=CARTESIAN_POINT('Ctrl Pts',(-0.350565643958771,3.08076686788102,
3.27918908665064));
#25429=CARTESIAN_POINT('Ctrl Pts',(-0.231847433996731,-1.07108968133524,
4.37000829001264));
#25430=CARTESIAN_POINT('Ctrl Pts',(-0.113129224034693,-4.24795979980585,
1.48291709123456));
#25431=CARTESIAN_POINT('Ctrl Pts',(0.00558898592734578,-3.55801723644702,
-2.75403683805935));
#25432=CARTESIAN_POINT('Ctrl Pts',(0.124307195889386,0.370700367271144,
-4.48405918760526));
#25433=CARTESIAN_POINT('Ctrl Pts',(0.243025405851424,3.9619786003558,-2.13235342534128));
#25434=CARTESIAN_POINT('Ctrl Pts',(0.361743615813462,3.94676576031572,2.16038089082496));
#25435=CARTESIAN_POINT('Ctrl Pts',(0.480461825775502,0.338909718968374,
4.48657394485266));
#25436=CARTESIAN_POINT('Ctrl Pts',(0.59918003573754,-3.57744745258317,2.72874976578071));
#25437=CARTESIAN_POINT('Ctrl Pts',(0.71789824569958,-4.23734273886472,-1.51298779692127));
#25438=CARTESIAN_POINT('Ctrl Pts',(0.836616455661619,-1.04008979115191,
-4.37749000987822));
#25439=CARTESIAN_POINT('Ctrl Pts',(0.955334665623656,3.10393115442452,-3.25727139625099));
#25440=CARTESIAN_POINT('Ctrl Pts',(1.0740528755857,4.42252038287345,0.827960761939252));
#25441=CARTESIAN_POINT('Ctrl Pts',(1.19277108554773,1.71539875056379,4.15952072801739));
#25442=CARTESIAN_POINT('Ctrl Pts',(1.31148929550978,-2.55320791354339,3.70477191072022));
#25443=CARTESIAN_POINT('Ctrl Pts',(1.43020750547181,-4.4976925979915,-0.122339095200565));
#25444=CARTESIAN_POINT('Ctrl Pts',(1.54892571543385,-2.34803901454013,-3.83808785027642));
#25445=CARTESIAN_POINT('Ctrl Pts',(1.66764392539589,1.93897637710659,-4.06012021610996));
#25446=CARTESIAN_POINT('Ctrl Pts',(1.78636213535793,4.46098955637215,-0.586325624700695));
#25447=CARTESIAN_POINT('Ctrl Pts',(1.90508034531997,2.92227433823694,3.42118667311853));
#25448=CARTESIAN_POINT('Ctrl Pts',(2.02379855528201,-1.27651489269748,4.31447740624096));
#25449=CARTESIAN_POINT('Ctrl Pts',(2.14251676524405,-4.31332420662509,1.28040612650213));
#25450=CARTESIAN_POINT('Ctrl Pts',(2.26123497520609,-3.42382123676361,-2.91918716407984));
#25451=CARTESIAN_POINT('Ctrl Pts',(2.37995318516812,0.582301475883412,-4.46151662009971));
#25452=CARTESIAN_POINT('Ctrl Pts',(2.49867139513016,4.05836956520357,-1.94263790565087));
#25453=CARTESIAN_POINT('Ctrl Pts',(2.6173896050922,3.8402042714778,2.34457602000145));
#25454=CARTESIAN_POINT('Ctrl Pts',(2.73610781505424,0.126396062664967,4.4975804156885));
#25455=CARTESIAN_POINT('Ctrl Pts',(2.85482602501628,-3.70246735407811,2.55654866025033));
#25456=CARTESIAN_POINT('Ctrl Pts',(2.97354423497832,-4.16106636307827,-1.71164607390103));
#25457=CARTESIAN_POINT('Ctrl Pts',(3.09226244494036,-0.831949635356866,
-4.4217717449538));
#25458=CARTESIAN_POINT('Ctrl Pts',(3.2109806549024,3.25447025723634,-3.10686802181972));
#25459=CARTESIAN_POINT('Ctrl Pts',(3.32969886486444,4.37842641279199,1.03614077615325));
#25460=CARTESIAN_POINT('Ctrl Pts',(3.44841707482647,1.51680935736416,4.23597626688993));
#25461=CARTESIAN_POINT('Ctrl Pts',(3.56713528478851,-2.72552171970801,3.57990738925493));
#25462=CARTESIAN_POINT('Ctrl Pts',(3.68585349475055,-4.48687782360591,-0.334862593126525));
#25463=CARTESIAN_POINT('Ctrl Pts',(3.80457170471259,-2.16394008109515,-3.94481544380366));
#25464=CARTESIAN_POINT('Ctrl Pts',(3.92328991467463,2.1287787663781,-3.96390041803019));
#25465=CARTESIAN_POINT('Ctrl Pts',(4.04200812463667,4.48372298354147,-0.374744936061991));
#25466=CARTESIAN_POINT('Ctrl Pts',(4.16072633459871,2.75724512713418,3.55553158741935));
#25467=CARTESIAN_POINT('Ctrl Pts',(4.27944454456074,-1.47908473517061,4.24929569533909));
#25468=CARTESIAN_POINT('Ctrl Pts',(4.39816275452279,-4.36904036584561,1.0750310887848));
#25469=CARTESIAN_POINT('Ctrl Pts',(4.51688096448482,-3.28196667179659,-3.0778077141788));
#25470=CARTESIAN_POINT('Ctrl Pts',(4.63559917444687,0.792600065012534,-4.42899432119574));
#25471=CARTESIAN_POINT('Ctrl Pts',(4.7543173844089,4.14568257705346,-1.74857700160942));
#25472=CARTESIAN_POINT('Ctrl Pts',(4.87303559437094,3.72505283208995,2.52352669064166));
#25473=CARTESIAN_POINT('Ctrl Pts',(4.99175380433298,-0.0864003223296886,
4.4985264859222));
#25474=CARTESIAN_POINT('Ctrl Pts',(5.11047201429502,-3.8192054014747,2.37862894575603));
#25475=CARTESIAN_POINT('Ctrl Pts',(5.22919022425706,-4.07548231723908,-1.90647565998456));
#25476=CARTESIAN_POINT('Ctrl Pts',(5.34790843421909,-0.6219485352676,-4.45616265184752));
#25477=CARTESIAN_POINT('Ctrl Pts',(5.46662664418114,3.39772960704553,-2.94951505804741));
#25478=CARTESIAN_POINT('Ctrl Pts',(5.58534485414316,4.32453857141784,1.24200310167139));
#25479=CARTESIAN_POINT('Ctrl Pts',(5.70406306410522,1.31482709325133,4.30295657369375));
#25480=CARTESIAN_POINT('Ctrl Pts',(5.82278127406724,-2.89173894997714,3.44703516161749));
#25481=CARTESIAN_POINT('Ctrl Pts',(5.9414994840293,-4.46602658868237,-0.54663705456568));
#25482=CARTESIAN_POINT('Ctrl Pts',(6.06021769399132,-1.97500074412587,-4.04271908756276));
#25483=CARTESIAN_POINT('Ctrl Pts',(6.17893590395337,2.31381940261713,-3.8588139800092));
#25484=CARTESIAN_POINT('Ctrl Pts',(6.2976541139154,4.49642700706827,-0.162326000225504));
#25485=CARTESIAN_POINT('Ctrl Pts',(6.41637232387745,2.5860483797178,3.68192332049448));
#25486=CARTESIAN_POINT('Ctrl Pts',(6.53509053383948,-1.67834609094981,4.17460895884099));
#25487=CARTESIAN_POINT('Ctrl Pts',(6.65380874380152,-4.41498364892716,0.86725137068082));
#25488=CARTESIAN_POINT('Ctrl Pts',(6.77252695376356,-3.13277084854633,-3.2295436784073));
#25489=CARTESIAN_POINT('Ctrl Pts',(6.8912451637256,1.00112572882749,-4.38656503830979));
#25490=CARTESIAN_POINT('Ctrl Pts',(7.00996337368764,4.22372233003087,-1.55060479782585));
#25491=CARTESIAN_POINT('Ctrl Pts',(7.12868158364969,3.60156901833821,2.69683261742147));
#25492=CARTESIAN_POINT('Ctrl Pts',(7.24739979361171,-0.299003442996754,
4.48941003933905));
#25493=CARTESIAN_POINT('Ctrl Pts',(7.36611800357376,-3.92740046958695,2.19538860153057));
#25494=CARTESIAN_POINT('Ctrl Pts',(7.48483621353579,-3.9807820397889,-2.09704075113864));
#25495=CARTESIAN_POINT('Ctrl Pts',(7.60355442349784,-0.410556231277453,
-4.48058580335219));
#25496=CARTESIAN_POINT('Ctrl Pts',(7.72227263345987,3.53338875456248,-2.78556447948591));
#25497=CARTESIAN_POINT('Ctrl Pts',(7.84099084342191,4.26097739762341,1.44508725590692));
#25498=CARTESIAN_POINT('Ctrl Pts',(7.95970905338396,1.10990376170705,4.3603118237106));
#25499=CARTESIAN_POINT('Ctrl Pts',(8.07842726334598,-3.05148780178832,3.30645244269127));
#25500=CARTESIAN_POINT('Ctrl Pts',(8.19714547330804,-4.43518553424934,-0.757188772386117));
#25501=CARTESIAN_POINT('Ctrl Pts',(8.31586368327006,-1.7816436320778,-4.13157978605264));
#25502=CARTESIAN_POINT('Ctrl Pts',(8.43458189323211,2.49368437817648,-3.74509596436201));
#25503=CARTESIAN_POINT('Ctrl Pts',(8.55330010319414,4.49907320999184,0.0504560340860681));
#25504=CARTESIAN_POINT('Ctrl Pts',(8.67201831315618,2.40906703696972,3.80007915333722));
#25505=CARTESIAN_POINT('Ctrl Pts',(8.79073652311823,-1.87385324280966,4.09058425957148));
#25506=CARTESIAN_POINT('Ctrl Pts',(8.90945473308026,-4.45105128776116,0.65753174369126));
#25507=CARTESIAN_POINT('Ctrl Pts',(9.02817294304229,-2.97656749528695,-3.37405564658367));
#25508=CARTESIAN_POINT('Ctrl Pts',(9.14689115300435,1.20741202726054,-4.33432367926863));
#25509=CARTESIAN_POINT('Ctrl Pts',(9.26560936296637,4.29231426112518,-1.34916412788942));
#25510=CARTESIAN_POINT('Ctrl Pts',(9.38432757292842,3.47002904465779,2.86410614144681));
#25511=CARTESIAN_POINT('Ctrl Pts',(9.50304578289045,-0.510937738620143,
4.47025146803797));
#25512=CARTESIAN_POINT('Ctrl Pts',(9.6217639928525,-4.02681054256906,2.00723750824284));
#25513=CARTESIAN_POINT('Ctrl Pts',(9.74048220281453,-3.87717736078754,-2.28291508235387));
#25514=CARTESIAN_POINT('Ctrl Pts',(9.85920041277658,-0.198245575690498,
-4.49498656860741));
#25515=CARTESIAN_POINT('Ctrl Pts',(9.9779186227386,3.66114425098962,-2.61538301854392));
#25516=CARTESIAN_POINT('Ctrl Pts',(10.0966368327007,4.18788506804854,1.64493897061816));
#25517=CARTESIAN_POINT('Ctrl Pts',(10.2153550426627,0.902497744931939,4.40791372200438));
#25518=CARTESIAN_POINT('Ctrl Pts',(10.3340732526247,-3.20441094135405,3.15847369455137));
#25519=CARTESIAN_POINT('Ctrl Pts',(10.4527914625868,-4.39442364703602,-0.966046774546791));
#25520=CARTESIAN_POINT('Ctrl Pts',(10.5715096725488,-1.58430125528474,-4.21119877145971));
#25521=CARTESIAN_POINT('Ctrl Pts',(10.6902278825109,2.66797136257167,-3.62300074092517));
#25522=CARTESIAN_POINT('Ctrl Pts',(10.8089460924729,4.49165567315985,0.263125205955005));
#25523=CARTESIAN_POINT('Ctrl Pts',(10.9276643024349,2.22669697912923,3.90973478939049));
#25524=CARTESIAN_POINT('Ctrl Pts',(11.046382512397,-2.06516887110756,3.99740954795515));
#25525=CARTESIAN_POINT('Ctrl Pts',(11.165100722359,-4.47716260454366,0.446341318591266));
#25526=CARTESIAN_POINT('Ctrl Pts',(11.283818932321,-2.81370601507375,-3.51102036749106));
#25527=CARTESIAN_POINT('Ctrl Pts',(11.4025371422831,1.41099752937478,-4.27238710003659));
#25528=CARTESIAN_POINT('Ctrl Pts',(11.5212553522451,4.35130494063695,-1.14470558377753));
#25529=CARTESIAN_POINT('Ctrl Pts',(11.6399735622072,3.33072714592842,3.02497309730951));
#25530=CARTESIAN_POINT('Ctrl Pts',(11.7586917721692,-0.721729144628708,
4.44109362696541));
#25531=CARTESIAN_POINT('Ctrl Pts',(11.8774099821313,-4.11721325510543,1.81459653087615));
#25532=CARTESIAN_POINT('Ctrl Pts',(11.9961281920933,-3.76490002839014,-2.46368288059964));
#25533=CARTESIAN_POINT('Ctrl Pts',(12.1148464020553,0.0145085255642979,
-4.49933273631779));
#25534=CARTESIAN_POINT('Ctrl Pts',(12.2335646120174,3.78071032567269,-2.43935134322764));
#25535=CARTESIAN_POINT('Ctrl Pts',(12.3522828219794,4.1054250811977,1.84111120435702));
#25536=CARTESIAN_POINT('Ctrl Pts',(12.4710010319414,0.69307297447411,4.44565579739554));
#25537=CARTESIAN_POINT('Ctrl Pts',(12.5897192419035,-3.35016629527918,3.00342990975242));
#25538=CARTESIAN_POINT('Ctrl Pts',(12.7084374518655,-4.3438321197717,-1.17274385228079));
#25539=CARTESIAN_POINT('Ctrl Pts',(12.8271556618276,-1.38341501072103,-4.28139799640262));
#25540=CARTESIAN_POINT('Ctrl Pts',(12.9458738717896,2.83629044958729,-3.49280132653712));
#25541=CARTESIAN_POINT('Ctrl Pts',(13.0645920817516,4.47419108896694,0.475205632849264));
#25542=CARTESIAN_POINT('Ctrl Pts',(13.1833102917137,2.03934594904864,4.01064527677402));
#25543=CARTESIAN_POINT('Ctrl Pts',(13.3020285016757,-2.25186466854054,3.89529261205869));
#25544=CARTESIAN_POINT('Ctrl Pts',(13.4207467116377,-4.49325988344233,0.234153693318749));
#25545=CARTESIAN_POINT('Ctrl Pts',(13.5394649215998,-2.64454938970079,-3.64013374872553));
#25546=CARTESIAN_POINT('Ctrl Pts',(13.6581831315618,1.61142434572711,-4.20088951349786));
#25547=CARTESIAN_POINT('Ctrl Pts',(13.7769013415238,4.40056716929698,-0.937694742114035));
#25548=CARTESIAN_POINT('Ctrl Pts',(13.8956195514859,3.18396587864461,3.17908930919281));
#25549=CARTESIAN_POINT('Ctrl Pts',(14.0143377614479,-0.930888960089293,
4.40197195856363));
#25550=CARTESIAN_POINT('Ctrl Pts',(14.13305597141,-4.19843908613166,1.61795320998123));
#25551=CARTESIAN_POINT('Ctrl Pts',(14.251774181372,-3.64413901050886,-2.63904749591409));
#25552=CARTESIAN_POINT('Ctrl Pts',(14.3704923913341,0.227111922447612,-4.4934097594205));
#25553=CARTESIAN_POINT('Ctrl Pts',(14.4892106012961,3.89204443861984,-2.25825280979074));
#25554=CARTESIAN_POINT('Ctrl Pts',(14.6079288112581,4.01335392304761,2.03390673205702));
#25555=CARTESIAN_POINT('Ctrl Pts',(14.7266470212201,0.48291387105078,4.47203760783125));
#25556=CARTESIAN_POINT('Ctrl Pts',(14.8453652311822,-3.48999757972489,2.84440991822266));
#25557=CARTESIAN_POINT('Ctrl Pts',(14.9640834411442,-4.28038381967528,-1.38245107535402));
#25558=CARTESIAN_POINT('Ctrl Pts',(15.0432289144523,-2.218006852333,-3.34617921147789));
#25559=CARTESIAN_POINT('Ctrl Pts',(15.0828016511063,-0.99888354844532,-3.6773328645804));
#25560=CARTESIAN_POINT('Ctrl Pts',(-5.72880165110628,2.12895594028432,-2.98590990578069));
#25561=CARTESIAN_POINT('Ctrl Pts',(-5.68922891445227,3.11885608897856,-2.28011037788103));
#25562=CARTESIAN_POINT('Ctrl Pts',(-5.61008344114424,4.32502740486394,0.180749337256433));
#25563=CARTESIAN_POINT('Ctrl Pts',(-5.4913652311822,2.20086088058893,3.73226999274757));
#25564=CARTESIAN_POINT('Ctrl Pts',(-5.37264702122016,-1.92845986425349,
3.87544625272694));
#25565=CARTESIAN_POINT('Ctrl Pts',(-5.25392881125813,-4.30142319409022,
0.496400384313214));
#25566=CARTESIAN_POINT('Ctrl Pts',(-5.13521060129608,-2.75939557394876,
-3.337368732023));
#25567=CARTESIAN_POINT('Ctrl Pts',(-5.01649239133405,1.29469824274977,-4.13171211913313));
#25568=CARTESIAN_POINT('Ctrl Pts',(-4.897774181372,4.17012530923491,-1.16584937792148));
#25569=CARTESIAN_POINT('Ctrl Pts',(-4.77905597140997,3.24966148195661,2.86167212604844));
#25570=CARTESIAN_POINT('Ctrl Pts',(-4.66033776144792,-0.628926095827896,
4.28406613375186));
#25571=CARTESIAN_POINT('Ctrl Pts',(-4.5416195514859,-3.93499818695361,1.80689548253486));
#25572=CARTESIAN_POINT('Ctrl Pts',(-4.42290134152385,-3.65914912746798,
-2.31510773801199));
#25573=CARTESIAN_POINT('Ctrl Pts',(-4.30418313156181,-0.0524617433560917,
-4.32969395443989));
#25574=CARTESIAN_POINT('Ctrl Pts',(-4.18546492159977,3.60197741397228,-2.40308359134747));
#25575=CARTESIAN_POINT('Ctrl Pts',(-4.06674671163773,3.97762716969217,1.71100306730448));
#25576=CARTESIAN_POINT('Ctrl Pts',(-3.9480285016757,0.732540557869959,4.26760136358546));
#25577=CARTESIAN_POINT('Ctrl Pts',(-3.82931029171366,-3.17935918076875,
2.93951017389669));
#25578=CARTESIAN_POINT('Ctrl Pts',(-3.71059208175161,-4.19716715467372,
-1.06434565857122));
#25579=CARTESIAN_POINT('Ctrl Pts',(-3.59187387178958,-1.39439761993295,
-4.09935330671497));
#25580=CARTESIAN_POINT('Ctrl Pts',(-3.47315566182754,2.67765750085913,-3.40282143876642));
#25581=CARTESIAN_POINT('Ctrl Pts',(-3.35443745186551,4.31230729412316,0.391214760957178));
#25582=CARTESIAN_POINT('Ctrl Pts',(-3.23571924190346,2.02157045720355,3.82913774763917));
#25583=CARTESIAN_POINT('Ctrl Pts',(-3.11700103194143,-2.10935193048935,
3.78149145329314));
#25584=CARTESIAN_POINT('Ctrl Pts',(-2.99828282197938,-4.32018346043948,
0.291647042331706));
#25585=CARTESIAN_POINT('Ctrl Pts',(-2.87956461201735,-2.59845889517359,
-3.46367643972069));
#25586=CARTESIAN_POINT('Ctrl Pts',(-2.76084640205531,1.48857849723153,-4.06610098148393));
#25587=CARTESIAN_POINT('Ctrl Pts',(-2.64212819209327,4.22059972201472,-0.967254419370101));
#25588=CARTESIAN_POINT('Ctrl Pts',(-2.52340998213123,3.1107134663514,3.01205990206451));
#25589=CARTESIAN_POINT('Ctrl Pts',(-2.40469177216919,-0.830778276959734,
4.24957063494798));
#25590=CARTESIAN_POINT('Ctrl Pts',(-2.28597356220715,-4.01603311405792,
1.6188023820654));
#25591=CARTESIAN_POINT('Ctrl Pts',(-2.16725535224512,-3.54559239183993,
-2.4855216185338));
#25592=CARTESIAN_POINT('Ctrl Pts',(-2.04853714228307,0.152313342141281,
-4.32733679895125));
#25593=CARTESIAN_POINT('Ctrl Pts',(-1.92981893232104,3.711572010072,-2.23008437947081));
#25594=CARTESIAN_POINT('Ctrl Pts',(-1.811100722359,3.89227852721326,1.89715866287202));
#25595=CARTESIAN_POINT('Ctrl Pts',(-1.69238251239696,0.529940222952991,
4.29746512326462));
#25596=CARTESIAN_POINT('Ctrl Pts',(-1.57366430243492,-3.31478955187358,
2.78589543097564));
#25597=CARTESIAN_POINT('Ctrl Pts',(-1.45494609247288,-4.14214842847016,
-1.26160592978457));
#25598=CARTESIAN_POINT('Ctrl Pts',(-1.33622788251084,-1.19901209605891,
-4.16069863352995));
#25599=CARTESIAN_POINT('Ctrl Pts',(-1.2175096725488,2.83555527553512,-3.27241033565973));
#25600=CARTESIAN_POINT('Ctrl Pts',(-1.09879146258676,4.28898685107728,0.594672108674195));
#25601=CARTESIAN_POINT('Ctrl Pts',(-0.980073252624725,1.83825983531098,
3.92043924878734));
#25602=CARTESIAN_POINT('Ctrl Pts',(-0.861355042662685,-2.28578961726445,
3.67752755953711));
#25603=CARTESIAN_POINT('Ctrl Pts',(-0.742636832700648,-4.32914134750355,
0.0870535403315232));
#25604=CARTESIAN_POINT('Ctrl Pts',(-0.623918622738608,-2.43178284203752,
-3.58266316233067));
#25605=CARTESIAN_POINT('Ctrl Pts',(-0.505200412776569,1.67916740539267,
-3.99117024821242));
#25606=CARTESIAN_POINT('Ctrl Pts',(-0.38648220281453,4.2616131179203,-0.766613826329018));
#25607=CARTESIAN_POINT('Ctrl Pts',(-0.267763992852492,2.96481787101653,
3.15577219032842));
#25608=CARTESIAN_POINT('Ctrl Pts',(-0.149045782890452,-1.03077771375419,
4.20553687778111));
#25609=CARTESIAN_POINT('Ctrl Pts',(-0.0303275729284135,-4.08808185427113,
1.42710541948671));
#25610=CARTESIAN_POINT('Ctrl Pts',(0.0883906370336247,-3.42410625029169,
-2.65038478569859));
#25611=CARTESIAN_POINT('Ctrl Pts',(0.207108846995665,0.356748537234746,
-4.31529530933053));
#25612=CARTESIAN_POINT('Ctrl Pts',(0.325827056957703,3.81286395974495,-2.05209930315938));
#25613=CARTESIAN_POINT('Ctrl Pts',(0.444545266919742,3.79822367634993,2.07907191553442));
#25614=CARTESIAN_POINT('Ctrl Pts',(0.56326347688178,0.326154374722222,4.31771542014972));
#25615=CARTESIAN_POINT('Ctrl Pts',(0.68198168684382,-3.44280518289795,2.62604942797354));
#25616=CARTESIAN_POINT('Ctrl Pts',(0.800699896805859,-4.0778643813607,-1.45604437184413));
#25617=CARTESIAN_POINT('Ctrl Pts',(0.919418106767897,-1.00094454806639,
-4.21273701258996));
#25618=CARTESIAN_POINT('Ctrl Pts',(1.03813631672994,2.98711033703512,-3.13467940305337));
#25619=CARTESIAN_POINT('Ctrl Pts',(1.15685452669198,4.25607260412292,0.796799293413037));
#25620=CARTESIAN_POINT('Ctrl Pts',(1.27557273665401,1.6508373043784,4.0029713114163));
#25621=CARTESIAN_POINT('Ctrl Pts',(1.39429094661605,-2.45711434039823,3.56533760585987));
#25622=CARTESIAN_POINT('Ctrl Pts',(1.51300915657809,-4.32841560712957,-0.117734691175787));
#25623=CARTESIAN_POINT('Ctrl Pts',(1.63172736654013,-2.25966726165839,-3.69363601240545));
#25624=CARTESIAN_POINT('Ctrl Pts',(1.75044557650217,1.86600027228884,-3.90731187766823));
#25625=CARTESIAN_POINT('Ctrl Pts',(1.86916378646421,4.29309393613648,-0.564258434635544));
#25626=CARTESIAN_POINT('Ctrl Pts',(1.98788199642625,2.8122904307839,3.29242549778585));
#25627=CARTESIAN_POINT('Ctrl Pts',(2.10660020638829,-1.22847145817667,4.1520959769729));
#25628=CARTESIAN_POINT('Ctrl Pts',(2.22531841635032,-4.15098617964756,1.23221623992068));
#25629=CARTESIAN_POINT('Ctrl Pts',(2.34403662631236,-3.29496090592035,-2.80931944677098));
#25630=CARTESIAN_POINT('Ctrl Pts',(2.4627548362744,0.560385740322455,-4.29360116307888));
#25631=CARTESIAN_POINT('Ctrl Pts',(2.58147304623644,3.90562711497251,-1.86952399405324));
#25632=CARTESIAN_POINT('Ctrl Pts',(2.70019125619848,3.69567277911633,2.25633460179288));
#25633=CARTESIAN_POINT('Ctrl Pts',(2.81890946616052,0.12163896896003,4.32830764696543));
#25634=CARTESIAN_POINT('Ctrl Pts',(2.93762767612256,-3.56311978445035,2.4603293534012));
#25635=CARTESIAN_POINT('Ctrl Pts',(3.05634588608459,-4.00445877432637,-1.64722586498323));
#25636=CARTESIAN_POINT('Ctrl Pts',(3.17506409604664,-0.800638039965777,
-4.25535214224499));
#25637=CARTESIAN_POINT('Ctrl Pts',(3.29378230600867,3.13198368884777,-2.98993667129265));
#25638=CARTESIAN_POINT('Ctrl Pts',(3.41250051597072,4.2136381726622,0.99714415980492));
#25639=CARTESIAN_POINT('Ctrl Pts',(3.53121872593275,1.45972210248142,4.07654933848181));
#25640=CARTESIAN_POINT('Ctrl Pts',(3.64993693589479,-2.62294287395784,3.44517253639104));
#25641=CARTESIAN_POINT('Ctrl Pts',(3.76865514585683,-4.31800786199842,-0.322259568157221));
#25642=CARTESIAN_POINT('Ctrl Pts',(3.88737335581887,-2.08249715066972,-3.79634676274463));
#25643=CARTESIAN_POINT('Ctrl Pts',(4.0060915657809,2.04865918151714,-3.81471344710645));
#25644=CARTESIAN_POINT('Ctrl Pts',(4.12480977574295,4.31497175877985,-0.360640882986961));
#25645=CARTESIAN_POINT('Ctrl Pts',(4.24352798570498,2.65347232629884,3.4217141521634));
#25646=CARTESIAN_POINT('Ctrl Pts',(4.36224619566703,-1.42341729953675,4.08936747149588));
#25647=CARTESIAN_POINT('Ctrl Pts',(4.48096440562906,-4.20460538280232,1.03457078078738));
#25648=CARTESIAN_POINT('Ctrl Pts',(4.59968261559111,-3.15844523714832,-2.96197008922851));
#25649=CARTESIAN_POINT('Ctrl Pts',(4.71840082555314,0.762769446080897,-4.2623028866652));
#25650=CARTESIAN_POINT('Ctrl Pts',(4.83711903551519,3.98965397873934,-1.68276684525171));
#25651=CARTESIAN_POINT('Ctrl Pts',(4.95583724547721,3.58485522621101,2.42855021209299));
#25652=CARTESIAN_POINT('Ctrl Pts',(5.07455545543927,-0.0831485246012159,
4.32921811051441));
#25653=CARTESIAN_POINT('Ctrl Pts',(5.19327366540129,-3.67546423113905,2.2891058977615));
#25654=CARTESIAN_POINT('Ctrl Pts',(5.31199187536334,-3.92209580450113,-1.83472276539637));
#25655=CARTESIAN_POINT('Ctrl Pts',(5.43071008532537,-0.598540626828496,
-4.28844869895689));
#25656=CARTESIAN_POINT('Ctrl Pts',(5.54942829528742,3.26985127140738,-2.83850590776641));
#25657=CARTESIAN_POINT('Ctrl Pts',(5.66814650524945,4.16177847603852,1.19525856697685));
#25658=CARTESIAN_POINT('Ctrl Pts',(5.78686471521149,1.2653417251431,4.14100874717272));
#25659=CARTESIAN_POINT('Ctrl Pts',(5.90558292517353,-2.78290428483595,3.31730114204168));
#25660=CARTESIAN_POINT('Ctrl Pts',(6.02430113513557,-4.29794139264672,-0.526063599694207));
#25661=CARTESIAN_POINT('Ctrl Pts',(6.1430193450976,-1.90066881155562,-3.89056566508378));
#25662=CARTESIAN_POINT('Ctrl Pts',(6.26173755505965,2.2267355529899,-3.71358208507633));
#25663=CARTESIAN_POINT('Ctrl Pts',(6.38045576502168,4.3271976485019,-0.156216632753608));
#25664=CARTESIAN_POINT('Ctrl Pts',(6.49917397498373,2.48871880940937,3.54334895448378));
#25665=CARTESIAN_POINT('Ctrl Pts',(6.61789218494576,-1.61517917375591,4.01749167543808));
#25666=CARTESIAN_POINT('Ctrl Pts',(6.7366103949078,-4.24881952576571,0.834611144798058));
#25667=CARTESIAN_POINT('Ctrl Pts',(6.85532860486984,-3.01486460868043,-3.10799525689398));
#25668=CARTESIAN_POINT('Ctrl Pts',(6.97404681483187,0.963446953064535,-4.22147048955455));
#25669=CARTESIAN_POINT('Ctrl Pts',(7.09276502479393,4.06475659578232,-1.4922456039785));
#25670=CARTESIAN_POINT('Ctrl Pts',(7.21148323475594,3.46601889957775,2.59533352641215));
#25671=CARTESIAN_POINT('Ctrl Pts',(7.33020144471801,-0.287750027609826,
4.32044477422867));
#25672=CARTESIAN_POINT('Ctrl Pts',(7.44891965468002,-3.77958722559195,2.1127620617787));
#25673=CARTESIAN_POINT('Ctrl Pts',(7.56763786464209,-3.83095970527152,-2.01811567114847));
#25674=CARTESIAN_POINT('Ctrl Pts',(7.6863560746041,-0.395104369707096,-4.31195265078218));
#25675=CARTESIAN_POINT('Ctrl Pts',(7.80507428456616,3.40040469598434,-2.68072583996889));
#25676=CARTESIAN_POINT('Ctrl Pts',(7.92379249452818,4.10060951647421,1.39069936325232));
#25677=CARTESIAN_POINT('Ctrl Pts',(8.04251070449023,1.06813097158531,4.19620535163489));
#25678=CARTESIAN_POINT('Ctrl Pts',(8.16122891445227,-2.93664076378281,3.18200945159473));
#25679=CARTESIAN_POINT('Ctrl Pts',(8.2799471244143,-4.26826108470218,-0.728690907289412));
#25680=CARTESIAN_POINT('Ctrl Pts',(8.39866533437635,-1.71458896654529,-3.97608196612575));
#25681=CARTESIAN_POINT('Ctrl Pts',(8.51738354433838,2.39983105705674,-3.60414400699182));
#25682=CARTESIAN_POINT('Ctrl Pts',(8.63610175430043,4.32974425785424,0.0485570502327038));
#25683=CARTESIAN_POINT('Ctrl Pts',(8.75481996426246,2.31839840857459,3.65705782626801));
#25684=CARTESIAN_POINT('Ctrl Pts',(8.8735381742245,-1.8033281388038,3.93662936397977));
#25685=CARTESIAN_POINT('Ctrl Pts',(8.99225638418654,-4.28352970825152,0.63278461112424));
#25686=CARTESIAN_POINT('Ctrl Pts',(9.11097459414858,-2.86454018845754,-3.24706831376562));
#25687=CARTESIAN_POINT('Ctrl Pts',(9.22969280411062,1.16196937633404,-4.17119530758405));
#25688=CARTESIAN_POINT('Ctrl Pts',(9.34841101407265,4.13076697301538,-1.29838643715753));
#25689=CARTESIAN_POINT('Ctrl Pts',(9.4671292240347,3.33942961793276,2.75631147594436));
#25690=CARTESIAN_POINT('Ctrl Pts',(9.58584743399673,-0.491707877746567,
4.30200726272179));
#25691=CARTESIAN_POINT('Ctrl Pts',(9.70456564395877,-3.8752558605702,1.93169229968585));
#25692=CARTESIAN_POINT('Ctrl Pts',(9.82328385392082,-3.73125433417492,-2.19699436031369));
#25693=CARTESIAN_POINT('Ctrl Pts',(9.94200206388284,-0.190784324443694,
-4.32581142296975));
#25694=CARTESIAN_POINT('Ctrl Pts',(10.0607202738449,3.52335193450366,-2.51694939781845));
#25695=CARTESIAN_POINT('Ctrl Pts',(10.1794384838069,4.03026811959114,1.58302937741427));
#25696=CARTESIAN_POINT('Ctrl Pts',(10.298156693769,0.868530972149402,4.24201568549269));
#25697=CARTESIAN_POINT('Ctrl Pts',(10.416874903731,-3.0838084257709,3.03960009190256));
#25698=CARTESIAN_POINT('Ctrl Pts',(10.5355931136931,-4.22903332848136,-0.929688244597408));
#25699=CARTESIAN_POINT('Ctrl Pts',(10.6543113236551,-1.5246738478374,-4.05270437896332));
#25700=CARTESIAN_POINT('Ctrl Pts',(10.7730295336171,2.56755850550722,-3.4866440091227));
#25701=CARTESIAN_POINT('Ctrl Pts',(10.8917477435791,4.32260589046018,0.253222118513249));
#25702=CARTESIAN_POINT('Ctrl Pts',(11.0104659535412,2.14289210452383,3.76258641813191));
#25703=CARTESIAN_POINT('Ctrl Pts',(11.1291841635032,-1.98744333417803,3.84696141376681));
#25704=CARTESIAN_POINT('Ctrl Pts',(11.2479023734653,-4.30865828887852,0.429542634896841));
#25705=CARTESIAN_POINT('Ctrl Pts',(11.3666205834273,-2.70780822925922,-3.37887817464105));
#25706=CARTESIAN_POINT('Ctrl Pts',(11.4853387933894,1.35789265155523,-4.11158979867935));
#25707=CARTESIAN_POINT('Ctrl Pts',(11.6040570033514,4.18753745528177,-1.10162297810297));
#25708=CARTESIAN_POINT('Ctrl Pts',(11.7227752133134,3.20537054221196,2.91112397752316));
#25709=CARTESIAN_POINT('Ctrl Pts',(11.8414934232755,-0.694565852527616,
4.27394681803398));
#25710=CARTESIAN_POINT('Ctrl Pts',(11.9602116332375,-3.96225613978983,1.7463016366203));
#25711=CARTESIAN_POINT('Ctrl Pts',(12.0789298431995,-3.62320271719853,-2.37095870806454));
#25712=CARTESIAN_POINT('Ctrl Pts',(12.1976480531616,0.0139624767857471,
-4.32999401654167));
#25713=CARTESIAN_POINT('Ctrl Pts',(12.3163662631236,3.63841797169183,-2.34754292234513));
#25714=CARTESIAN_POINT('Ctrl Pts',(12.4350844730857,3.9509116303975,1.77181839304862));
#25715=CARTESIAN_POINT('Ctrl Pts',(12.5538026830477,0.66698819766677,4.2783372847593));
#25716=CARTESIAN_POINT('Ctrl Pts',(12.6725208930098,-3.22407807181873,2.89039159814913));
#25717=CARTESIAN_POINT('Ctrl Pts',(12.7912391029718,-4.18034588454684,-1.12860598691075));
#25718=CARTESIAN_POINT('Ctrl Pts',(12.9099573129338,-1.33134823980997,-4.12026155727892));
#25719=CARTESIAN_POINT('Ctrl Pts',(13.0286755228959,2.72954266679506,-3.36134483293444));
#25720=CARTESIAN_POINT('Ctrl Pts',(13.1473937328579,4.30579861047257,0.457320600064824));
#25721=CARTESIAN_POINT('Ctrl Pts',(13.2661119428199,1.96259229413334,3.85969899730394));
#25722=CARTESIAN_POINT('Ctrl Pts',(13.384830152782,-2.16711257252377,3.74868779246955));
#25723=CARTESIAN_POINT('Ctrl Pts',(13.503548362744,-4.32414972403095,0.225340989528843));
#25724=CARTESIAN_POINT('Ctrl Pts',(13.6222665727061,-2.54501805154884,-3.50313219206192));
#25725=CARTESIAN_POINT('Ctrl Pts',(13.7409847826681,1.55077612259861,-4.04278312443387));
#25726=CARTESIAN_POINT('Ctrl Pts',(13.8597029926301,4.23494563063579,-0.902403280807197));
#25727=CARTESIAN_POINT('Ctrl Pts',(13.9784212025922,3.0641328417704,3.05943980887305));
#25728=CARTESIAN_POINT('Ctrl Pts',(14.0971394125542,-0.895853643967219,
4.23629754868133));
#25729=CARTESIAN_POINT('Ctrl Pts',(14.2158576225162,-4.04042492235024,1.55705926385799));
#25730=CARTESIAN_POINT('Ctrl Pts',(14.3345758324783,-3.50698671018115,-2.53972322927799));
#25731=CARTESIAN_POINT('Ctrl Pts',(14.4532940424403,0.218564245614825,-4.32429395921576));
#25732=CARTESIAN_POINT('Ctrl Pts',(14.5720122524024,3.74556186860945,-2.17326028708754));
#25733=CARTESIAN_POINT('Ctrl Pts',(14.6907304623644,3.86230569986296,1.95735778972818));
#25734=CARTESIAN_POINT('Ctrl Pts',(14.8094486723264,0.464738727873276,4.30372617863017));
#25735=CARTESIAN_POINT('Ctrl Pts',(14.9281668822885,-3.35864660907939,2.73735654780123));
#25736=CARTESIAN_POINT('Ctrl Pts',(15.0468850922505,-4.11928555052006,-1.33042058350709));
#25737=CARTESIAN_POINT('Ctrl Pts',(15.1260305655586,-2.13452904287985,-3.22024104752762));
#25738=CARTESIAN_POINT('Ctrl Pts',(15.1656033022126,-0.961289160296659,
-3.53893126683851));
#25739=CARTESIAN_POINT('Ctrl Pts',(-5.646,2.04569608541839,-2.86913603522103));
#25740=CARTESIAN_POINT('Ctrl Pts',(-5.60642726334599,2.99688291874876,-2.19093912940735));
#25741=CARTESIAN_POINT('Ctrl Pts',(-5.52728179003796,4.15588292084424,0.17368053733326));
#25742=CARTESIAN_POINT('Ctrl Pts',(-5.40856358007592,2.11478894550069,3.58630724545133));
#25743=CARTESIAN_POINT('Ctrl Pts',(-5.28984537011388,-1.85304107076213,
3.72388412481386));
#25744=CARTESIAN_POINT('Ctrl Pts',(-5.17112716015185,-4.13320183070728,
0.476987007469099));
#25745=CARTESIAN_POINT('Ctrl Pts',(-5.0524089501898,-2.65148029460583,-3.20684990304941));
#25746=CARTESIAN_POINT('Ctrl Pts',(-4.93369074022778,1.24406479104381,-3.9701278679622));
#25747=CARTESIAN_POINT('Ctrl Pts',(-4.81497253026572,4.0070387833704,-1.12025498671569));
#25748=CARTESIAN_POINT('Ctrl Pts',(-4.69625432030369,3.12257273473017,2.74975698427391));
#25749=CARTESIAN_POINT('Ctrl Pts',(-4.57753611034165,-0.604329863247786,
4.116523575551));
#25750=CARTESIAN_POINT('Ctrl Pts',(-4.45881790037961,-3.78110708392794,
1.73623086576801));
#25751=CARTESIAN_POINT('Ctrl Pts',(-4.34009969041758,-3.51604601315693,
-2.22456780215962));
#25752=CARTESIAN_POINT('Ctrl Pts',(-4.22138148045554,-0.0504100535793502,
-4.16036696958348));
#25753=CARTESIAN_POINT('Ctrl Pts',(-4.10266327049349,3.46111018837926,-2.30910306912985));
#25754=CARTESIAN_POINT('Ctrl Pts',(-3.98394506053146,3.82206891947539,1.64408864020745));
#25755=CARTESIAN_POINT('Ctrl Pts',(-3.86522685056942,0.703892139470341,
4.1007027146119));
#25756=CARTESIAN_POINT('Ctrl Pts',(-3.74650864060738,-3.05501983726778,
2.82455091812984));
#25757=CARTESIAN_POINT('Ctrl Pts',(-3.62779043064534,-4.03302306811295,
-1.02272090561931));
#25758=CARTESIAN_POINT('Ctrl Pts',(-3.5090722206833,-1.33986509473402,-3.93903455379817));
#25759=CARTESIAN_POINT('Ctrl Pts',(-3.39035401072126,2.57293885887897,-3.26974286547831));
#25760=CARTESIAN_POINT('Ctrl Pts',(-3.27163580075922,4.14366027205377,0.375915015385937));
#25761=CARTESIAN_POINT('Ctrl Pts',(-3.15291759079718,1.94251026639215,3.67938666679367));
#25762=CARTESIAN_POINT('Ctrl Pts',(-3.03419938083515,-2.0268587551866,3.63360373818345));
#25763=CARTESIAN_POINT('Ctrl Pts',(-2.9154811708731,-4.15122841486805,0.280241221310659));
#25764=CARTESIAN_POINT('Ctrl Pts',(-2.79676296091107,-2.4968375762945,-3.32821793059103));
#25765=CARTESIAN_POINT('Ctrl Pts',(-2.67804475094903,1.43036271770746,-3.90708267059147));
#25766=CARTESIAN_POINT('Ctrl Pts',(-2.55932654098699,4.05553922750062,-0.929426740059659));
#25767=CARTESIAN_POINT('Ctrl Pts',(-2.44060833102495,2.9890587402779,2.89426334951592));
#25768=CARTESIAN_POINT('Ctrl Pts',(-2.32189012106291,-0.798287948035305,
4.08337713718073));
#25769=CARTESIAN_POINT('Ctrl Pts',(-2.20317191110087,-3.858972872516,1.55549376734164));
#25770=CARTESIAN_POINT('Ctrl Pts',(-2.08445370113884,-3.40693028880043,
-2.38831708493618));
#25771=CARTESIAN_POINT('Ctrl Pts',(-1.96573549117679,0.14635662574293,-4.15810199844688));
#25772=CARTESIAN_POINT('Ctrl Pts',(-1.84701728121476,3.56641872576227,-2.14286956292151));
#25773=CARTESIAN_POINT('Ctrl Pts',(-1.72829907125272,3.74005811760244,1.82296400626149));
#25774=CARTESIAN_POINT('Ctrl Pts',(-1.60958086129068,0.509215159922919,
4.12939855331646));
#25775=CARTESIAN_POINT('Ctrl Pts',(-1.49086265132864,-3.18515375632809,
2.67694378718369));
#25776=CARTESIAN_POINT('Ctrl Pts',(-1.3721444413666,-3.98015603094717,-1.21226666229469));
#25777=CARTESIAN_POINT('Ctrl Pts',(-1.25342623140456,-1.15212076721019,
-3.99798076895909));
#25778=CARTESIAN_POINT('Ctrl Pts',(-1.13470802144252,2.72466151947467,-3.14443191936036));
#25779=CARTESIAN_POINT('Ctrl Pts',(-1.01598981148048,4.12125185197025,0.571415491416797));
#25780=CARTESIAN_POINT('Ctrl Pts',(-0.897271601518446,1.76636861191941,
3.76711752113286));
#25781=CARTESIAN_POINT('Ctrl Pts',(-0.778553391556407,-2.19639626337378,
3.53370569592844));
#25782=CARTESIAN_POINT('Ctrl Pts',(-0.659835181594368,-4.15983597416688,
0.083649024063062));
#25783=CARTESIAN_POINT('Ctrl Pts',(-0.541116971632329,-2.33667994081619,
-3.44255128435104));
#25784=CARTESIAN_POINT('Ctrl Pts',(-0.422398761670289,1.61349801702105,
-3.83508235117171));
#25785=CARTESIAN_POINT('Ctrl Pts',(-0.303680551708251,4.09494865907512,
-0.736632860208229));
#25786=CARTESIAN_POINT('Ctrl Pts',(-0.184962341746212,2.84886887415203,
3.0323552940062));
#25787=CARTESIAN_POINT('Ctrl Pts',(-0.0662441317841732,-0.990465746173143,
4.04106546554956));
#25788=CARTESIAN_POINT('Ctrl Pts',(0.0524740781778656,-3.92820390873641,
1.37129374773886));
#25789=CARTESIAN_POINT('Ctrl Pts',(0.171192288139904,-3.29019526413636,
-2.54673273333783));
#25790=CARTESIAN_POINT('Ctrl Pts',(0.289910498101944,0.342796707198351,
-4.1465314310558));
#25791=CARTESIAN_POINT('Ctrl Pts',(0.408628708063982,3.66374931913409,-1.97184518097748));
#25792=CARTESIAN_POINT('Ctrl Pts',(0.52734691802602,3.64968159238416,1.99776294024389));
#25793=CARTESIAN_POINT('Ctrl Pts',(0.64606512798806,0.313399030476065,4.14885689544678));
#25794=CARTESIAN_POINT('Ctrl Pts',(0.764783337950098,-3.30816291321273,
2.52334909016639));
#25795=CARTESIAN_POINT('Ctrl Pts',(0.883501547912138,-3.91838602385669,
-1.399100946767));
#25796=CARTESIAN_POINT('Ctrl Pts',(1.00221975787418,-0.961799304980866,
-4.04798401530169));
#25797=CARTESIAN_POINT('Ctrl Pts',(1.12093796783622,2.87028951964572,-3.01208740985575));
#25798=CARTESIAN_POINT('Ctrl Pts',(1.23965617779825,4.0896248253724,0.765637824886821));
#25799=CARTESIAN_POINT('Ctrl Pts',(1.35837438776029,1.586275858193,3.84642189481521));
#25800=CARTESIAN_POINT('Ctrl Pts',(1.47709259772233,-2.36102076725307,3.42590330099951));
#25801=CARTESIAN_POINT('Ctrl Pts',(1.59581080768437,-4.15913861626764,-0.11313028715101));
#25802=CARTESIAN_POINT('Ctrl Pts',(1.71452901764641,-2.17129550877666,-3.54918417453448));
#25803=CARTESIAN_POINT('Ctrl Pts',(1.83324722760845,1.7930241674711,-3.7545035392265));
#25804=CARTESIAN_POINT('Ctrl Pts',(1.95196543757049,4.12519831590081,-0.54219124457039));
#25805=CARTESIAN_POINT('Ctrl Pts',(2.07068364753253,2.70230652333086,3.16366432245317));
#25806=CARTESIAN_POINT('Ctrl Pts',(2.18940185749457,-1.18042802365586,3.98971454770484));
#25807=CARTESIAN_POINT('Ctrl Pts',(2.3081200674566,-3.98864815267002,1.18402635333924));
#25808=CARTESIAN_POINT('Ctrl Pts',(2.42683827741864,-3.16610057507709,-2.69945172946213));
#25809=CARTESIAN_POINT('Ctrl Pts',(2.54555648738068,0.538470004761492,-4.12568570605805));
#25810=CARTESIAN_POINT('Ctrl Pts',(2.66427469734272,3.75288466474145,-1.79641008245562));
#25811=CARTESIAN_POINT('Ctrl Pts',(2.78299290730476,3.55114128675486,2.16809318358432));
#25812=CARTESIAN_POINT('Ctrl Pts',(2.9017111172668,0.116881875255089,4.15903487824236));
#25813=CARTESIAN_POINT('Ctrl Pts',(3.02042932722884,-3.42377221482258,2.36411004655206));
#25814=CARTESIAN_POINT('Ctrl Pts',(3.13914753719088,-3.8478511855745,-1.58280565606543));
#25815=CARTESIAN_POINT('Ctrl Pts',(3.25786574715292,-0.769326444574681,
-4.08893253953619));
#25816=CARTESIAN_POINT('Ctrl Pts',(3.37658395711495,3.0094971204592,-2.87300532076558));
#25817=CARTESIAN_POINT('Ctrl Pts',(3.495302167077,4.04884993253241,0.958147543456581));
#25818=CARTESIAN_POINT('Ctrl Pts',(3.61402037703903,1.40263484759868,3.9171224100737));
#25819=CARTESIAN_POINT('Ctrl Pts',(3.73273858700107,-2.52036402820767,3.31043768352714));
#25820=CARTESIAN_POINT('Ctrl Pts',(3.8514567969631,-4.14913790039093,-0.309656543187913));
#25821=CARTESIAN_POINT('Ctrl Pts',(3.97017500692515,-2.00105422024427,-3.6478780816856));
#25822=CARTESIAN_POINT('Ctrl Pts',(4.08889321688719,1.96853959665618,-3.66552647618271));
#25823=CARTESIAN_POINT('Ctrl Pts',(4.20761142684923,4.14622053401822,-0.346536829911929));
#25824=CARTESIAN_POINT('Ctrl Pts',(4.32632963681127,2.54969952546351,3.28789671690745));
#25825=CARTESIAN_POINT('Ctrl Pts',(4.4450478467733,-1.3677498639029,3.92943924765267));
#25826=CARTESIAN_POINT('Ctrl Pts',(4.56376605673535,-4.04017039975903,0.994110472789965));
#25827=CARTESIAN_POINT('Ctrl Pts',(4.68248426669738,-3.03492380250006,-2.84613246427821));
#25828=CARTESIAN_POINT('Ctrl Pts',(4.80120247665942,0.732938827149255,-4.09561145213467));
#25829=CARTESIAN_POINT('Ctrl Pts',(4.91992068662146,3.83362538042524,-1.61695668889399));
#25830=CARTESIAN_POINT('Ctrl Pts',(5.0386388965835,3.44465762033206,2.33357373354433));
#25831=CARTESIAN_POINT('Ctrl Pts',(5.15735710654553,-0.0798967268727354,
4.15990973510661));
#25832=CARTESIAN_POINT('Ctrl Pts',(5.27607531650758,-3.5317230608034,2.19958284976698));
#25833=CARTESIAN_POINT('Ctrl Pts',(5.39479352646961,-3.76870929176318,-1.76296987080819));
#25834=CARTESIAN_POINT('Ctrl Pts',(5.51351173643166,-0.575132718389392,
-4.12073474606626));
#25835=CARTESIAN_POINT('Ctrl Pts',(5.63222994639369,3.14197293576922,-2.72749675748542));
#25836=CARTESIAN_POINT('Ctrl Pts',(5.75094815635573,3.99901838065921,1.14851403228232));
#25837=CARTESIAN_POINT('Ctrl Pts',(5.86966636631777,1.21585635703487,3.97906092065169));
#25838=CARTESIAN_POINT('Ctrl Pts',(5.98838457627981,-2.67406961969476,3.18756712246586));
#25839=CARTESIAN_POINT('Ctrl Pts',(6.10710278624185,-4.12985619661107,-0.505490144822725));
#25840=CARTESIAN_POINT('Ctrl Pts',(6.22582099620389,-1.82633687898537,-3.73841224260482));
#25841=CARTESIAN_POINT('Ctrl Pts',(6.34453920616593,2.13965170336266,-3.56835019014346));
#25842=CARTESIAN_POINT('Ctrl Pts',(6.46325741612797,4.15796828993553,-0.15010726528171));
#25843=CARTESIAN_POINT('Ctrl Pts',(6.58197562609,2.39138923910093,3.40477458847308));
#25844=CARTESIAN_POINT('Ctrl Pts',(6.70069383605204,-1.55201225656202,3.86037439203516));
#25845=CARTESIAN_POINT('Ctrl Pts',(6.81941204601408,-4.08265540260426,0.801970918915297));
#25846=CARTESIAN_POINT('Ctrl Pts',(6.93813025597612,-2.89695836881454,-2.98644683538066));
#25847=CARTESIAN_POINT('Ctrl Pts',(7.05684846593816,0.925768177301577,-4.05637594079931));
#25848=CARTESIAN_POINT('Ctrl Pts',(7.1755666759002,3.90579086153378,-1.43388641013115));
#25849=CARTESIAN_POINT('Ctrl Pts',(7.29428488586224,3.33046878081729,2.49383443540284));
#25850=CARTESIAN_POINT('Ctrl Pts',(7.41300309582428,-0.276496612222895,
4.15147950911829));
#25851=CARTESIAN_POINT('Ctrl Pts',(7.53172130578631,-3.63177398159695,2.03013552202684));
#25852=CARTESIAN_POINT('Ctrl Pts',(7.65043951574835,-3.68113737075413,-1.93919059115831));
#25853=CARTESIAN_POINT('Ctrl Pts',(7.76915772571038,-0.379652508136737,
-4.14331949821216));
#25854=CARTESIAN_POINT('Ctrl Pts',(7.88787593567244,3.26742063740621,-2.57588720045187));
#25855=CARTESIAN_POINT('Ctrl Pts',(8.00659414563445,3.940241635325,1.33631147059774));
#25856=CARTESIAN_POINT('Ctrl Pts',(8.12531235559652,1.02635818146356,4.03209887955918));
#25857=CARTESIAN_POINT('Ctrl Pts',(8.24403056555854,-2.82179372577729,3.0575664604982));
#25858=CARTESIAN_POINT('Ctrl Pts',(8.36274877552059,-4.10133663515502,-0.700193042192699));
#25859=CARTESIAN_POINT('Ctrl Pts',(8.48146698548262,-1.64753430101277,-3.82058414619887));
#25860=CARTESIAN_POINT('Ctrl Pts',(8.60018519544467,2.305977735937,-3.46319204962163));
#25861=CARTESIAN_POINT('Ctrl Pts',(8.7189034054067,4.16041530571664,0.0466580663793381));
#25862=CARTESIAN_POINT('Ctrl Pts',(8.83762161536874,2.22772978017945,3.5140364991988));
#25863=CARTESIAN_POINT('Ctrl Pts',(8.95633982533078,-1.73280303479793,3.78267446838806));
#25864=CARTESIAN_POINT('Ctrl Pts',(9.07505803529282,-4.11600812874189,0.608037478557221));
#25865=CARTESIAN_POINT('Ctrl Pts',(9.19377624525485,-2.75251288162813,-3.12008098094757));
#25866=CARTESIAN_POINT('Ctrl Pts',(9.31249445521691,1.11652672540754,-4.00806693589946));
#25867=CARTESIAN_POINT('Ctrl Pts',(9.43121266517893,3.96921968490559,-1.24760874642564));
#25868=CARTESIAN_POINT('Ctrl Pts',(9.54993087514098,3.20883019120772,2.64851681044191));
#25869=CARTESIAN_POINT('Ctrl Pts',(9.66864908510301,-0.472478016872994,
4.1337630574056));
#25870=CARTESIAN_POINT('Ctrl Pts',(9.78736729506506,-3.72370117857135,1.85614709112886));
#25871=CARTESIAN_POINT('Ctrl Pts',(9.90608550502709,-3.58533130756231,-2.11107363827349));
#25872=CARTESIAN_POINT('Ctrl Pts',(10.0248037149891,-0.183323073196887,
-4.15663627733209));
#25873=CARTESIAN_POINT('Ctrl Pts',(10.1435219249512,3.3855596180177,-2.41851577709298));
#25874=CARTESIAN_POINT('Ctrl Pts',(10.2622401349132,3.87265117113374,1.52111978421037));
#25875=CARTESIAN_POINT('Ctrl Pts',(10.3809583448753,0.834564199366861,4.07611764898101));
#25876=CARTESIAN_POINT('Ctrl Pts',(10.4996765548373,-2.96320591018775,2.92072648925374));
#25877=CARTESIAN_POINT('Ctrl Pts',(10.6183947647993,-4.0636430099267,-0.893329714648016));
#25878=CARTESIAN_POINT('Ctrl Pts',(10.7371129747614,-1.46504644039007,-3.89420998646693));
#25879=CARTESIAN_POINT('Ctrl Pts',(10.8558311847234,2.46714564844276,-3.35028727732022));
#25880=CARTESIAN_POINT('Ctrl Pts',(10.9745493946854,4.1535561077605,0.243319031071492));
#25881=CARTESIAN_POINT('Ctrl Pts',(11.0932676046475,2.05908722991844,3.61543804687332));
#25882=CARTESIAN_POINT('Ctrl Pts',(11.2119858146095,-1.90971779724849,3.69651327957846));
#25883=CARTESIAN_POINT('Ctrl Pts',(11.3307040245716,-4.14015397321339,0.412743951202418));
#25884=CARTESIAN_POINT('Ctrl Pts',(11.4494222345336,-2.60191044344467,-3.24673598179103));
#25885=CARTESIAN_POINT('Ctrl Pts',(11.5681404444956,1.30478777373567,-3.9507924973221));
#25886=CARTESIAN_POINT('Ctrl Pts',(11.6868586544577,4.02376996992659,-1.05854037242841));
#25887=CARTESIAN_POINT('Ctrl Pts',(11.8055768644197,3.0800139384955,2.79727485773682));
#25888=CARTESIAN_POINT('Ctrl Pts',(11.9242950743818,-0.66740256042652,4.10680000910255));
#25889=CARTESIAN_POINT('Ctrl Pts',(12.0430132843438,-3.80729902447422,1.67800674236445));
#25890=CARTESIAN_POINT('Ctrl Pts',(12.1617314943058,-3.48150540600691,-2.27823453552944));
#25891=CARTESIAN_POINT('Ctrl Pts',(12.2804497042679,0.0134164280071953,
-4.16065529676554));
#25892=CARTESIAN_POINT('Ctrl Pts',(12.3991679142299,3.49612561771096,-2.25573450146264));
#25893=CARTESIAN_POINT('Ctrl Pts',(12.5178861241919,3.79639817959729,1.70252558174023));
#25894=CARTESIAN_POINT('Ctrl Pts',(12.636604334154,0.640903420859428,4.11101877212304));
#25895=CARTESIAN_POINT('Ctrl Pts',(12.755322544116,-3.09798984835828,2.77735328654585));
#25896=CARTESIAN_POINT('Ctrl Pts',(12.8740407540781,-4.01685964932199,-1.08446812154071));
#25897=CARTESIAN_POINT('Ctrl Pts',(12.9927589640401,-1.2792814688989,-3.95912511815523));
#25898=CARTESIAN_POINT('Ctrl Pts',(13.1114771740022,2.62279488400284,-3.22988833933176));
#25899=CARTESIAN_POINT('Ctrl Pts',(13.2301953839642,4.1374061319782,0.439435567280381));
#25900=CARTESIAN_POINT('Ctrl Pts',(13.3489135939262,1.88583863921803,3.70875271783386));
#25901=CARTESIAN_POINT('Ctrl Pts',(13.4676318038883,-2.08236047650701,3.60208297288041));
#25902=CARTESIAN_POINT('Ctrl Pts',(13.5863500138503,-4.15503956461956,0.216528285738942));
#25903=CARTESIAN_POINT('Ctrl Pts',(13.7050682238123,-2.44548671339688,-3.36613063539831));
#25904=CARTESIAN_POINT('Ctrl Pts',(13.8237864337744,1.49012789947011,-3.88467673536986));
#25905=CARTESIAN_POINT('Ctrl Pts',(13.9425046437364,4.06932409197459,-0.867111819500367));
#25906=CARTESIAN_POINT('Ctrl Pts',(14.0612228536985,2.9442998048962,2.93979030855331));
#25907=CARTESIAN_POINT('Ctrl Pts',(14.1799410636605,-0.860818327845137,
4.07062313879903));
#25908=CARTESIAN_POINT('Ctrl Pts',(14.2986592736225,-3.88241075856883,1.49616531773476));
#25909=CARTESIAN_POINT('Ctrl Pts',(14.4173774835846,-3.36983440985343,-2.44039896264189));
#25910=CARTESIAN_POINT('Ctrl Pts',(14.5360956935466,0.210016568782032,-4.155178159011));
#25911=CARTESIAN_POINT('Ctrl Pts',(14.6548139035087,3.59907929859906,-2.08826776438434));
#25912=CARTESIAN_POINT('Ctrl Pts',(14.7735321134707,3.7112574766783,1.88080884739934));
#25913=CARTESIAN_POINT('Ctrl Pts',(14.8922503234327,0.446563584695773,4.13541474942909));
#25914=CARTESIAN_POINT('Ctrl Pts',(15.0109685333948,-3.22729563843389,2.6303031773798));
#25915=CARTESIAN_POINT('Ctrl Pts',(15.1296867433568,-3.95818728136483,-1.27839009166015));
#25916=CARTESIAN_POINT('Ctrl Pts',(15.2088322166648,-2.05105123342669,-3.09430288357736));
#25917=CARTESIAN_POINT('Ctrl Pts',(15.2484049533188,-0.923694772147997,
-3.40052966909663));
#25918=CARTESIAN_POINT('Ctrl Pts',(15.,-1.03647793659398,-3.81573446232228));
#25919=CARTESIAN_POINT('Ctrl Pts',(14.960427263346,-2.30148466178617,-3.47211737542815));
#25920=CARTESIAN_POINT('Ctrl Pts',(14.920854526692,-3.37148337530834,-2.45329947131456));
#25921=CARTESIAN_POINT('Ctrl Pts',(14.881281790038,-3.76979380899274,-1.21289970995026));
#25922=CARTESIAN_POINT('Ctrl Pts',(14.8689078082356,-3.89434132515796,-0.825039648387669));
#25923=CARTESIAN_POINT('Ctrl Pts',(14.8565338264332,-3.95321467832305,-0.415514473039758));
#25924=CARTESIAN_POINT('Ctrl Pts',(14.8441598446308,-3.95012252210193,-0.00484157028959653));
#25925=CARTESIAN_POINT('Origin',(15.4,4.91674827952517,-1.16214730382437));
#25926=CARTESIAN_POINT('',(20.4,4.68474025750198,-1.25527236874723));
#25927=CARTESIAN_POINT('',(20.4,4.91674827952517,-1.16214730382437));
#25928=CARTESIAN_POINT('',(15.4,4.68474025750198,-1.25527236874723));
#25929=CARTESIAN_POINT('',(15.4,4.68474025750198,-1.25527236874723));
#25930=CARTESIAN_POINT('',(15.4,4.91674827952517,-1.16214730382437));
#25931=CARTESIAN_POINT('Origin',(15.4,4.78133284013089,-1.28115427325748));
#25932=CARTESIAN_POINT('',(15.4,4.68474025750198,-1.25527236874723));
#25933=CARTESIAN_POINT('Origin',(15.4,4.68474025750198,-1.25527236874723));
#25934=CARTESIAN_POINT('',(20.4,4.68474025750198,-1.25527236874723));
#25935=CARTESIAN_POINT('Origin',(20.4,4.78133284013089,-1.28115427325748));
#25936=CARTESIAN_POINT('Origin',(15.4,4.44842828911141,-2.39509618943234));
#25937=CARTESIAN_POINT('',(20.4,4.20022320835453,-2.425));
#25938=CARTESIAN_POINT('',(20.4,4.44842828911141,-2.39509618943234));
#25939=CARTESIAN_POINT('',(15.4,4.20022320835453,-2.425));
#25940=CARTESIAN_POINT('',(15.4,4.20022320835453,-2.425));
#25941=CARTESIAN_POINT('',(15.4,4.44842828911141,-2.39509618943234));
#25942=CARTESIAN_POINT('Origin',(15.4,4.28682574873297,-2.475));
#25943=CARTESIAN_POINT('',(15.4,4.20022320835453,-2.425));
#25944=CARTESIAN_POINT('Origin',(15.4,4.20022320835453,-2.425));
#25945=CARTESIAN_POINT('',(20.4,4.20022320835453,-2.425));
#25946=CARTESIAN_POINT('Origin',(20.4,4.28682574873297,-2.475));
#25947=CARTESIAN_POINT('Origin',(15.4,3.67695526217005,-3.46482322781408));
#25948=CARTESIAN_POINT('',(20.4,3.42946788875475,-3.42946788875476));
#25949=CARTESIAN_POINT('',(20.4,3.67695526217005,-3.46482322781408));
#25950=CARTESIAN_POINT('',(15.4,3.42946788875475,-3.42946788875476));
#25951=CARTESIAN_POINT('',(15.4,3.42946788875475,-3.42946788875476));
#25952=CARTESIAN_POINT('',(15.4,3.67695526217005,-3.46482322781408));
#25953=CARTESIAN_POINT('Origin',(15.4,3.50017856687341,-3.50017856687341));
#25954=CARTESIAN_POINT('',(15.4,3.42946788875475,-3.42946788875476));
#25955=CARTESIAN_POINT('Origin',(15.4,3.42946788875475,-3.42946788875476));
#25956=CARTESIAN_POINT('',(20.4,3.42946788875475,-3.42946788875476));
#25957=CARTESIAN_POINT('Origin',(20.4,3.50017856687341,-3.50017856687341));
#25958=CARTESIAN_POINT('Origin',(15.4,2.65490381056766,-4.29842828911142));
#25959=CARTESIAN_POINT('',(20.4,2.425,-4.20022320835453));
#25960=CARTESIAN_POINT('',(20.4,2.65490381056766,-4.29842828911142));
#25961=CARTESIAN_POINT('',(15.4,2.425,-4.20022320835453));
#25962=CARTESIAN_POINT('',(15.4,2.425,-4.20022320835453));
#25963=CARTESIAN_POINT('',(15.4,2.65490381056766,-4.29842828911142));
#25964=CARTESIAN_POINT('Origin',(15.4,2.475,-4.28682574873297));
#25965=CARTESIAN_POINT('',(15.4,2.425,-4.20022320835453));
#25966=CARTESIAN_POINT('Origin',(15.4,2.425,-4.20022320835453));
#25967=CARTESIAN_POINT('',(20.4,2.425,-4.20022320835453));
#25968=CARTESIAN_POINT('Origin',(20.4,2.475,-4.28682574873297));
#25969=CARTESIAN_POINT('Origin',(15.4,1.45192505171109,-4.83910256599442));
#25970=CARTESIAN_POINT('',(20.4,1.25527236874722,-4.68474025750198));
#25971=CARTESIAN_POINT('',(20.4,1.45192505171109,-4.83910256599442));
#25972=CARTESIAN_POINT('',(15.4,1.25527236874722,-4.68474025750198));
#25973=CARTESIAN_POINT('',(15.4,1.25527236874722,-4.68474025750198));
#25974=CARTESIAN_POINT('',(15.4,1.45192505171109,-4.83910256599442));
#25975=CARTESIAN_POINT('Origin',(15.4,1.28115427325748,-4.78133284013089));
#25976=CARTESIAN_POINT('',(15.4,1.25527236874722,-4.68474025750198));
#25977=CARTESIAN_POINT('Origin',(15.4,1.25527236874722,-4.68474025750198));
#25978=CARTESIAN_POINT('',(20.4,1.25527236874722,-4.68474025750198));
#25979=CARTESIAN_POINT('Origin',(20.4,1.28115427325748,-4.78133284013089));
#25980=CARTESIAN_POINT('Origin',(15.4,0.149999999999999,-5.05));
#25981=CARTESIAN_POINT('',(20.4,-8.90930546379699E-16,-4.85));
#25982=CARTESIAN_POINT('',(20.4,0.149999999999999,-5.05));
#25983=CARTESIAN_POINT('',(15.4,-8.90930546379699E-16,-4.85));
#25984=CARTESIAN_POINT('',(15.4,-8.90930546379699E-16,-4.85));
#25985=CARTESIAN_POINT('',(15.4,0.149999999999999,-5.05));
#25986=CARTESIAN_POINT('Origin',(15.4,-9.0930024836691E-16,-4.95));
#25987=CARTESIAN_POINT('',(15.4,-8.90930546379699E-16,-4.85));
#25988=CARTESIAN_POINT('Origin',(15.4,-8.90930546379699E-16,-4.85));
#25989=CARTESIAN_POINT('',(20.4,-8.90930546379699E-16,-4.85));
#25990=CARTESIAN_POINT('Origin',(20.4,-9.0930024836691E-16,-4.95));
#25991=CARTESIAN_POINT('Origin',(15.4,-1.16214730382437,-4.91674827952517));
#25992=CARTESIAN_POINT('',(20.4,-1.25527236874723,-4.68474025750198));
#25993=CARTESIAN_POINT('',(20.4,-1.16214730382437,-4.91674827952517));
#25994=CARTESIAN_POINT('',(15.4,-1.25527236874723,-4.68474025750198));
#25995=CARTESIAN_POINT('',(15.4,-1.25527236874723,-4.68474025750198));
#25996=CARTESIAN_POINT('',(15.4,-1.16214730382437,-4.91674827952517));
#25997=CARTESIAN_POINT('Origin',(15.4,-1.28115427325748,-4.78133284013089));
#25998=CARTESIAN_POINT('',(15.4,-1.25527236874723,-4.68474025750198));
#25999=CARTESIAN_POINT('Origin',(15.4,-1.25527236874723,-4.68474025750198));
#26000=CARTESIAN_POINT('',(20.4,-1.25527236874723,-4.68474025750198));
#26001=CARTESIAN_POINT('Origin',(20.4,-1.28115427325748,-4.78133284013089));
#26002=CARTESIAN_POINT('Origin',(15.4,-2.39509618943234,-4.44842828911141));
#26003=CARTESIAN_POINT('',(20.4,-2.425,-4.20022320835453));
#26004=CARTESIAN_POINT('',(20.4,-2.39509618943234,-4.44842828911141));
#26005=CARTESIAN_POINT('',(15.4,-2.425,-4.20022320835453));
#26006=CARTESIAN_POINT('',(15.4,-2.425,-4.20022320835453));
#26007=CARTESIAN_POINT('',(15.4,-2.39509618943234,-4.44842828911141));
#26008=CARTESIAN_POINT('Origin',(15.4,-2.475,-4.28682574873297));
#26009=CARTESIAN_POINT('',(15.4,-2.425,-4.20022320835453));
#26010=CARTESIAN_POINT('Origin',(15.4,-2.425,-4.20022320835453));
#26011=CARTESIAN_POINT('',(20.4,-2.425,-4.20022320835453));
#26012=CARTESIAN_POINT('Origin',(20.4,-2.475,-4.28682574873297));
#26013=CARTESIAN_POINT('Origin',(15.4,-3.46482322781408,-3.67695526217005));
#26014=CARTESIAN_POINT('',(20.4,-3.42946788875476,-3.42946788875475));
#26015=CARTESIAN_POINT('',(20.4,-3.46482322781408,-3.67695526217005));
#26016=CARTESIAN_POINT('',(15.4,-3.42946788875476,-3.42946788875475));
#26017=CARTESIAN_POINT('',(15.4,-3.42946788875476,-3.42946788875475));
#26018=CARTESIAN_POINT('',(15.4,-3.46482322781408,-3.67695526217005));
#26019=CARTESIAN_POINT('Origin',(15.4,-3.50017856687341,-3.50017856687341));
#26020=CARTESIAN_POINT('',(15.4,-3.42946788875476,-3.42946788875475));
#26021=CARTESIAN_POINT('Origin',(15.4,-3.42946788875476,-3.42946788875475));
#26022=CARTESIAN_POINT('',(20.4,-3.42946788875476,-3.42946788875475));
#26023=CARTESIAN_POINT('Origin',(20.4,-3.50017856687341,-3.50017856687341));
#26024=CARTESIAN_POINT('Origin',(15.4,-4.29842828911142,-2.65490381056766));
#26025=CARTESIAN_POINT('',(20.4,-4.20022320835453,-2.425));
#26026=CARTESIAN_POINT('',(20.4,-4.29842828911142,-2.65490381056766));
#26027=CARTESIAN_POINT('',(15.4,-4.20022320835453,-2.425));
#26028=CARTESIAN_POINT('',(15.4,-4.20022320835453,-2.425));
#26029=CARTESIAN_POINT('',(15.4,-4.29842828911142,-2.65490381056766));
#26030=CARTESIAN_POINT('Origin',(15.4,-4.28682574873297,-2.475));
#26031=CARTESIAN_POINT('',(15.4,-4.20022320835453,-2.425));
#26032=CARTESIAN_POINT('Origin',(15.4,-4.20022320835453,-2.425));
#26033=CARTESIAN_POINT('',(20.4,-4.20022320835453,-2.425));
#26034=CARTESIAN_POINT('Origin',(20.4,-4.28682574873297,-2.475));
#26035=CARTESIAN_POINT('Origin',(15.4,-4.83910256599442,-1.45192505171109));
#26036=CARTESIAN_POINT('',(20.4,-4.68474025750198,-1.25527236874722));
#26037=CARTESIAN_POINT('',(20.4,-4.83910256599442,-1.45192505171109));
#26038=CARTESIAN_POINT('',(15.4,-4.68474025750198,-1.25527236874722));
#26039=CARTESIAN_POINT('',(15.4,-4.68474025750198,-1.25527236874722));
#26040=CARTESIAN_POINT('',(15.4,-4.83910256599442,-1.45192505171109));
#26041=CARTESIAN_POINT('Origin',(15.4,-4.78133284013089,-1.28115427325748));
#26042=CARTESIAN_POINT('',(15.4,-4.68474025750198,-1.25527236874722));
#26043=CARTESIAN_POINT('Origin',(15.4,-4.68474025750198,-1.25527236874722));
#26044=CARTESIAN_POINT('',(20.4,-4.68474025750198,-1.25527236874722));
#26045=CARTESIAN_POINT('Origin',(20.4,-4.78133284013089,-1.28115427325748));
#26046=CARTESIAN_POINT('Origin',(15.4,-5.05,-0.149999999999999));
#26047=CARTESIAN_POINT('',(20.4,-4.85,5.93953697586466E-16));
#26048=CARTESIAN_POINT('',(20.4,-5.05,-0.149999999999999));
#26049=CARTESIAN_POINT('',(15.4,-4.85,5.93953697586466E-16));
#26050=CARTESIAN_POINT('',(15.4,-4.85,5.93953697586466E-16));
#26051=CARTESIAN_POINT('',(15.4,-5.05,-0.149999999999999));
#26052=CARTESIAN_POINT('Origin',(15.4,-4.95,6.0620016557794E-16));
#26053=CARTESIAN_POINT('',(15.4,-4.85,5.93953697586466E-16));
#26054=CARTESIAN_POINT('Origin',(15.4,-4.85,5.93953697586466E-16));
#26055=CARTESIAN_POINT('',(20.4,-4.85,5.93953697586466E-16));
#26056=CARTESIAN_POINT('Origin',(20.4,-4.95,6.0620016557794E-16));
#26057=CARTESIAN_POINT('Origin',(15.4,-4.91674827952517,1.16214730382437));
#26058=CARTESIAN_POINT('',(20.4,-4.68474025750198,1.25527236874723));
#26059=CARTESIAN_POINT('',(20.4,-4.91674827952517,1.16214730382437));
#26060=CARTESIAN_POINT('',(15.4,-4.68474025750198,1.25527236874723));
#26061=CARTESIAN_POINT('',(15.4,-4.68474025750198,1.25527236874723));
#26062=CARTESIAN_POINT('',(15.4,-4.91674827952517,1.16214730382437));
#26063=CARTESIAN_POINT('Origin',(15.4,-4.78133284013089,1.28115427325748));
#26064=CARTESIAN_POINT('',(15.4,-4.68474025750198,1.25527236874723));
#26065=CARTESIAN_POINT('Origin',(15.4,-4.68474025750198,1.25527236874723));
#26066=CARTESIAN_POINT('',(20.4,-4.68474025750198,1.25527236874723));
#26067=CARTESIAN_POINT('Origin',(20.4,-4.78133284013089,1.28115427325748));
#26068=CARTESIAN_POINT('Origin',(15.4,-4.44842828911141,2.39509618943234));
#26069=CARTESIAN_POINT('',(20.4,-4.20022320835453,2.425));
#26070=CARTESIAN_POINT('',(20.4,-4.44842828911141,2.39509618943234));
#26071=CARTESIAN_POINT('',(15.4,-4.20022320835453,2.425));
#26072=CARTESIAN_POINT('',(15.4,-4.20022320835453,2.425));
#26073=CARTESIAN_POINT('',(15.4,-4.44842828911141,2.39509618943234));
#26074=CARTESIAN_POINT('Origin',(15.4,-4.28682574873297,2.475));
#26075=CARTESIAN_POINT('',(15.4,-4.20022320835453,2.425));
#26076=CARTESIAN_POINT('Origin',(15.4,-4.20022320835453,2.425));
#26077=CARTESIAN_POINT('',(20.4,-4.20022320835453,2.425));
#26078=CARTESIAN_POINT('Origin',(20.4,-4.28682574873297,2.475));
#26079=CARTESIAN_POINT('Origin',(15.4,-3.67695526217005,3.46482322781408));
#26080=CARTESIAN_POINT('',(20.4,-3.42946788875476,3.42946788875476));
#26081=CARTESIAN_POINT('',(20.4,-3.67695526217005,3.46482322781408));
#26082=CARTESIAN_POINT('',(15.4,-3.42946788875476,3.42946788875476));
#26083=CARTESIAN_POINT('',(15.4,-3.42946788875476,3.42946788875476));
#26084=CARTESIAN_POINT('',(15.4,-3.67695526217005,3.46482322781408));
#26085=CARTESIAN_POINT('Origin',(15.4,-3.50017856687341,3.50017856687341));
#26086=CARTESIAN_POINT('',(15.4,-3.42946788875476,3.42946788875476));
#26087=CARTESIAN_POINT('Origin',(15.4,-3.42946788875476,3.42946788875476));
#26088=CARTESIAN_POINT('',(20.4,-3.42946788875476,3.42946788875476));
#26089=CARTESIAN_POINT('Origin',(20.4,-3.50017856687341,3.50017856687341));
#26090=CARTESIAN_POINT('Origin',(15.4,-2.65490381056766,4.29842828911142));
#26091=CARTESIAN_POINT('',(20.4,-2.425,4.20022320835453));
#26092=CARTESIAN_POINT('',(20.4,-2.65490381056766,4.29842828911142));
#26093=CARTESIAN_POINT('',(15.4,-2.425,4.20022320835453));
#26094=CARTESIAN_POINT('',(15.4,-2.425,4.20022320835453));
#26095=CARTESIAN_POINT('',(15.4,-2.65490381056766,4.29842828911142));
#26096=CARTESIAN_POINT('Origin',(15.4,-2.475,4.28682574873297));
#26097=CARTESIAN_POINT('',(15.4,-2.425,4.20022320835453));
#26098=CARTESIAN_POINT('Origin',(15.4,-2.425,4.20022320835453));
#26099=CARTESIAN_POINT('',(20.4,-2.425,4.20022320835453));
#26100=CARTESIAN_POINT('Origin',(20.4,-2.475,4.28682574873297));
#26101=CARTESIAN_POINT('Origin',(15.4,-1.45192505171109,4.83910256599442));
#26102=CARTESIAN_POINT('',(20.4,-1.25527236874722,4.68474025750198));
#26103=CARTESIAN_POINT('',(20.4,-1.45192505171109,4.83910256599442));
#26104=CARTESIAN_POINT('',(15.4,-1.25527236874722,4.68474025750198));
#26105=CARTESIAN_POINT('',(15.4,-1.25527236874722,4.68474025750198));
#26106=CARTESIAN_POINT('',(15.4,-1.45192505171109,4.83910256599442));
#26107=CARTESIAN_POINT('Origin',(15.4,-1.28115427325748,4.78133284013089));
#26108=CARTESIAN_POINT('',(15.4,-1.25527236874722,4.68474025750198));
#26109=CARTESIAN_POINT('Origin',(15.4,-1.25527236874722,4.68474025750198));
#26110=CARTESIAN_POINT('',(20.4,-1.25527236874722,4.68474025750198));
#26111=CARTESIAN_POINT('Origin',(20.4,-1.28115427325748,4.78133284013089));
#26112=CARTESIAN_POINT('Origin',(15.4,-0.15,5.05));
#26113=CARTESIAN_POINT('',(20.4,2.96976848793233E-16,4.85));
#26114=CARTESIAN_POINT('',(20.4,-0.15,5.05));
#26115=CARTESIAN_POINT('',(15.4,2.96976848793233E-16,4.85));
#26116=CARTESIAN_POINT('',(15.4,2.96976848793233E-16,4.85));
#26117=CARTESIAN_POINT('',(15.4,-0.15,5.05));
#26118=CARTESIAN_POINT('Origin',(15.4,3.0310008278897E-16,4.95));
#26119=CARTESIAN_POINT('',(15.4,2.96976848793233E-16,4.85));
#26120=CARTESIAN_POINT('Origin',(15.4,2.96976848793233E-16,4.85));
#26121=CARTESIAN_POINT('',(20.4,2.96976848793233E-16,4.85));
#26122=CARTESIAN_POINT('Origin',(20.4,3.0310008278897E-16,4.95));
#26123=CARTESIAN_POINT('Origin',(15.4,1.16214730382437,4.91674827952517));
#26124=CARTESIAN_POINT('',(20.4,1.25527236874723,4.68474025750198));
#26125=CARTESIAN_POINT('',(20.4,1.16214730382437,4.91674827952517));
#26126=CARTESIAN_POINT('',(15.4,1.25527236874723,4.68474025750198));
#26127=CARTESIAN_POINT('',(15.4,1.25527236874723,4.68474025750198));
#26128=CARTESIAN_POINT('',(15.4,1.16214730382437,4.91674827952517));
#26129=CARTESIAN_POINT('Origin',(15.4,1.28115427325748,4.78133284013089));
#26130=CARTESIAN_POINT('',(15.4,1.25527236874723,4.68474025750198));
#26131=CARTESIAN_POINT('Origin',(15.4,1.25527236874723,4.68474025750198));
#26132=CARTESIAN_POINT('',(20.4,1.25527236874723,4.68474025750198));
#26133=CARTESIAN_POINT('Origin',(20.4,1.28115427325748,4.78133284013089));
#26134=CARTESIAN_POINT('Origin',(15.4,2.39509618943233,4.44842828911142));
#26135=CARTESIAN_POINT('',(20.4,2.425,4.20022320835453));
#26136=CARTESIAN_POINT('',(20.4,2.39509618943233,4.44842828911142));
#26137=CARTESIAN_POINT('',(15.4,2.425,4.20022320835453));
#26138=CARTESIAN_POINT('',(15.4,2.425,4.20022320835453));
#26139=CARTESIAN_POINT('',(15.4,2.39509618943233,4.44842828911142));
#26140=CARTESIAN_POINT('Origin',(15.4,2.475,4.28682574873297));
#26141=CARTESIAN_POINT('',(15.4,2.425,4.20022320835453));
#26142=CARTESIAN_POINT('Origin',(15.4,2.425,4.20022320835453));
#26143=CARTESIAN_POINT('',(20.4,2.425,4.20022320835453));
#26144=CARTESIAN_POINT('Origin',(20.4,2.475,4.28682574873297));
#26145=CARTESIAN_POINT('Origin',(15.4,3.46482322781408,3.67695526217005));
#26146=CARTESIAN_POINT('',(20.4,3.42946788875476,3.42946788875476));
#26147=CARTESIAN_POINT('',(20.4,3.46482322781408,3.67695526217005));
#26148=CARTESIAN_POINT('',(15.4,3.42946788875476,3.42946788875476));
#26149=CARTESIAN_POINT('',(15.4,3.42946788875476,3.42946788875476));
#26150=CARTESIAN_POINT('',(15.4,3.46482322781408,3.67695526217005));
#26151=CARTESIAN_POINT('Origin',(15.4,3.50017856687341,3.50017856687341));
#26152=CARTESIAN_POINT('',(15.4,3.42946788875476,3.42946788875476));
#26153=CARTESIAN_POINT('Origin',(15.4,3.42946788875476,3.42946788875476));
#26154=CARTESIAN_POINT('',(20.4,3.42946788875476,3.42946788875476));
#26155=CARTESIAN_POINT('Origin',(20.4,3.50017856687341,3.50017856687341));
#26156=CARTESIAN_POINT('Origin',(15.4,4.29842828911142,2.65490381056767));
#26157=CARTESIAN_POINT('',(20.4,4.20022320835453,2.425));
#26158=CARTESIAN_POINT('',(20.4,4.29842828911142,2.65490381056767));
#26159=CARTESIAN_POINT('',(15.4,4.20022320835453,2.425));
#26160=CARTESIAN_POINT('',(15.4,4.20022320835453,2.425));
#26161=CARTESIAN_POINT('',(15.4,4.29842828911142,2.65490381056767));
#26162=CARTESIAN_POINT('Origin',(15.4,4.28682574873297,2.475));
#26163=CARTESIAN_POINT('',(15.4,4.20022320835453,2.425));
#26164=CARTESIAN_POINT('Origin',(15.4,4.20022320835453,2.425));
#26165=CARTESIAN_POINT('',(20.4,4.20022320835453,2.425));
#26166=CARTESIAN_POINT('Origin',(20.4,4.28682574873297,2.475));
#26167=CARTESIAN_POINT('Origin',(15.4,4.83910256599442,1.45192505171109));
#26168=CARTESIAN_POINT('',(20.4,4.68474025750198,1.25527236874723));
#26169=CARTESIAN_POINT('',(20.4,4.83910256599442,1.45192505171109));
#26170=CARTESIAN_POINT('',(15.4,4.68474025750198,1.25527236874723));
#26171=CARTESIAN_POINT('',(15.4,4.68474025750198,1.25527236874723));
#26172=CARTESIAN_POINT('',(15.4,4.83910256599442,1.45192505171109));
#26173=CARTESIAN_POINT('Origin',(15.4,4.78133284013089,1.28115427325748));
#26174=CARTESIAN_POINT('',(15.4,4.68474025750198,1.25527236874723));
#26175=CARTESIAN_POINT('Origin',(15.4,4.68474025750198,1.25527236874723));
#26176=CARTESIAN_POINT('',(20.4,4.68474025750198,1.25527236874723));
#26177=CARTESIAN_POINT('Origin',(20.4,4.78133284013089,1.28115427325748));
#26178=CARTESIAN_POINT('Origin',(15.4,5.05,0.15));
#26179=CARTESIAN_POINT('',(20.4,4.85,0.));
#26180=CARTESIAN_POINT('',(20.4,5.05,0.15));
#26181=CARTESIAN_POINT('',(15.4,4.85,0.));
#26182=CARTESIAN_POINT('',(15.4,4.85,0.));
#26183=CARTESIAN_POINT('',(15.4,5.05,0.15));
#26184=CARTESIAN_POINT('Origin',(15.4,4.95,0.));
#26185=CARTESIAN_POINT('',(15.4,4.85,0.));
#26186=CARTESIAN_POINT('Origin',(15.4,4.85,0.));
#26187=CARTESIAN_POINT('',(20.4,4.85,0.));
#26188=CARTESIAN_POINT('Origin',(20.4,4.95,0.));
#26189=CARTESIAN_POINT('Origin',(-6.,3.6,0.));
#26190=CARTESIAN_POINT('',(-6.,-3.6,-4.40872847693047E-16));
#26191=CARTESIAN_POINT('Origin',(-6.,0.,0.));
#26192=CARTESIAN_POINT('Origin',(-5.8,0.,0.));
#26193=CARTESIAN_POINT('',(-5.8,-3.8,-4.65365783675994E-16));
#26194=CARTESIAN_POINT('Origin',(4.7,0.,0.));
#26195=CARTESIAN_POINT('Origin',(20.75,0.,0.));
#26196=CARTESIAN_POINT('',(21.,-4.5,-5.51091059616309E-16));
#26197=CARTESIAN_POINT('Origin',(21.,0.,0.));
#26198=CARTESIAN_POINT('',(20.75,-4.75,-5.81707229594993E-16));
#26199=CARTESIAN_POINT('Origin',(21.,3.,0.));
#26200=CARTESIAN_POINT('',(21.,-3.,-3.67394039744206E-16));
#26201=CARTESIAN_POINT('Origin',(21.,0.,0.));
#26202=CARTESIAN_POINT('Origin',(20.65,0.,0.));
#26203=CARTESIAN_POINT('',(20.3,-3.,-3.67394039744206E-16));
#26204=CARTESIAN_POINT('',(20.65,-3.,-3.67394039744206E-16));
#26205=CARTESIAN_POINT('Origin',(20.3,0.,0.));
#26206=CARTESIAN_POINT('Origin',(20.3,0.,0.));
#37159=UNCERTAINTY_MEASURE_WITH_UNIT(LENGTH_MEASURE(0.01),#37182,
'DISTANCE_ACCURACY_VALUE',
'Maximum model space distance between geometric entities at asserted c
onnectivities');
#37166=UNCERTAINTY_MEASURE_WITH_UNIT(LENGTH_MEASURE(0.01),#37182,
'DISTANCE_ACCURACY_VALUE',
'Maximum model space distance between geometric entities at asserted c
onnectivities');
#37174=(
GEOMETRIC_REPRESENTATION_CONTEXT(3)
GLOBAL_UNCERTAINTY_ASSIGNED_CONTEXT((#37159))
GLOBAL_UNIT_ASSIGNED_CONTEXT((#37182,#37184,#37185))
REPRESENTATION_CONTEXT('','3D')
);
#37181=(
GEOMETRIC_REPRESENTATION_CONTEXT(3)
GLOBAL_UNCERTAINTY_ASSIGNED_CONTEXT((#37166))
GLOBAL_UNIT_ASSIGNED_CONTEXT((#37182,#37184,#37185))
REPRESENTATION_CONTEXT('','3D')
);
#37182=(
LENGTH_UNIT()
NAMED_UNIT(*)
SI_UNIT(.MILLI.,.METRE.)
);
#37184=(
NAMED_UNIT(*)
PLANE_ANGLE_UNIT()
SI_UNIT($,.RADIAN.)
);
#37185=(
NAMED_UNIT(*)
SI_UNIT($,.STERADIAN.)
SOLID_ANGLE_UNIT()
);
#37193=SHAPE_DEFINITION_REPRESENTATION(#37207,#37244);
#37207=PRODUCT_DEFINITION_SHAPE('',$,#37259);
#37244=SHAPE_REPRESENTATION('',(#15455),#37174);
#37251=PRODUCT_DEFINITION_CONTEXT('part definition',#37295,'design');
#37259=PRODUCT_DEFINITION('2026-10-20-13-23-56-870','07_M8_Camera_Lens',
#37273,#37251);
#37273=PRODUCT_DEFINITION_FORMATION('',$,#37304);
#37295=APPLICATION_CONTEXT(
'Core Data for Automotive Mechanical Design Process');
#37296=PRODUCT_CONTEXT('part definition',#37295,'mechanical');
#37304=PRODUCT('2026-10-20-13-23-56-870','07_M8_Camera_Lens',$,(#37296));
#37381=COLOUR_RGB('Off White',0.89,0.88,0.83);
#37382=FILL_AREA_STYLE_COLOUR('',#37381);
#37383=FILL_AREA_STYLE('',(#37382));
#37384=SURFACE_STYLE_FILL_AREA(#37383);
#37385=SURFACE_SIDE_STYLE('',(#37384));
#37386=SURFACE_STYLE_USAGE(.BOTH.,#37385);
#37387=PRESENTATION_STYLE_ASSIGNMENT((#37386));
ENDSEC;
END-ISO-10303-21;
